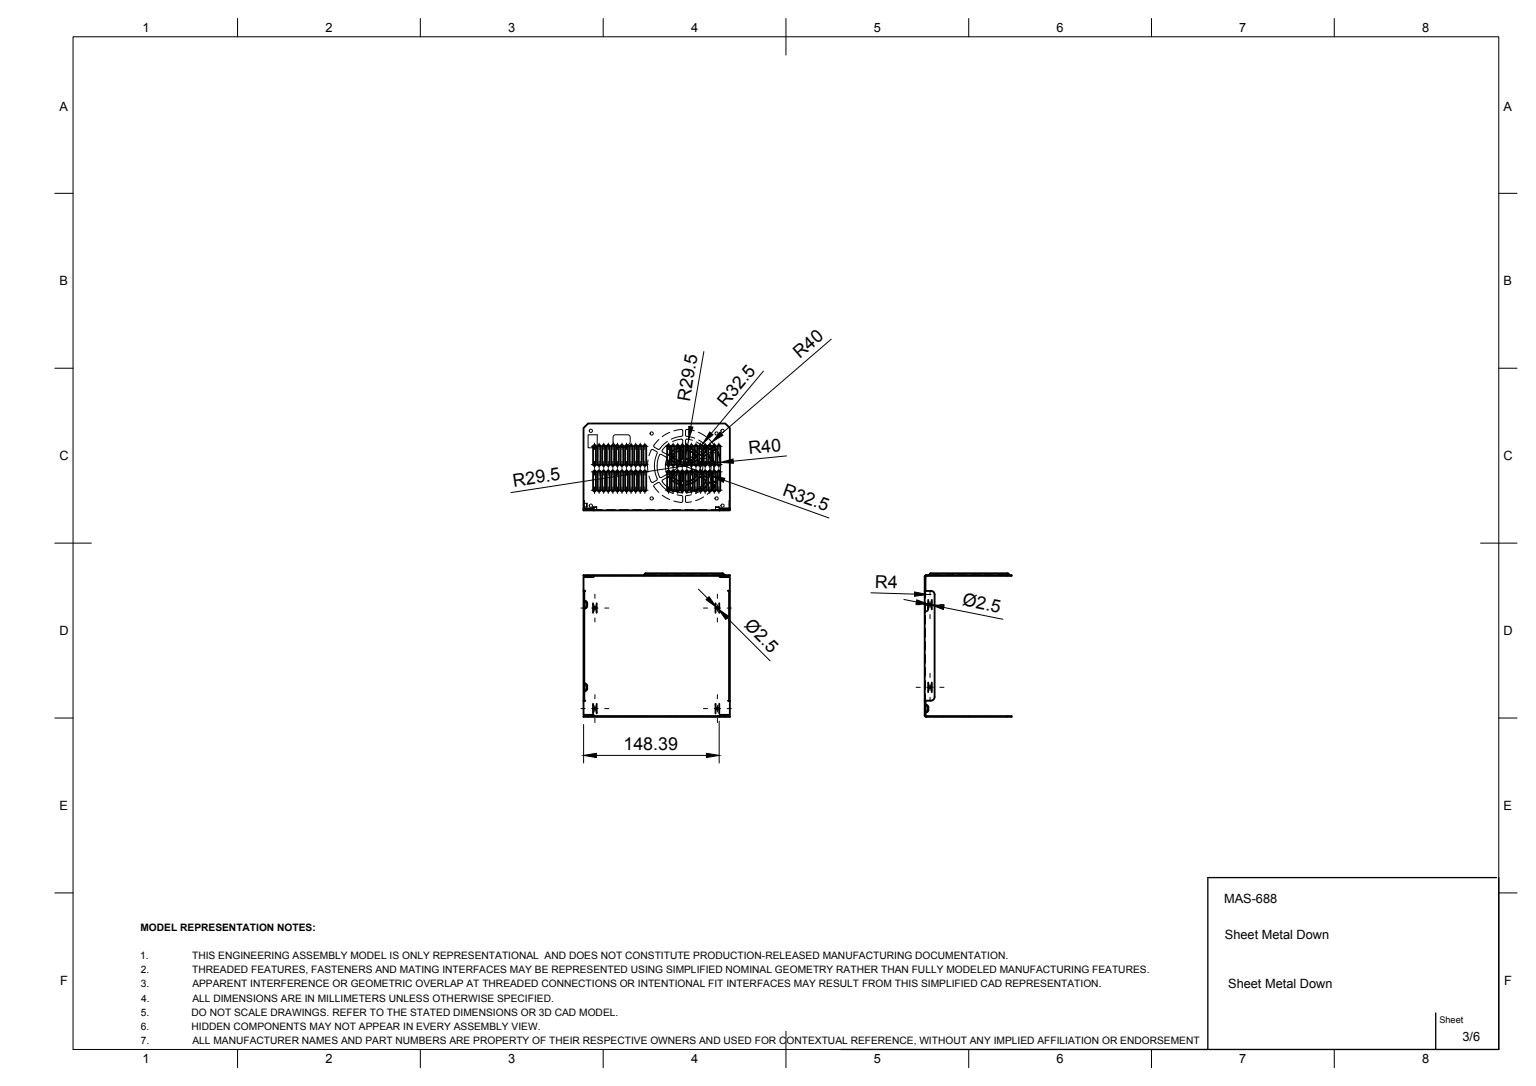
ISO-10303-21;
HEADER;
/* Generated by software containing ST-Developer
 * from STEP Tools, Inc. (www.steptools.com) 
 */

FILE_DESCRIPTION(
/* description */ ('STEP AP214'),
/* implementation_level */ '2;1');

FILE_NAME(
/* name */ 'Sheet Metal Down.step',
/* time_stamp */ '2026-11-14T03:58:36-08:00',
/* author */ (''),
/* organization */ (''),
/* preprocessor_version */ 'ST-DEVELOPER v20.2',
/* originating_system */ 'Autodesk Translation Framework v15.17.0.0',
/* authorisation */ '');

FILE_SCHEMA (('AUTOMOTIVE_DESIGN { 1 0 10303 214 3 1 1 }'));
ENDSEC;

DATA;
#10=MECHANICAL_DESIGN_GEOMETRIC_PRESENTATION_REPRESENTATION('',(#41),#65304);
#33=SHAPE_REPRESENTATION_RELATIONSHIP('SRR','None',#65324,#37);
#37=ADVANCED_BREP_SHAPE_REPRESENTATION('',(#45),#65300);
#41=STYLED_ITEM('',(#65353),#45);
#45=MANIFOLD_SOLID_BREP('Body1',#39933);
#48=FACE_BOUND('',#4336,.T.);
#49=FACE_BOUND('',#4337,.T.);
#50=FACE_BOUND('',#4338,.T.);
#51=FACE_BOUND('',#4339,.T.);
#52=FACE_BOUND('',#4341,.T.);
#53=FACE_BOUND('',#4342,.T.);
#54=FACE_BOUND('',#4343,.T.);
#55=FACE_BOUND('',#4344,.T.);
#56=FACE_BOUND('',#4348,.T.);
#57=FACE_BOUND('',#4349,.T.);
#58=FACE_BOUND('',#4351,.T.);
#59=FACE_BOUND('',#4352,.T.);
#60=FACE_BOUND('',#4356,.T.);
#61=FACE_BOUND('',#4357,.T.);
#62=FACE_BOUND('',#4358,.T.);
#63=FACE_BOUND('',#4359,.T.);
#64=FACE_BOUND('',#4360,.T.);
#65=FACE_BOUND('',#4361,.T.);
#66=FACE_BOUND('',#4362,.T.);
#67=FACE_BOUND('',#4363,.T.);
#68=FACE_BOUND('',#4364,.T.);
#69=FACE_BOUND('',#4365,.T.);
#70=FACE_BOUND('',#4366,.T.);
#71=FACE_BOUND('',#4367,.T.);
#72=FACE_BOUND('',#4368,.T.);
#73=FACE_BOUND('',#4369,.T.);
#74=FACE_BOUND('',#4370,.T.);
#75=FACE_BOUND('',#4371,.T.);
#76=FACE_BOUND('',#4372,.T.);
#77=FACE_BOUND('',#4373,.T.);
#78=FACE_BOUND('',#4374,.T.);
#79=FACE_BOUND('',#4375,.T.);
#80=FACE_BOUND('',#4376,.T.);
#81=FACE_BOUND('',#4377,.T.);
#82=FACE_BOUND('',#4378,.T.);
#83=FACE_BOUND('',#4379,.T.);
#84=FACE_BOUND('',#4380,.T.);
#85=FACE_BOUND('',#4381,.T.);
#86=FACE_BOUND('',#4382,.T.);
#87=FACE_BOUND('',#4383,.T.);
#88=FACE_BOUND('',#4384,.T.);
#89=FACE_BOUND('',#4385,.T.);
#90=FACE_BOUND('',#4386,.T.);
#91=FACE_BOUND('',#4387,.T.);
#92=FACE_BOUND('',#4388,.T.);
#93=FACE_BOUND('',#4389,.T.);
#94=FACE_BOUND('',#4390,.T.);
#95=FACE_BOUND('',#4391,.T.);
#96=FACE_BOUND('',#4392,.T.);
#97=FACE_BOUND('',#4393,.T.);
#98=FACE_BOUND('',#4394,.T.);
#99=FACE_BOUND('',#4395,.T.);
#100=FACE_BOUND('',#4396,.T.);
#101=FACE_BOUND('',#4397,.T.);
#102=FACE_BOUND('',#4398,.T.);
#103=FACE_BOUND('',#4399,.T.);
#104=FACE_BOUND('',#4400,.T.);
#105=FACE_BOUND('',#4401,.T.);
#106=FACE_BOUND('',#4402,.T.);
#107=FACE_BOUND('',#4403,.T.);
#108=FACE_BOUND('',#4405,.T.);
#109=FACE_BOUND('',#4406,.T.);
#110=FACE_BOUND('',#4407,.T.);
#111=FACE_BOUND('',#4408,.T.);
#112=FACE_BOUND('',#4409,.T.);
#113=FACE_BOUND('',#4410,.T.);
#114=FACE_BOUND('',#4411,.T.);
#115=FACE_BOUND('',#4412,.T.);
#116=FACE_BOUND('',#4413,.T.);
#117=FACE_BOUND('',#4414,.T.);
#118=FACE_BOUND('',#4415,.T.);
#119=FACE_BOUND('',#4416,.T.);
#120=FACE_BOUND('',#4417,.T.);
#121=FACE_BOUND('',#4418,.T.);
#122=FACE_BOUND('',#4419,.T.);
#123=FACE_BOUND('',#4420,.T.);
#124=FACE_BOUND('',#4421,.T.);
#125=FACE_BOUND('',#4422,.T.);
#126=FACE_BOUND('',#4423,.T.);
#127=FACE_BOUND('',#4424,.T.);
#128=FACE_BOUND('',#4425,.T.);
#129=FACE_BOUND('',#4426,.T.);
#130=FACE_BOUND('',#4427,.T.);
#131=FACE_BOUND('',#4428,.T.);
#132=FACE_BOUND('',#4429,.T.);
#133=FACE_BOUND('',#4430,.T.);
#134=FACE_BOUND('',#4431,.T.);
#135=FACE_BOUND('',#4432,.T.);
#136=FACE_BOUND('',#4433,.T.);
#137=FACE_BOUND('',#4434,.T.);
#138=FACE_BOUND('',#4435,.T.);
#139=FACE_BOUND('',#4436,.T.);
#140=FACE_BOUND('',#4437,.T.);
#141=FACE_BOUND('',#4438,.T.);
#142=FACE_BOUND('',#4439,.T.);
#143=FACE_BOUND('',#4440,.T.);
#144=FACE_BOUND('',#4441,.T.);
#145=FACE_BOUND('',#4442,.T.);
#146=FACE_BOUND('',#4443,.T.);
#147=FACE_BOUND('',#4444,.T.);
#148=FACE_BOUND('',#4445,.T.);
#149=FACE_BOUND('',#4446,.T.);
#150=FACE_BOUND('',#4447,.T.);
#151=FACE_BOUND('',#4448,.T.);
#152=FACE_BOUND('',#4449,.T.);
#153=FACE_BOUND('',#4450,.T.);
#154=FACE_BOUND('',#4451,.T.);
#155=FACE_BOUND('',#4452,.T.);
#156=FACE_BOUND('',#4479,.T.);
#157=FACE_BOUND('',#4480,.T.);
#158=FACE_BOUND('',#4481,.T.);
#159=FACE_BOUND('',#4482,.T.);
#160=FACE_BOUND('',#4483,.T.);
#161=FACE_BOUND('',#4484,.T.);
#162=FACE_BOUND('',#4485,.T.);
#163=FACE_BOUND('',#4486,.T.);
#164=FACE_BOUND('',#4487,.T.);
#165=FACE_BOUND('',#4488,.T.);
#166=FACE_BOUND('',#4489,.T.);
#167=FACE_BOUND('',#4490,.T.);
#168=FACE_BOUND('',#4491,.T.);
#169=FACE_BOUND('',#4492,.T.);
#170=FACE_BOUND('',#4493,.T.);
#171=FACE_BOUND('',#4494,.T.);
#172=FACE_BOUND('',#4495,.T.);
#173=FACE_BOUND('',#4496,.T.);
#174=FACE_BOUND('',#4503,.T.);
#175=FACE_BOUND('',#4504,.T.);
#176=FACE_BOUND('',#4505,.T.);
#177=FACE_BOUND('',#4506,.T.);
#178=FACE_BOUND('',#4507,.T.);
#179=FACE_BOUND('',#4508,.T.);
#180=FACE_BOUND('',#4509,.T.);
#181=FACE_BOUND('',#4510,.T.);
#182=FACE_BOUND('',#4511,.T.);
#183=FACE_BOUND('',#4512,.T.);
#184=FACE_BOUND('',#4513,.T.);
#185=FACE_BOUND('',#4515,.T.);
#186=FACE_BOUND('',#4516,.T.);
#187=FACE_BOUND('',#4517,.T.);
#188=FACE_BOUND('',#4518,.T.);
#189=FACE_BOUND('',#4519,.T.);
#190=FACE_BOUND('',#4520,.T.);
#191=FACE_BOUND('',#4521,.T.);
#192=FACE_BOUND('',#4522,.T.);
#193=FACE_BOUND('',#4523,.T.);
#194=FACE_BOUND('',#4524,.T.);
#195=FACE_BOUND('',#4525,.T.);
#196=FACE_BOUND('',#4567,.T.);
#197=FACE_BOUND('',#4575,.T.);
#198=FACE_BOUND('',#4587,.T.);
#199=FACE_BOUND('',#4595,.T.);
#200=FACE_BOUND('',#4607,.T.);
#201=FACE_BOUND('',#4615,.T.);
#202=FACE_BOUND('',#4627,.T.);
#203=FACE_BOUND('',#4635,.T.);
#204=FACE_BOUND('',#4637,.T.);
#205=FACE_BOUND('',#4638,.T.);
#206=FACE_BOUND('',#4639,.T.);
#207=FACE_BOUND('',#4640,.T.);
#208=FACE_BOUND('',#4641,.T.);
#209=FACE_BOUND('',#4642,.T.);
#210=FACE_BOUND('',#4643,.T.);
#211=FACE_BOUND('',#4644,.T.);
#212=FACE_BOUND('',#4645,.T.);
#213=FACE_BOUND('',#4646,.T.);
#214=FACE_BOUND('',#4647,.T.);
#215=FACE_BOUND('',#4648,.T.);
#216=FACE_BOUND('',#4649,.T.);
#217=FACE_BOUND('',#4650,.T.);
#218=FACE_BOUND('',#4651,.T.);
#219=FACE_BOUND('',#4652,.T.);
#220=FACE_BOUND('',#4653,.T.);
#221=FACE_BOUND('',#4654,.T.);
#222=FACE_BOUND('',#4941,.T.);
#223=FACE_BOUND('',#4949,.T.);
#224=FACE_BOUND('',#4961,.T.);
#225=FACE_BOUND('',#4969,.T.);
#629=PLANE('',#40239);
#630=PLANE('',#40244);
#631=PLANE('',#40249);
#632=PLANE('',#40250);
#633=PLANE('',#40251);
#634=PLANE('',#40254);
#635=PLANE('',#40257);
#636=PLANE('',#40258);
#637=PLANE('',#40259);
#638=PLANE('',#40310);
#639=PLANE('',#40361);
#640=PLANE('',#40362);
#641=PLANE('',#40363);
#642=PLANE('',#40364);
#643=PLANE('',#40365);
#644=PLANE('',#40366);
#645=PLANE('',#40367);
#646=PLANE('',#40368);
#647=PLANE('',#40369);
#648=PLANE('',#40370);
#649=PLANE('',#40371);
#650=PLANE('',#40372);
#651=PLANE('',#40373);
#652=PLANE('',#40374);
#653=PLANE('',#40375);
#654=PLANE('',#40376);
#655=PLANE('',#40377);
#656=PLANE('',#40378);
#657=PLANE('',#40379);
#658=PLANE('',#40380);
#659=PLANE('',#40381);
#660=PLANE('',#40382);
#661=PLANE('',#40383);
#662=PLANE('',#40384);
#663=PLANE('',#40385);
#664=PLANE('',#40440);
#665=PLANE('',#40441);
#666=PLANE('',#40450);
#667=PLANE('',#40460);
#668=PLANE('',#40462);
#669=PLANE('',#40464);
#670=PLANE('',#40466);
#671=PLANE('',#40469);
#672=PLANE('',#40470);
#673=PLANE('',#40471);
#674=PLANE('',#40472);
#675=PLANE('',#40473);
#676=PLANE('',#40478);
#677=PLANE('',#40479);
#678=PLANE('',#40480);
#679=PLANE('',#40481);
#680=PLANE('',#40482);
#681=PLANE('',#40485);
#682=PLANE('',#40488);
#683=PLANE('',#40497);
#684=PLANE('',#40504);
#685=PLANE('',#40513);
#686=PLANE('',#40514);
#687=PLANE('',#40515);
#688=PLANE('',#40520);
#689=PLANE('',#40521);
#690=PLANE('',#40522);
#691=PLANE('',#40523);
#692=PLANE('',#40526);
#693=PLANE('',#40535);
#694=PLANE('',#40542);
#695=PLANE('',#40551);
#696=PLANE('',#40552);
#697=PLANE('',#40553);
#698=PLANE('',#40558);
#699=PLANE('',#40559);
#700=PLANE('',#40560);
#701=PLANE('',#40561);
#702=PLANE('',#40564);
#703=PLANE('',#40573);
#704=PLANE('',#40580);
#705=PLANE('',#40589);
#706=PLANE('',#40590);
#707=PLANE('',#40591);
#708=PLANE('',#40596);
#709=PLANE('',#40597);
#710=PLANE('',#40598);
#711=PLANE('',#40599);
#712=PLANE('',#40602);
#713=PLANE('',#40611);
#714=PLANE('',#40618);
#715=PLANE('',#40627);
#716=PLANE('',#40628);
#717=PLANE('',#40629);
#718=PLANE('',#40634);
#719=PLANE('',#40635);
#720=PLANE('',#40636);
#721=PLANE('',#40637);
#722=PLANE('',#40692);
#723=PLANE('',#40693);
#724=PLANE('',#40694);
#725=PLANE('',#40695);
#726=PLANE('',#40696);
#727=PLANE('',#40697);
#728=PLANE('',#40698);
#729=PLANE('',#40699);
#730=PLANE('',#40700);
#731=PLANE('',#40701);
#732=PLANE('',#40702);
#733=PLANE('',#40758);
#734=PLANE('',#40760);
#735=PLANE('',#40762);
#736=PLANE('',#40764);
#737=PLANE('',#40766);
#738=PLANE('',#40768);
#739=PLANE('',#40769);
#740=PLANE('',#40770);
#741=PLANE('',#40771);
#742=PLANE('',#40772);
#743=PLANE('',#40773);
#744=PLANE('',#40774);
#745=PLANE('',#40775);
#746=PLANE('',#40776);
#747=PLANE('',#40777);
#748=PLANE('',#40779);
#749=PLANE('',#40780);
#750=PLANE('',#40781);
#751=PLANE('',#40783);
#752=PLANE('',#40784);
#753=PLANE('',#40786);
#754=PLANE('',#40788);
#755=PLANE('',#40789);
#756=PLANE('',#40790);
#757=PLANE('',#40792);
#758=PLANE('',#40794);
#759=PLANE('',#40795);
#760=PLANE('',#40797);
#761=PLANE('',#40798);
#762=PLANE('',#40799);
#763=PLANE('',#40801);
#764=PLANE('',#40802);
#765=PLANE('',#40804);
#766=PLANE('',#40805);
#767=PLANE('',#40807);
#768=PLANE('',#40808);
#769=PLANE('',#40810);
#770=PLANE('',#40812);
#771=PLANE('',#40813);
#772=PLANE('',#40815);
#773=PLANE('',#40816);
#774=PLANE('',#40818);
#775=PLANE('',#40819);
#776=PLANE('',#40821);
#777=PLANE('',#40822);
#778=PLANE('',#40824);
#779=PLANE('',#40825);
#780=PLANE('',#40827);
#781=PLANE('',#40828);
#782=PLANE('',#40830);
#783=PLANE('',#40831);
#784=PLANE('',#40832);
#785=PLANE('',#40834);
#786=PLANE('',#40835);
#787=PLANE('',#40837);
#788=PLANE('',#40838);
#789=PLANE('',#40840);
#790=PLANE('',#40841);
#791=PLANE('',#40843);
#792=PLANE('',#40844);
#793=PLANE('',#40846);
#794=PLANE('',#40848);
#795=PLANE('',#40849);
#796=PLANE('',#40851);
#797=PLANE('',#40852);
#798=PLANE('',#40854);
#799=PLANE('',#40855);
#800=PLANE('',#40857);
#801=PLANE('',#40858);
#802=PLANE('',#40860);
#803=PLANE('',#40861);
#804=PLANE('',#40863);
#805=PLANE('',#40864);
#806=PLANE('',#40866);
#807=PLANE('',#40867);
#808=PLANE('',#40869);
#809=PLANE('',#40870);
#810=PLANE('',#40872);
#811=PLANE('',#40873);
#812=PLANE('',#40875);
#813=PLANE('',#40876);
#814=PLANE('',#40878);
#815=PLANE('',#40879);
#816=PLANE('',#40881);
#817=PLANE('',#40882);
#818=PLANE('',#40884);
#819=PLANE('',#40885);
#820=PLANE('',#40887);
#821=PLANE('',#40888);
#822=PLANE('',#40890);
#823=PLANE('',#40891);
#824=PLANE('',#40893);
#825=PLANE('',#40894);
#826=PLANE('',#40896);
#827=PLANE('',#40897);
#828=PLANE('',#40899);
#829=PLANE('',#40900);
#830=PLANE('',#40902);
#831=PLANE('',#40903);
#832=PLANE('',#40905);
#833=PLANE('',#40906);
#834=PLANE('',#40908);
#835=PLANE('',#40909);
#836=PLANE('',#40911);
#837=PLANE('',#40912);
#838=PLANE('',#40914);
#839=PLANE('',#40915);
#840=PLANE('',#40917);
#841=PLANE('',#40918);
#842=PLANE('',#40920);
#843=PLANE('',#40921);
#844=PLANE('',#40922);
#845=PLANE('',#40923);
#846=PLANE('',#40924);
#847=PLANE('',#40925);
#848=PLANE('',#40926);
#849=PLANE('',#40927);
#850=PLANE('',#40930);
#851=PLANE('',#40935);
#852=PLANE('',#40936);
#853=PLANE('',#40938);
#854=PLANE('',#40940);
#855=PLANE('',#40943);
#856=PLANE('',#40952);
#857=PLANE('',#40959);
#858=PLANE('',#40968);
#859=PLANE('',#40969);
#860=PLANE('',#40970);
#861=PLANE('',#40975);
#862=PLANE('',#40976);
#863=PLANE('',#40977);
#864=PLANE('',#40978);
#865=PLANE('',#40981);
#866=PLANE('',#40990);
#867=PLANE('',#40997);
#868=PLANE('',#41006);
#869=PLANE('',#41007);
#870=PLANE('',#41008);
#871=PLANE('',#41013);
#872=PLANE('',#41014);
#873=PLANE('',#41015);
#874=PLANE('',#41016);
#875=PLANE('',#41017);
#876=PLANE('',#41018);
#877=PLANE('',#41019);
#878=PLANE('',#41020);
#879=PLANE('',#41021);
#880=PLANE('',#41022);
#881=PLANE('',#41025);
#882=PLANE('',#41030);
#883=PLANE('',#41031);
#884=PLANE('',#41032);
#885=PLANE('',#41035);
#886=PLANE('',#41039);
#2181=TOROIDAL_SURFACE('',#40213,42.,0.5);
#2182=TOROIDAL_SURFACE('',#40217,44.4494897427832,1.2);
#2183=TOROIDAL_SURFACE('',#40221,42.,1.3);
#2184=TOROIDAL_SURFACE('',#40224,44.4494897427832,2.);
#2193=B_SPLINE_CURVE_WITH_KNOTS('',3,(#53095,#53096,#53097,#53098,#53099,
#53100,#53101),.UNSPECIFIED.,.F.,.F.,(4,3,4),(0.,0.157051988846949,0.161817475839807),
 .UNSPECIFIED.);
#2194=B_SPLINE_CURVE_WITH_KNOTS('',3,(#53105,#53106,#53107,#53108,#53109,
#53110,#53111),.UNSPECIFIED.,.F.,.F.,(4,3,4),(-0.161817475844561,-0.157051988849942,
0.),.UNSPECIFIED.);
#2195=B_SPLINE_CURVE_WITH_KNOTS('',3,(#53125,#53126,#53127,#53128,#53129),
 .UNSPECIFIED.,.F.,.F.,(4,1,4),(0.,0.0312500000000001,0.0615627359467318),
 .UNSPECIFIED.);
#2196=B_SPLINE_CURVE_WITH_KNOTS('',3,(#53133,#53134,#53135,#53136,#53137),
 .UNSPECIFIED.,.F.,.F.,(4,1,4),(0.938437264048131,0.96875,1.),
 .UNSPECIFIED.);
#2197=B_SPLINE_CURVE_WITH_KNOTS('',3,(#53151,#53152,#53153,#53154,#53155),
 .UNSPECIFIED.,.F.,.F.,(4,1,4),(0.946686835703626,0.96875,1.),
 .UNSPECIFIED.);
#2198=B_SPLINE_CURVE_WITH_KNOTS('',3,(#53159,#53160,#53161,#53162,#53163),
 .UNSPECIFIED.,.F.,.F.,(4,1,4),(3.5013190022134E-10,0.0220631646607223,
0.0533131646607223),.UNSPECIFIED.);
#2199=B_SPLINE_CURVE_WITH_KNOTS('',3,(#53179,#53180,#53181,#53182,#53183,
#53184),.UNSPECIFIED.,.F.,.F.,(4,1,1,4),(0.,0.0312500000000001,0.0625000000000001,
0.0692715472300784),.UNSPECIFIED.);
#2200=B_SPLINE_CURVE_WITH_KNOTS('',3,(#53188,#53189,#53190,#53191,#53192,
#53193),.UNSPECIFIED.,.F.,.F.,(4,1,1,4),(0.930728452769685,0.9375,0.96875,
1.),.UNSPECIFIED.);
#2201=B_SPLINE_CURVE_WITH_KNOTS('',3,(#53209,#53210,#53211,#53212,#53213,
#53214),.UNSPECIFIED.,.F.,.F.,(4,1,1,4),(0.933751327236427,0.9375,0.96875,
1.),.UNSPECIFIED.);
#2202=B_SPLINE_CURVE_WITH_KNOTS('',3,(#53218,#53219,#53220,#53221,#53222,
#53223),.UNSPECIFIED.,.F.,.F.,(4,1,1,4),(0.,0.00374867276368319,0.0349986727636832,
0.0662486727636832),.UNSPECIFIED.);
#2203=B_SPLINE_CURVE_WITH_KNOTS('',3,(#53311,#53312,#53313,#53314,#53315,
#53316,#53317,#53318),.UNSPECIFIED.,.F.,.F.,(4,1,1,1,1,4),(-0.0709179217772133,
-0.0624999946725598,-0.0468738960837615,-0.0312499946726309,-0.0156244480037392,
3.22111226580546E-11),.UNSPECIFIED.);
#2204=B_SPLINE_CURVE_WITH_KNOTS('',3,(#53322,#53323,#53324,#53325,#53326,
#53327,#53328,#53329),.UNSPECIFIED.,.F.,.F.,(4,1,1,1,1,4),(-0.0709179217772133,
-0.0624999946725598,-0.0468738960837615,-0.0312499946726309,-0.0156244480037392,
3.22111226580546E-11),.UNSPECIFIED.);
#2205=B_SPLINE_CURVE_WITH_KNOTS('',3,(#54357,#54358,#54359,#54360,#54361,
#54362,#54363,#54364,#54365,#54366,#54367,#54368,#54369),.UNSPECIFIED.,
 .F.,.F.,(4,1,1,1,1,1,1,1,1,1,4),(0.762413302244216,0.765626103915763,0.781250005327804,
0.796876103916497,0.812500005327733,0.828126103916075,0.843750005327655,
0.859376103915845,0.875000005327586,0.890626103916147,0.904252904949607),
 .UNSPECIFIED.);
#2206=B_SPLINE_CURVE_WITH_KNOTS('',3,(#54373,#54374,#54375,#54376,#54377,
#54378,#54379,#54380,#54381,#54382,#54383,#54384,#54385),.UNSPECIFIED.,
 .F.,.F.,(4,1,1,1,1,1,1,1,1,1,4),(0.762413302244216,0.765626103915763,0.781250005327804,
0.796876103916497,0.812500005327733,0.828126103916075,0.843750005327655,
0.859376103915845,0.875000005327586,0.890626103916147,0.904252904949607),
 .UNSPECIFIED.);
#2207=B_SPLINE_CURVE_WITH_KNOTS('',3,(#54391,#54392,#54393,#54394,#54395),
 .UNSPECIFIED.,.F.,.F.,(4,1,4),(0.938437264053268,0.96875,1.),
 .UNSPECIFIED.);
#2208=B_SPLINE_CURVE_WITH_KNOTS('',3,(#54397,#54398,#54399,#54400,#54401,
#54402),.UNSPECIFIED.,.F.,.F.,(4,1,1,4),(0.,0.03125,0.0625,0.0662486727635731),
 .UNSPECIFIED.);
#2209=B_SPLINE_CURVE_WITH_KNOTS('',3,(#54409,#54410,#54411,#54412,#54413,
#54414,#54415),.UNSPECIFIED.,.F.,.F.,(4,3,4),(0.,0.00476894941081738,0.161935046139474),
 .UNSPECIFIED.);
#2210=B_SPLINE_CURVE_WITH_KNOTS('',3,(#54419,#54420,#54421,#54422,#54423),
 .UNSPECIFIED.,.F.,.F.,(4,1,4),(0.,0.0312500000000001,0.053313164296374),
 .UNSPECIFIED.);
#2211=B_SPLINE_CURVE_WITH_KNOTS('',3,(#54429,#54430,#54431,#54432,#54433,
#54434),.UNSPECIFIED.,.F.,.F.,(4,1,1,4),(0.801135800019621,0.8125,0.84375,
0.865533173173361),.UNSPECIFIED.);
#2212=B_SPLINE_CURVE_WITH_KNOTS('',3,(#54440,#54441,#54442,#54443,#54444,
#54445,#54446,#54447),.UNSPECIFIED.,.F.,.F.,(4,1,1,1,1,4),(0.780018892621858,
0.78125,0.8125,0.84375,0.875,0.886647915447513),.UNSPECIFIED.);
#2213=B_SPLINE_CURVE_WITH_KNOTS('',3,(#54452,#54453,#54454,#54455,#54456,
#54457),.UNSPECIFIED.,.F.,.F.,(4,1,1,4),(0.634466826826639,0.65625,0.6875,
0.698864199980379),.UNSPECIFIED.);
#2214=B_SPLINE_CURVE_WITH_KNOTS('',3,(#54465,#54466,#54467,#54468,#54469,
#54470,#54471,#54472),.UNSPECIFIED.,.F.,.F.,(4,1,1,1,1,4),(0.613352084552486,
0.625,0.65625,0.6875,0.71875,0.719981107378142),.UNSPECIFIED.);
#2215=B_SPLINE_CURVE_WITH_KNOTS('',3,(#54479,#54480,#54481,#54482,#54483,
#54484,#54485),.UNSPECIFIED.,.F.,.F.,(4,1,1,1,4),(0.467801769610686,0.46875,
0.5,0.53125,0.532198230389313),.UNSPECIFIED.);
#2216=B_SPLINE_CURVE_WITH_KNOTS('',3,(#54492,#54493,#54494,#54495,#54496,
#54497,#54498),.UNSPECIFIED.,.F.,.F.,(4,1,1,1,4),(0.446686835703626,0.46875,
0.5,0.53125,0.553313164296374),.UNSPECIFIED.);
#2217=B_SPLINE_CURVE_WITH_KNOTS('',3,(#54504,#54505,#54506,#54507,#54508,
#54509),.UNSPECIFIED.,.F.,.F.,(4,1,1,4),(0.301135800019622,0.3125,0.34375,
0.36553317317336),.UNSPECIFIED.);
#2218=B_SPLINE_CURVE_WITH_KNOTS('',3,(#54516,#54517,#54518,#54519,#54520,
#54521,#54522,#54523),.UNSPECIFIED.,.F.,.F.,(4,1,1,1,1,4),(0.280018892621858,
0.28125,0.3125,0.34375,0.375,0.386647915447513),.UNSPECIFIED.);
#2219=B_SPLINE_CURVE_WITH_KNOTS('',3,(#54530,#54531,#54532,#54533,#54534,
#54535),.UNSPECIFIED.,.F.,.F.,(4,1,1,4),(0.13446682682664,0.15625,0.1875,
0.198864199980378),.UNSPECIFIED.);
#2220=B_SPLINE_CURVE_WITH_KNOTS('',3,(#54540,#54541,#54542,#54543,#54544,
#54545,#54546,#54547),.UNSPECIFIED.,.F.,.F.,(4,1,1,1,1,4),(0.113352084552487,
0.125,0.15625,0.1875,0.21875,0.219981107378142),.UNSPECIFIED.);
#2221=B_SPLINE_CURVE_WITH_KNOTS('',3,(#54551,#54552,#54553,#54554,#54555,
#54556,#54557,#54558),.UNSPECIFIED.,.F.,.F.,(4,1,1,1,1,4),(0.771771373885868,
0.78125,0.8125,0.84375,0.875,0.894896231061431),.UNSPECIFIED.);
#2222=B_SPLINE_CURVE_WITH_KNOTS('',3,(#54562,#54563,#54564,#54565,#54566,
#54567,#54568,#54569),.UNSPECIFIED.,.F.,.F.,(4,1,1,1,1,4),(0.767085043602908,
0.78125,0.8125,0.84375,0.875,0.899580964190556),.UNSPECIFIED.);
#2223=B_SPLINE_CURVE_WITH_KNOTS('',3,(#54572,#54573,#54574,#54575,#54576,
#54577,#54578,#54579),.UNSPECIFIED.,.F.,.F.,(4,1,1,1,1,4),(0.605103768938569,
0.625,0.65625,0.6875,0.71875,0.728228626114132),.UNSPECIFIED.);
#2224=B_SPLINE_CURVE_WITH_KNOTS('',3,(#54584,#54585,#54586,#54587,#54588,
#54589,#54590,#54591),.UNSPECIFIED.,.F.,.F.,(4,1,1,1,1,4),(0.600419035809444,
0.625,0.65625,0.6875,0.71875,0.732914956397092),.UNSPECIFIED.);
#2225=B_SPLINE_CURVE_WITH_KNOTS('',3,(#54596,#54597,#54598,#54599,#54600,
#54601,#54602),.UNSPECIFIED.,.F.,.F.,(4,1,1,1,4),(0.438437264053268,0.46875,
0.5,0.53125,0.561562735946732),.UNSPECIFIED.);
#2226=B_SPLINE_CURVE_WITH_KNOTS('',3,(#54606,#54607,#54608,#54609,#54610,
#54611,#54612,#54613,#54614),.UNSPECIFIED.,.F.,.F.,(4,1,1,1,1,1,4),(0.433751327236426,
0.4375,0.46875,0.5,0.53125,0.5625,0.566248672763573),.UNSPECIFIED.);
#2227=B_SPLINE_CURVE_WITH_KNOTS('',3,(#54618,#54619,#54620,#54621,#54622,
#54623,#54624,#54625),.UNSPECIFIED.,.F.,.F.,(4,1,1,1,1,4),(0.271771373885868,
0.28125,0.3125,0.34375,0.375,0.394896231061431),.UNSPECIFIED.);
#2228=B_SPLINE_CURVE_WITH_KNOTS('',3,(#54629,#54630,#54631,#54632,#54633,
#54634,#54635,#54636),.UNSPECIFIED.,.F.,.F.,(4,1,1,1,1,4),(0.267085043602908,
0.28125,0.3125,0.34375,0.375,0.399580964190556),.UNSPECIFIED.);
#2229=B_SPLINE_CURVE_WITH_KNOTS('',3,(#54640,#54641,#54642,#54643,#54644,
#54645,#54646,#54647),.UNSPECIFIED.,.F.,.F.,(4,1,1,1,1,4),(0.105103768938569,
0.125,0.15625,0.1875,0.21875,0.228228626114132),.UNSPECIFIED.);
#2230=B_SPLINE_CURVE_WITH_KNOTS('',3,(#54650,#54651,#54652,#54653,#54654,
#54655,#54656,#54657),.UNSPECIFIED.,.F.,.F.,(4,1,1,1,1,4),(0.100419035809444,
0.125,0.15625,0.1875,0.21875,0.232914956397092),.UNSPECIFIED.);
#2231=B_SPLINE_CURVE_WITH_KNOTS('',3,(#54661,#54662,#54663,#54664,#54665,
#54666,#54667,#54668),.UNSPECIFIED.,.F.,.F.,(4,1,1,1,1,4),(0.764061321213706,
0.78125,0.8125,0.84375,0.875,0.902605614421776),.UNSPECIFIED.);
#2232=B_SPLINE_CURVE_WITH_KNOTS('',3,(#54672,#54673,#54674,#54675,#54676,
#54677,#54678,#54679),.UNSPECIFIED.,.F.,.F.,(4,1,1,1,1,4),(0.597394385578223,
0.625,0.65625,0.6875,0.71875,0.735938678786293),.UNSPECIFIED.);
#2233=B_SPLINE_CURVE_WITH_KNOTS('',3,(#54684,#54685,#54686,#54687,#54688,
#54689,#54690,#54691,#54692,#54693,#54694,#54695,#54696),.UNSPECIFIED.,
 .F.,.F.,(4,1,1,1,1,1,1,1,1,1,4),(0.595747106058032,0.609376103916341,0.625000005328168,
0.640626103916569,0.656250005328095,0.671876103916693,0.687500005328024,
0.703126103916646,0.718750005327949,0.734376103915816,0.737586706461852),
 .UNSPECIFIED.);
#2234=B_SPLINE_CURVE_WITH_KNOTS('',3,(#54701,#54702,#54703,#54704,#54705,
#54706,#54707,#54708,#54709),.UNSPECIFIED.,.F.,.F.,(4,1,1,1,1,1,4),(0.430728452769921,
0.4375,0.46875,0.5,0.53125,0.5625,0.569271547230078),.UNSPECIFIED.);
#2235=B_SPLINE_CURVE_WITH_KNOTS('',3,(#54713,#54714,#54715,#54716,#54717,
#54718,#54719,#54720,#54721,#54722,#54723,#54724,#54725),.UNSPECIFIED.,
 .F.,.F.,(4,1,1,1,1,1,1,1,1,1,4),(0.429082078647101,0.437500005328602,0.453126103916167,
0.468750005328528,0.484376103916409,0.500000005328459,0.515626103916853,
0.531250005328387,0.546876103916685,0.562500005328313,0.57091793098853),
 .UNSPECIFIED.);
#2236=B_SPLINE_CURVE_WITH_KNOTS('',3,(#54729,#54730,#54731,#54732,#54733,
#54734,#54735,#54736),.UNSPECIFIED.,.F.,.F.,(4,1,1,1,1,4),(0.264061321213707,
0.28125,0.3125,0.34375,0.375,0.402605614421775),.UNSPECIFIED.);
#2237=B_SPLINE_CURVE_WITH_KNOTS('',3,(#54740,#54741,#54742,#54743,#54744,
#54745,#54746,#54747,#54748,#54749,#54750,#54751,#54752),.UNSPECIFIED.,
 .F.,.F.,(4,1,1,1,1,1,1,1,1,1,4),(0.262413302245398,0.265626103917436,0.28125000532897,
0.296876103917406,0.312500005328897,0.328126103917406,0.343750005328825,
0.359376103917345,0.375000005328751,0.390626103917082,0.404252904915522),
 .UNSPECIFIED.);
#2238=B_SPLINE_CURVE_WITH_KNOTS('',3,(#54756,#54757,#54758,#54759,#54760,
#54761,#54762,#54763),.UNSPECIFIED.,.F.,.F.,(4,1,1,1,1,4),(0.097394385578224,
0.125,0.15625,0.1875,0.21875,0.235938678786293),.UNSPECIFIED.);
#2239=B_SPLINE_CURVE_WITH_KNOTS('',3,(#54766,#54767,#54768,#54769,#54770,
#54771,#54772,#54773,#54774,#54775,#54776,#54777,#54778),.UNSPECIFIED.,
 .F.,.F.,(4,1,1,1,1,1,1,1,1,1,4),(0.0957471060944922,0.109376103917698,
0.125000005329334,0.140626103917786,0.156250005329262,0.171876103917926,
0.18750000532919,0.203126103917764,0.218750005329116,0.234376103917514,
0.237586706463033),.UNSPECIFIED.);
#2240=B_SPLINE_CURVE_WITH_KNOTS('',3,(#54783,#54784,#54785,#54786,#54787,
#54788),.UNSPECIFIED.,.F.,.F.,(4,1,1,4),(0.930728452769921,0.9375,0.96875,
1.),.UNSPECIFIED.);
#2241=B_SPLINE_CURVE_WITH_KNOTS('',3,(#54790,#54791,#54792,#54793,#54794,
#54795,#54796,#54797),.UNSPECIFIED.,.F.,.F.,(4,1,1,1,1,4),(0.,0.0156255519209496,
0.0312500053295531,0.0468761039179887,0.0625000053294804,0.0709179305664047),
 .UNSPECIFIED.);
#2242=B_SPLINE_CURVE_WITH_KNOTS('',3,(#54814,#54815,#54816,#54817,#54818,
#54819,#54820,#54821),.UNSPECIFIED.,.F.,.F.,(4,1,1,1,1,4),(0.,0.0156255519209496,
0.0312500053295531,0.0468761039179887,0.0625000053294804,0.0709179305664047),
 .UNSPECIFIED.);
#2243=B_SPLINE_CURVE_WITH_KNOTS('',3,(#54853,#54854,#54855,#54856,#54857,
#54858,#54859,#54860,#54861,#54862,#54863,#54864,#54865),.UNSPECIFIED.,
 .F.,.F.,(4,1,1,1,1,1,1,1,1,1,4),(0.0957471060944922,0.109376103917698,
0.125000005329334,0.140626103917786,0.156250005329262,0.171876103917926,
0.18750000532919,0.203126103917764,0.218750005329116,0.234376103917514,
0.237586706463033),.UNSPECIFIED.);
#2244=B_SPLINE_CURVE_WITH_KNOTS('',3,(#54895,#54896,#54897,#54898,#54899,
#54900,#54901,#54902,#54903,#54904,#54905,#54906,#54907),.UNSPECIFIED.,
 .F.,.F.,(4,1,1,1,1,1,1,1,1,1,4),(0.262413302245398,0.265626103917436,0.28125000532897,
0.296876103917406,0.312500005328897,0.328126103917406,0.343750005328825,
0.359376103917345,0.375000005328751,0.390626103917082,0.404252904915522),
 .UNSPECIFIED.);
#2245=B_SPLINE_CURVE_WITH_KNOTS('',3,(#54936,#54937,#54938,#54939,#54940,
#54941,#54942,#54943,#54944,#54945,#54946,#54947,#54948),.UNSPECIFIED.,
 .F.,.F.,(4,1,1,1,1,1,1,1,1,1,4),(0.429082078647101,0.437500005328602,0.453126103916167,
0.468750005328528,0.484376103916409,0.500000005328459,0.515626103916853,
0.531250005328387,0.546876103916685,0.562500005328313,0.57091793098853),
 .UNSPECIFIED.);
#2246=B_SPLINE_CURVE_WITH_KNOTS('',3,(#55119,#55120,#55121,#55122,#55123,
#55124,#55125,#55126,#55127,#55128,#55129,#55130,#55131,#55132,#55133,#55134,
#55135,#55136,#55137,#55138),.UNSPECIFIED.,.F.,.F.,(4,2,2,2,2,2,2,2,2,4),
(0.,0.25,0.375,0.4375,0.46875,0.484375,0.4921875,0.5,0.75,1.),
 .UNSPECIFIED.);
#2247=B_SPLINE_CURVE_WITH_KNOTS('',3,(#55142,#55143,#55144,#55145,#55146,
#55147,#55148,#55149,#55150,#55151,#55152,#55153,#55154,#55155,#55156,#55157,
#55158,#55159,#55160,#55161,#55162,#55163,#55164,#55165,#55166,#55167,#55168,
#55169,#55170,#55171,#55172,#55173,#55174,#55175,#55176,#55177,#55178,#55179,
#55180,#55181,#55182,#55183,#55184),.UNSPECIFIED.,.F.,.F.,(4,3,3,3,3,3,
3,3,3,3,3,3,3,3,4),(0.,0.0927561114044612,0.190932288541826,0.249999999999901,
0.374999999999842,0.437499999999813,0.468749992147447,0.484374999999801,
0.492187499999797,0.499999999999798,0.749999999999899,0.83185850735952,
0.909993813469674,0.982561474349579,1.),.UNSPECIFIED.);
#2248=B_SPLINE_CURVE_WITH_KNOTS('',3,(#55228,#55229,#55230,#55231,#55232,
#55233,#55234,#55235,#55236,#55237,#55238,#55239,#55240,#55241,#55242,#55243,
#55244,#55245,#55246,#55247),.UNSPECIFIED.,.F.,.F.,(4,2,2,2,2,2,2,2,2,4),
(0.,0.25,0.375,0.4375,0.46875,0.484375,0.4921875,0.5,0.75,1.),
 .UNSPECIFIED.);
#2249=B_SPLINE_CURVE_WITH_KNOTS('',3,(#55248,#55249,#55250,#55251,#55252,
#55253,#55254,#55255,#55256,#55257,#55258,#55259,#55260,#55261,#55262,#55263,
#55264,#55265,#55266,#55267,#55268,#55269,#55270,#55271,#55272,#55273,#55274,
#55275,#55276,#55277,#55278,#55279,#55280,#55281,#55282,#55283,#55284,#55285,
#55286,#55287,#55288,#55289,#55290),.UNSPECIFIED.,.F.,.F.,(4,3,3,3,3,3,
3,3,3,3,3,3,3,3,4),(0.,0.0927561113839666,0.190932288501874,0.2499999999999,
0.374999999999847,0.437499999999822,0.468749992147457,0.48437499999981,
0.492187499999816,0.49999999999981,0.749999999999905,0.83185850736903,0.909993813488733,
0.982561474378202,1.),.UNSPECIFIED.);
#2250=B_SPLINE_CURVE_WITH_KNOTS('',3,(#55351,#55352,#55353,#55354,#55355,
#55356,#55357,#55358,#55359,#55360,#55361,#55362,#55363,#55364,#55365,#55366,
#55367,#55368,#55369,#55370),.UNSPECIFIED.,.F.,.F.,(4,2,2,2,2,2,2,2,2,4),
(0.,0.25,0.375,0.4375,0.46875,0.484375,0.4921875,0.5,0.75,1.),
 .UNSPECIFIED.);
#2251=B_SPLINE_CURVE_WITH_KNOTS('',3,(#55371,#55372,#55373,#55374,#55375,
#55376,#55377,#55378,#55379,#55380,#55381,#55382,#55383,#55384,#55385,#55386,
#55387,#55388,#55389,#55390,#55391,#55392,#55393,#55394,#55395,#55396,#55397,
#55398,#55399,#55400,#55401,#55402,#55403,#55404,#55405,#55406,#55407,#55408,
#55409,#55410,#55411,#55412,#55413),.UNSPECIFIED.,.F.,.F.,(4,3,3,3,3,3,
3,3,3,3,3,3,3,3,4),(0.,0.0927561113855575,0.190932288505144,0.250000000000093,
0.37500000000014,0.437500000000168,0.468749992147812,0.48437500000018,0.492187500000186,
0.500000000000184,0.750000000000092,0.831858507368402,0.909993813487336,
0.982561474376173,1.),.UNSPECIFIED.);
#2252=B_SPLINE_CURVE_WITH_KNOTS('',3,(#55454,#55455,#55456,#55457,#55458,
#55459,#55460,#55461,#55462,#55463,#55464,#55465,#55466,#55467,#55468,#55469,
#55470,#55471,#55472,#55473),.UNSPECIFIED.,.F.,.F.,(4,2,2,2,2,2,2,2,2,4),
(0.,0.25,0.375,0.4375,0.46875,0.484375,0.4921875,0.5,0.75,1.),
 .UNSPECIFIED.);
#2253=B_SPLINE_CURVE_WITH_KNOTS('',3,(#55477,#55478,#55479,#55480,#55481,
#55482,#55483,#55484,#55485,#55486,#55487,#55488,#55489,#55490,#55491,#55492,
#55493,#55494,#55495,#55496,#55497,#55498,#55499,#55500,#55501,#55502,#55503,
#55504,#55505,#55506,#55507,#55508,#55509,#55510,#55511,#55512,#55513,#55514,
#55515,#55516,#55517,#55518,#55519),.UNSPECIFIED.,.F.,.F.,(4,3,3,3,3,3,
3,3,3,3,3,3,3,3,4),(0.,0.092756111383829,0.190932288501491,0.249999999999982,
0.374999999999972,0.437499999999958,0.468749992147606,0.484374999999957,
0.492187499999956,0.499999999999956,0.749999999999978,0.831858507368429,
0.909993813487417,0.982561474376421,1.),.UNSPECIFIED.);
#2254=B_SPLINE_CURVE_WITH_KNOTS('',3,(#55882,#55883,#55884,#55885,#55886),
 .UNSPECIFIED.,.F.,.F.,(4,1,4),(0.,0.0312500000000001,0.0533131643109959),
 .UNSPECIFIED.);
#2255=B_SPLINE_CURVE_WITH_KNOTS('',3,(#55889,#55890,#55891,#55892,#55893,
#55894,#55895),.UNSPECIFIED.,.F.,.F.,(4,3,4),(-0.161935046144155,-0.00476894941103452,
0.),.UNSPECIFIED.);
#2256=B_SPLINE_CURVE_WITH_KNOTS('',3,(#55903,#55904,#55905,#55906,#55907,
#55908,#55909,#55910),.UNSPECIFIED.,.F.,.F.,(4,1,1,1,1,4),(0.,0.00123110737814575,
0.0324811073781457,0.0637311073781457,0.0949811073781457,0.106629022825536),
 .UNSPECIFIED.);
#2257=B_SPLINE_CURVE_WITH_KNOTS('',3,(#55915,#55916,#55917,#55918,#55919,
#55920),.UNSPECIFIED.,.F.,.F.,(4,1,1,4),(0.134466826826819,0.15625,0.1875,
0.198864199679252),.UNSPECIFIED.);
#2258=B_SPLINE_CURVE_WITH_KNOTS('',3,(#55928,#55929,#55930,#55931,#55932,
#55933,#55934,#55935),.UNSPECIFIED.,.F.,.F.,(4,1,1,1,1,4),(0.,0.0116479154473907,
0.0428979154473907,0.0741479154473907,0.105397915447391,0.106629022825536),
 .UNSPECIFIED.);
#2259=B_SPLINE_CURVE_WITH_KNOTS('',3,(#55942,#55943,#55944,#55945,#55946,
#55947),.UNSPECIFIED.,.F.,.F.,(4,1,1,4),(0.301135800390954,0.3125,0.34375,
0.365533173173181),.UNSPECIFIED.);
#2260=B_SPLINE_CURVE_WITH_KNOTS('',3,(#55952,#55953,#55954,#55955,#55956,
#55957,#55958),.UNSPECIFIED.,.F.,.F.,(4,1,1,1,4),(0.,0.0220631642961554,
0.0533131642961553,0.0845631642961553,0.10662632859231),.UNSPECIFIED.);
#2261=B_SPLINE_CURVE_WITH_KNOTS('',3,(#55966,#55967,#55968,#55969,#55970,
#55971,#55972),.UNSPECIFIED.,.F.,.F.,(4,1,1,1,4),(0.467801769610687,0.46875,
0.5,0.53125,0.532198230389314),.UNSPECIFIED.);
#2262=B_SPLINE_CURVE_WITH_KNOTS('',3,(#55977,#55978,#55979,#55980,#55981,
#55982,#55983,#55984),.UNSPECIFIED.,.F.,.F.,(4,1,1,1,1,4),(0.,0.00123110737814613,
0.0324811073781462,0.063731107378146,0.0949811073781461,0.106629022825536),
 .UNSPECIFIED.);
#2263=B_SPLINE_CURVE_WITH_KNOTS('',3,(#55992,#55993,#55994,#55995,#55996,
#55997),.UNSPECIFIED.,.F.,.F.,(4,1,1,4),(0.63446682682682,0.65625,0.6875,
0.698864199679252),.UNSPECIFIED.);
#2264=B_SPLINE_CURVE_WITH_KNOTS('',3,(#56002,#56003,#56004,#56005,#56006,
#56007,#56008,#56009),.UNSPECIFIED.,.F.,.F.,(4,1,1,1,1,4),(0.,0.0116479154473909,
0.0428979154473909,0.0741479154473906,0.105397915447391,0.106629022825536),
 .UNSPECIFIED.);
#2265=B_SPLINE_CURVE_WITH_KNOTS('',3,(#56015,#56016,#56017,#56018,#56019,
#56020),.UNSPECIFIED.,.F.,.F.,(4,1,1,4),(0.801135800390954,0.8125,0.84375,
0.86553317317318),.UNSPECIFIED.);
#2266=B_SPLINE_CURVE_WITH_KNOTS('',3,(#56026,#56027,#56028,#56029,#56030,
#56031),.UNSPECIFIED.,.F.,.F.,(4,1,1,4),(0.,0.03125,0.0625,0.0662486727636835),
 .UNSPECIFIED.);
#2267=B_SPLINE_CURVE_WITH_KNOTS('',3,(#56034,#56035,#56036,#56037,#56038),
 .UNSPECIFIED.,.F.,.F.,(4,1,4),(0.,0.03125,0.0615627359472197),
 .UNSPECIFIED.);
#2268=B_SPLINE_CURVE_WITH_KNOTS('',3,(#56043,#56044,#56045,#56046,#56047,
#56048,#56049,#56050),.UNSPECIFIED.,.F.,.F.,(4,1,1,1,1,4),(0.,0.0141649563968439,
0.0454149563968439,0.0766649563968438,0.107914956396844,0.132495920587091),
 .UNSPECIFIED.);
#2269=B_SPLINE_CURVE_WITH_KNOTS('',3,(#56053,#56054,#56055,#56056,#56057,
#56058,#56059,#56060),.UNSPECIFIED.,.F.,.F.,(4,1,1,1,1,4),(0.105103768938473,
0.125,0.15625,0.1875,0.21875,0.228228626114295),.UNSPECIFIED.);
#2270=B_SPLINE_CURVE_WITH_KNOTS('',3,(#56065,#56066,#56067,#56068,#56069,
#56070,#56071,#56072),.UNSPECIFIED.,.F.,.F.,(4,1,1,1,1,4),(0.,0.0245809641902474,
0.0558309641902474,0.0870809641902473,0.118330964190247,0.132495920587091),
 .UNSPECIFIED.);
#2271=B_SPLINE_CURVE_WITH_KNOTS('',3,(#56076,#56077,#56078,#56079,#56080,
#56081,#56082,#56083),.UNSPECIFIED.,.F.,.F.,(4,1,1,1,1,4),(0.271771373885705,
0.28125,0.3125,0.34375,0.375,0.394896231061528),.UNSPECIFIED.);
#2272=B_SPLINE_CURVE_WITH_KNOTS('',3,(#56086,#56087,#56088,#56089,#56090,
#56091,#56092,#56093,#56094),.UNSPECIFIED.,.F.,.F.,(4,1,1,1,1,1,4),(0.,
0.00374867276368307,0.034998672763683,0.0662486727636831,0.0974986727636831,
0.128748672763683,0.132497345527366),.UNSPECIFIED.);
#2273=B_SPLINE_CURVE_WITH_KNOTS('',3,(#56099,#56100,#56101,#56102,#56103,
#56104,#56105),.UNSPECIFIED.,.F.,.F.,(4,1,1,1,4),(0.43843726405327,0.46875,
0.5,0.53125,0.561562735946731),.UNSPECIFIED.);
#2274=B_SPLINE_CURVE_WITH_KNOTS('',3,(#56108,#56109,#56110,#56111,#56112,
#56113,#56114,#56115),.UNSPECIFIED.,.F.,.F.,(4,1,1,1,1,4),(0.,0.0141649563968442,
0.0454149563968442,0.0766649563968441,0.107914956396844,0.132495920587091),
 .UNSPECIFIED.);
#2275=B_SPLINE_CURVE_WITH_KNOTS('',3,(#56120,#56121,#56122,#56123,#56124,
#56125,#56126,#56127),.UNSPECIFIED.,.F.,.F.,(4,1,1,1,1,4),(0.605103768938473,
0.625,0.65625,0.6875,0.71875,0.728228626114296),.UNSPECIFIED.);
#2276=B_SPLINE_CURVE_WITH_KNOTS('',3,(#56130,#56131,#56132,#56133,#56134,
#56135,#56136,#56137),.UNSPECIFIED.,.F.,.F.,(4,1,1,1,1,4),(0.,0.0245809641902476,
0.0558309641902476,0.0870809641902475,0.118330964190247,0.132495920587092),
 .UNSPECIFIED.);
#2277=B_SPLINE_CURVE_WITH_KNOTS('',3,(#56141,#56142,#56143,#56144,#56145,
#56146,#56147,#56148),.UNSPECIFIED.,.F.,.F.,(4,1,1,1,1,4),(0.771771373885705,
0.78125,0.8125,0.84375,0.875,0.894896231061527),.UNSPECIFIED.);
#2278=B_SPLINE_CURVE_WITH_KNOTS('',3,(#56153,#56154,#56155,#56156,#56157,
#56158),.UNSPECIFIED.,.F.,.F.,(4,1,1,4),(0.,0.03125,0.0625,0.0692715472303151),
 .UNSPECIFIED.);
#2279=B_SPLINE_CURVE_WITH_KNOTS('',3,(#56163,#56164,#56165,#56166,#56167,
#56168,#56169,#56170),.UNSPECIFIED.,.F.,.F.,(4,1,1,1,1,4),(0.0973943855783285,
0.125,0.15625,0.1875,0.21875,0.235938678786541),.UNSPECIFIED.);
#2280=B_SPLINE_CURVE_WITH_KNOTS('',3,(#56175,#56176,#56177,#56178,#56179,
#56180,#56181,#56182,#56183,#56184,#56185,#56186,#56187),.UNSPECIFIED.,
 .F.,.F.,(4,1,1,1,1,1,1,1,1,1,4),(0.595747106058032,0.609376103916341,0.625000005328168,
0.640626103916569,0.656250005328095,0.671876103916693,0.687500005328024,
0.703126103916646,0.718750005327949,0.734376103915816,0.737586706461852),
 .UNSPECIFIED.);
#2281=B_SPLINE_CURVE_WITH_KNOTS('',3,(#56191,#56192,#56193,#56194,#56195,
#56196,#56197,#56198),.UNSPECIFIED.,.F.,.F.,(4,1,1,1,1,4),(0.26406132121346,
0.28125,0.3125,0.34375,0.375,0.402605614421673),.UNSPECIFIED.);
#2282=B_SPLINE_CURVE_WITH_KNOTS('',3,(#56204,#56205,#56206,#56207,#56208,
#56209,#56210,#56211,#56212),.UNSPECIFIED.,.F.,.F.,(4,1,1,1,1,1,4),(0.430728452769685,
0.4375,0.46875,0.5,0.53125,0.5625,0.569271547230316),.UNSPECIFIED.);
#2283=B_SPLINE_CURVE_WITH_KNOTS('',3,(#56218,#56219,#56220,#56221,#56222,
#56223,#56224,#56225),.UNSPECIFIED.,.F.,.F.,(4,1,1,1,1,4),(0.597394385578329,
0.625,0.65625,0.6875,0.71875,0.735938678786541),.UNSPECIFIED.);
#2284=B_SPLINE_CURVE_WITH_KNOTS('',3,(#56230,#56231,#56232,#56233,#56234,
#56235,#56236,#56237),.UNSPECIFIED.,.F.,.F.,(4,1,1,1,1,4),(0.76406132121346,
0.78125,0.8125,0.84375,0.875,0.902605614421672),.UNSPECIFIED.);
#2285=B_SPLINE_SURFACE_WITH_KNOTS('',3,1,((#53083,#53084),(#53085,#53086),
(#53087,#53088),(#53089,#53090),(#53091,#53092)),.UNSPECIFIED.,.F.,.F.,
 .F.,(4,1,4),(2,2),(0.967801769610354,0.96875,1.),(0.,0.0959999999999937),
 .UNSPECIFIED.);
#2286=B_SPLINE_SURFACE_WITH_KNOTS('',3,1,((#53113,#53114),(#53115,#53116),
(#53117,#53118),(#53119,#53120),(#53121,#53122)),.UNSPECIFIED.,.F.,.F.,
 .F.,(4,1,4),(2,2),(0.938437264048131,0.96875,1.),(0.,0.0959999999999979),
 .UNSPECIFIED.);
#2287=B_SPLINE_SURFACE_WITH_KNOTS('',3,1,((#53139,#53140),(#53141,#53142),
(#53143,#53144),(#53145,#53146),(#53147,#53148)),.UNSPECIFIED.,.F.,.F.,
 .F.,(4,1,4),(2,2),(0.,0.0220631646607223,0.0533131646607223),(0.,0.0960000000000576),
 .UNSPECIFIED.);
#2288=B_SPLINE_SURFACE_WITH_KNOTS('',3,1,((#53165,#53166),(#53167,#53168),
(#53169,#53170),(#53171,#53172),(#53173,#53174),(#53175,#53176)),
 .UNSPECIFIED.,.F.,.F.,.F.,(4,1,1,4),(2,2),(0.930728452769685,0.9375,0.96875,
1.),(0.,0.0960000000000171),.UNSPECIFIED.);
#2289=B_SPLINE_SURFACE_WITH_KNOTS('',3,1,((#53195,#53196),(#53197,#53198),
(#53199,#53200),(#53201,#53202),(#53203,#53204),(#53205,#53206)),
 .UNSPECIFIED.,.F.,.F.,.F.,(4,1,1,4),(2,2),(0.,0.00374867276368319,0.0349986727636832,
0.0662486727636832),(0.,0.0960000000000512),.UNSPECIFIED.);
#2290=B_SPLINE_SURFACE_WITH_KNOTS('',3,1,((#53293,#53294),(#53295,#53296),
(#53297,#53298),(#53299,#53300),(#53301,#53302),(#53303,#53304),(#53305,
#53306),(#53307,#53308)),.UNSPECIFIED.,.F.,.F.,.F.,(4,1,1,1,1,4),(2,2),
(-3.22111226580546E-11,0.0156244480037392,0.0312499946726309,0.0468738960837615,
0.0624999946725598,0.0709179217772133),(0.,0.0960000000000491),
 .UNSPECIFIED.);
#2291=B_SPLINE_SURFACE_WITH_KNOTS('',3,1,((#54329,#54330),(#54331,#54332),
(#54333,#54334),(#54335,#54336),(#54337,#54338),(#54339,#54340),(#54341,
#54342),(#54343,#54344),(#54345,#54346),(#54347,#54348),(#54349,#54350),
(#54351,#54352),(#54353,#54354)),.UNSPECIFIED.,.F.,.F.,.F.,(4,1,1,1,1,1,
1,1,1,1,4),(2,2),(0.0957470950504153,0.109373896083853,0.124999994672414,
0.140623896084155,0.156249994672345,0.171873896083925,0.187499994672267,
0.203123896083503,0.218749994672196,0.234373896084237,0.237586697755757),
(0.,0.0960000000000299),.UNSPECIFIED.);
#2292=B_SPLINE_SURFACE_WITH_KNOTS('',3,1,((#54798,#54799),(#54800,#54801),
(#54802,#54803),(#54804,#54805),(#54806,#54807),(#54808,#54809),(#54810,
#54811),(#54812,#54813)),.UNSPECIFIED.,.F.,.F.,.F.,(4,1,1,1,1,4),(2,2),
(0.929082069433556,0.93749999467052,0.953123896082011,0.968749994670447,
0.98437444807905,1.),(0.,0.0960000000000576),.UNSPECIFIED.);
#2293=B_SPLINE_SURFACE_WITH_KNOTS('',3,1,((#54826,#54827),(#54828,#54829),
(#54830,#54831),(#54832,#54833),(#54834,#54835),(#54836,#54837),(#54838,
#54839),(#54840,#54841),(#54842,#54843),(#54844,#54845),(#54846,#54847),
(#54848,#54849),(#54850,#54851)),.UNSPECIFIED.,.F.,.F.,.F.,(4,1,1,1,1,1,
1,1,1,1,4),(2,2),(0.762413293536994,0.765623896082486,0.781249994670884,
0.796873896082236,0.81249999467081,0.828123896082074,0.843749994670738,
0.859373896082214,0.874999994670666,0.890623896082302,0.904252893905486),
(0.,0.0960000000000257),.UNSPECIFIED.);
#2294=B_SPLINE_SURFACE_WITH_KNOTS('',3,1,((#54867,#54868),(#54869,#54870),
(#54871,#54872),(#54873,#54874),(#54875,#54876),(#54877,#54878),(#54879,
#54880),(#54881,#54882),(#54883,#54884),(#54885,#54886),(#54887,#54888),
(#54889,#54890),(#54891,#54892)),.UNSPECIFIED.,.F.,.F.,.F.,(4,1,1,1,1,1,
1,1,1,1,4),(2,2),(0.595747095084501,0.609373896082918,0.624999994671249,
0.640623896082655,0.656249994671175,0.671873896082594,0.687499994671103,
0.703123896082594,0.71874999467103,0.734373896082564,0.737586697754574),
(0.,0.0960000000000214),.UNSPECIFIED.);
#2295=B_SPLINE_SURFACE_WITH_KNOTS('',3,1,((#54908,#54909),(#54910,#54911),
(#54912,#54913),(#54914,#54915),(#54916,#54917),(#54918,#54919),(#54920,
#54921),(#54922,#54923),(#54924,#54925),(#54926,#54927),(#54928,#54929),
(#54930,#54931),(#54932,#54933)),.UNSPECIFIED.,.F.,.F.,.F.,(4,1,1,1,1,1,
1,1,1,1,4),(2,2),(0.429082069011431,0.437499994671687,0.453123896083315,
0.468749994671613,0.484373896083147,0.499999994671541,0.515623896083591,
0.531249994671472,0.546873896083833,0.562499994671398,0.570917921352938),
(0.,0.0960000000000299),.UNSPECIFIED.);
#2296=B_SPLINE_SURFACE_WITH_KNOTS('',1,3,((#55079,#55080,#55081,#55082,
#55083,#55084,#55085,#55086,#55087,#55088,#55089,#55090,#55091,#55092,#55093,
#55094,#55095,#55096,#55097,#55098),(#55099,#55100,#55101,#55102,#55103,
#55104,#55105,#55106,#55107,#55108,#55109,#55110,#55111,#55112,#55113,#55114,
#55115,#55116,#55117,#55118)),.UNSPECIFIED.,.F.,.F.,.F.,(2,2),(4,2,2,2,
2,2,2,2,2,4),(0.,1.),(0.,0.25,0.375,0.4375,0.46875,0.484375,0.4921875,0.5,
0.75,1.),.UNSPECIFIED.);
#2297=B_SPLINE_SURFACE_WITH_KNOTS('',1,3,((#55185,#55186,#55187,#55188,
#55189,#55190,#55191,#55192,#55193,#55194,#55195,#55196,#55197,#55198,#55199,
#55200,#55201,#55202,#55203,#55204),(#55205,#55206,#55207,#55208,#55209,
#55210,#55211,#55212,#55213,#55214,#55215,#55216,#55217,#55218,#55219,#55220,
#55221,#55222,#55223,#55224)),.UNSPECIFIED.,.F.,.F.,.F.,(2,2),(4,2,2,2,
2,2,2,2,2,4),(0.,1.),(0.,0.25,0.375,0.4375,0.46875,0.484375,0.4921875,0.5,
0.75,1.),.UNSPECIFIED.);
#2298=B_SPLINE_SURFACE_WITH_KNOTS('',1,3,((#55308,#55309,#55310,#55311,
#55312,#55313,#55314,#55315,#55316,#55317,#55318,#55319,#55320,#55321,#55322,
#55323,#55324,#55325,#55326,#55327),(#55328,#55329,#55330,#55331,#55332,
#55333,#55334,#55335,#55336,#55337,#55338,#55339,#55340,#55341,#55342,#55343,
#55344,#55345,#55346,#55347)),.UNSPECIFIED.,.F.,.F.,.F.,(2,2),(4,2,2,2,
2,2,2,2,2,4),(0.,1.),(0.,0.25,0.375,0.4375,0.46875,0.484375,0.4921875,0.5,
0.75,1.),.UNSPECIFIED.);
#2299=B_SPLINE_SURFACE_WITH_KNOTS('',1,3,((#55414,#55415,#55416,#55417,
#55418,#55419,#55420,#55421,#55422,#55423,#55424,#55425,#55426,#55427,#55428,
#55429,#55430,#55431,#55432,#55433),(#55434,#55435,#55436,#55437,#55438,
#55439,#55440,#55441,#55442,#55443,#55444,#55445,#55446,#55447,#55448,#55449,
#55450,#55451,#55452,#55453)),.UNSPECIFIED.,.F.,.F.,.F.,(2,2),(4,2,2,2,
2,2,2,2,2,4),(0.,1.),(0.,0.25,0.375,0.4375,0.46875,0.484375,0.4921875,0.5,
0.75,1.),.UNSPECIFIED.);
#2300=B_SPLINE_SURFACE_WITH_KNOTS('',3,1,((#56240,#56241),(#56242,#56243),
(#56244,#56245),(#56246,#56247),(#56248,#56249),(#56250,#56251),(#56252,
#56253),(#56254,#56255),(#56256,#56257),(#56258,#56259),(#56260,#56261),
(#56262,#56263),(#56264,#56265)),.UNSPECIFIED.,.F.,.F.,.F.,(4,1,1,1,1,1,
1,1,1,1,4),(2,2),(0.262413293538176,0.265623896084184,0.281249994672051,
0.296873896083354,0.312499994671976,0.328123896083308,0.343749994671905,
0.359373896083431,0.374999994671832,0.390623896083659,0.404252893941946),
(0.,0.0960000000000214),.UNSPECIFIED.);
#2301=B_SPLINE_SURFACE_WITH_KNOTS('',3,1,((#56296,#56297),(#56298,#56299),
(#56300,#56301),(#56302,#56303),(#56304,#56305),(#56306,#56307),(#56308,
#56309),(#56310,#56311)),.UNSPECIFIED.,.F.,.F.,.F.,(4,1,1,1,1,4),(2,2),
(0.,0.0245809641902474,0.0558309641902474,0.0870809641902473,0.118330964190247,
0.132495920587091),(0.,0.096000000000015),.UNSPECIFIED.);
#2302=B_SPLINE_SURFACE_WITH_KNOTS('',3,1,((#56314,#56315),(#56316,#56317),
(#56318,#56319),(#56320,#56321),(#56322,#56323),(#56324,#56325),(#56326,
#56327),(#56328,#56329)),.UNSPECIFIED.,.F.,.F.,.F.,(4,1,1,1,1,4),(2,2),
(0.26406132121346,0.28125,0.3125,0.34375,0.375,0.402605614421673),(0.,0.0960000000000342),
 .UNSPECIFIED.);
#2303=B_SPLINE_SURFACE_WITH_KNOTS('',3,1,((#56331,#56332),(#56333,#56334),
(#56335,#56336),(#56337,#56338),(#56339,#56340),(#56341,#56342),(#56343,
#56344),(#56345,#56346)),.UNSPECIFIED.,.F.,.F.,.F.,(4,1,1,1,1,4),(2,2),
(0.,0.0141649563968439,0.0454149563968439,0.0766649563968438,0.107914956396844,
0.132495920587091),(0.,0.0959999999999916),.UNSPECIFIED.);
#2304=B_SPLINE_SURFACE_WITH_KNOTS('',3,1,((#56349,#56350),(#56351,#56352),
(#56353,#56354),(#56355,#56356),(#56357,#56358),(#56359,#56360),(#56361,
#56362),(#56363,#56364)),.UNSPECIFIED.,.F.,.F.,.F.,(4,1,1,1,1,4),(2,2),
(0.0973943855783285,0.125,0.15625,0.1875,0.21875,0.235938678786541),(0.,
0.0960000000000321),.UNSPECIFIED.);
#2305=B_SPLINE_SURFACE_WITH_KNOTS('',3,1,((#56366,#56367),(#56368,#56369),
(#56370,#56371),(#56372,#56373),(#56374,#56375),(#56376,#56377)),
 .UNSPECIFIED.,.F.,.F.,.F.,(4,1,1,4),(2,2),(0.,0.03125,0.0625,0.0662486727636835),
(0.,0.0960000000000193),.UNSPECIFIED.);
#2306=B_SPLINE_SURFACE_WITH_KNOTS('',3,1,((#56378,#56379),(#56380,#56381),
(#56382,#56383),(#56384,#56385),(#56386,#56387),(#56388,#56389)),
 .UNSPECIFIED.,.F.,.F.,.F.,(4,1,1,4),(2,2),(0.,0.03125,0.0625,0.0692715472303151),
(0.,0.0960000000000278),.UNSPECIFIED.);
#2307=B_SPLINE_SURFACE_WITH_KNOTS('',3,1,((#56391,#56392),(#56393,#56394),
(#56395,#56396),(#56397,#56398),(#56399,#56400),(#56401,#56402),(#56403,
#56404),(#56405,#56406)),.UNSPECIFIED.,.F.,.F.,.F.,(4,1,1,1,1,4),(2,2),
(0.,0.0245809641902476,0.0558309641902476,0.0870809641902475,0.118330964190247,
0.132495920587092),(0.,0.0959999999999617),.UNSPECIFIED.);
#2308=B_SPLINE_SURFACE_WITH_KNOTS('',3,1,((#56408,#56409),(#56410,#56411),
(#56412,#56413),(#56414,#56415),(#56416,#56417),(#56418,#56419),(#56420,
#56421),(#56422,#56423)),.UNSPECIFIED.,.F.,.F.,.F.,(4,1,1,1,1,4),(2,2),
(0.76406132121346,0.78125,0.8125,0.84375,0.875,0.902605614421672),(0.,0.0960000000000022),
 .UNSPECIFIED.);
#2309=B_SPLINE_SURFACE_WITH_KNOTS('',3,1,((#56426,#56427),(#56428,#56429),
(#56430,#56431),(#56432,#56433),(#56434,#56435),(#56436,#56437),(#56438,
#56439),(#56440,#56441)),.UNSPECIFIED.,.F.,.F.,.F.,(4,1,1,1,1,4),(2,2),
(0.,0.0141649563968442,0.0454149563968442,0.0766649563968441,0.107914956396844,
0.132495920587091),(0.,0.0959999999999745),.UNSPECIFIED.);
#2310=B_SPLINE_SURFACE_WITH_KNOTS('',3,1,((#56443,#56444),(#56445,#56446),
(#56447,#56448),(#56449,#56450),(#56451,#56452),(#56453,#56454),(#56455,
#56456),(#56457,#56458)),.UNSPECIFIED.,.F.,.F.,.F.,(4,1,1,1,1,4),(2,2),
(0.597394385578329,0.625,0.65625,0.6875,0.71875,0.735938678786541),(0.,
0.0960000000000129),.UNSPECIFIED.);
#2311=B_SPLINE_SURFACE_WITH_KNOTS('',3,1,((#56461,#56462),(#56463,#56464),
(#56465,#56466),(#56467,#56468),(#56469,#56470),(#56471,#56472),(#56473,
#56474),(#56475,#56476),(#56477,#56478)),.UNSPECIFIED.,.F.,.F.,.F.,(4,1,
1,1,1,1,4),(2,2),(0.430728452769685,0.4375,0.46875,0.5,0.53125,0.5625,0.569271547230316),
(0.,0.0959999999999958),.UNSPECIFIED.);
#2312=B_SPLINE_SURFACE_WITH_KNOTS('',3,1,((#56481,#56482),(#56483,#56484),
(#56485,#56486),(#56487,#56488),(#56489,#56490),(#56491,#56492),(#56493,
#56494),(#56495,#56496),(#56497,#56498)),.UNSPECIFIED.,.F.,.F.,.F.,(4,1,
1,1,1,1,4),(2,2),(0.,0.00374867276368307,0.034998672763683,0.0662486727636831,
0.0974986727636831,0.128748672763683,0.132497345527366),(0.,0.0959999999999873),
 .UNSPECIFIED.);
#2313=B_SPLINE_SURFACE_WITH_KNOTS('',3,1,((#56500,#56501),(#56502,#56503),
(#56504,#56505),(#56506,#56507),(#56508,#56509),(#56510,#56511),(#56512,
#56513),(#56514,#56515)),.UNSPECIFIED.,.F.,.F.,.F.,(4,1,1,1,1,4),(2,2),
(0.,0.0116479154473907,0.0428979154473907,0.0741479154473907,0.105397915447391,
0.106629022825536),(0.,0.0960000000000235),.UNSPECIFIED.);
#2314=B_SPLINE_SURFACE_WITH_KNOTS('',3,1,((#56518,#56519),(#56520,#56521),
(#56522,#56523),(#56524,#56525),(#56526,#56527),(#56528,#56529),(#56530,
#56531),(#56532,#56533)),.UNSPECIFIED.,.F.,.F.,.F.,(4,1,1,1,1,4),(2,2),
(0.271771373885705,0.28125,0.3125,0.34375,0.375,0.394896231061528),(0.,
0.0959999999999894),.UNSPECIFIED.);
#2315=B_SPLINE_SURFACE_WITH_KNOTS('',3,1,((#56535,#56536),(#56537,#56538),
(#56539,#56540),(#56541,#56542),(#56543,#56544),(#56545,#56546),(#56547,
#56548),(#56549,#56550)),.UNSPECIFIED.,.F.,.F.,.F.,(4,1,1,1,1,4),(2,2),
(0.,0.00123110737814575,0.0324811073781457,0.0637311073781457,0.0949811073781457,
0.106629022825536),(0.,0.0960000000000043),.UNSPECIFIED.);
#2316=B_SPLINE_SURFACE_WITH_KNOTS('',3,1,((#56553,#56554),(#56555,#56556),
(#56557,#56558),(#56559,#56560),(#56561,#56562),(#56563,#56564),(#56565,
#56566),(#56567,#56568)),.UNSPECIFIED.,.F.,.F.,.F.,(4,1,1,1,1,4),(2,2),
(0.105103768938473,0.125,0.15625,0.1875,0.21875,0.228228626114295),(0.,
0.0959999999999894),.UNSPECIFIED.);
#2317=B_SPLINE_SURFACE_WITH_KNOTS('',3,1,((#56570,#56571),(#56572,#56573),
(#56574,#56575),(#56576,#56577),(#56578,#56579)),.UNSPECIFIED.,.F.,.F.,
 .F.,(4,1,4),(2,2),(0.,0.0312500000000001,0.0533131646711191),(0.,0.0960000000000768),
 .UNSPECIFIED.);
#2318=B_SPLINE_SURFACE_WITH_KNOTS('',3,1,((#56580,#56581),(#56582,#56583),
(#56584,#56585),(#56586,#56587),(#56588,#56589)),.UNSPECIFIED.,.F.,.F.,
 .F.,(4,1,4),(2,2),(0.,0.03125,0.0615627359472197),(0.,0.0960000000000001),
 .UNSPECIFIED.);
#2319=B_SPLINE_SURFACE_WITH_KNOTS('',3,1,((#56591,#56592),(#56593,#56594),
(#56595,#56596),(#56597,#56598),(#56599,#56600),(#56601,#56602),(#56603,
#56604),(#56605,#56606)),.UNSPECIFIED.,.F.,.F.,.F.,(4,1,1,1,1,4),(2,2),
(0.,0.0116479154473909,0.0428979154473909,0.0741479154473906,0.105397915447391,
0.106629022825536),(0.,0.0960000000000491),.UNSPECIFIED.);
#2320=B_SPLINE_SURFACE_WITH_KNOTS('',3,1,((#56608,#56609),(#56610,#56611),
(#56612,#56613),(#56614,#56615),(#56616,#56617),(#56618,#56619),(#56620,
#56621),(#56622,#56623)),.UNSPECIFIED.,.F.,.F.,.F.,(4,1,1,1,1,4),(2,2),
(0.771771373885705,0.78125,0.8125,0.84375,0.875,0.894896231061527),(0.,
0.0960000000000001),.UNSPECIFIED.);
#2321=B_SPLINE_SURFACE_WITH_KNOTS('',3,1,((#56626,#56627),(#56628,#56629),
(#56630,#56631),(#56632,#56633),(#56634,#56635),(#56636,#56637),(#56638,
#56639),(#56640,#56641)),.UNSPECIFIED.,.F.,.F.,.F.,(4,1,1,1,1,4),(2,2),
(0.,0.00123110737814613,0.0324811073781462,0.063731107378146,0.0949811073781461,
0.106629022825536),(0.,0.0960000000000043),.UNSPECIFIED.);
#2322=B_SPLINE_SURFACE_WITH_KNOTS('',3,1,((#56643,#56644),(#56645,#56646),
(#56647,#56648),(#56649,#56650),(#56651,#56652),(#56653,#56654),(#56655,
#56656),(#56657,#56658)),.UNSPECIFIED.,.F.,.F.,.F.,(4,1,1,1,1,4),(2,2),
(0.605103768938473,0.625,0.65625,0.6875,0.71875,0.728228626114296),(0.,
0.0959999999999873),.UNSPECIFIED.);
#2323=B_SPLINE_SURFACE_WITH_KNOTS('',3,1,((#56661,#56662),(#56663,#56664),
(#56665,#56666),(#56667,#56668),(#56669,#56670),(#56671,#56672),(#56673,
#56674)),.UNSPECIFIED.,.F.,.F.,.F.,(4,1,1,1,4),(2,2),(0.43843726405327,
0.46875,0.5,0.53125,0.561562735946731),(0.,0.0960000000000065),
 .UNSPECIFIED.);
#2324=B_SPLINE_SURFACE_WITH_KNOTS('',3,1,((#56677,#56678),(#56679,#56680),
(#56681,#56682),(#56683,#56684),(#56685,#56686),(#56687,#56688),(#56689,
#56690)),.UNSPECIFIED.,.F.,.F.,.F.,(4,1,1,1,4),(2,2),(0.,0.0220631642961554,
0.0533131642961553,0.0845631642961553,0.10662632859231),(0.,0.0960000000000299),
 .UNSPECIFIED.);
#2325=B_SPLINE_SURFACE_WITH_KNOTS('',3,1,((#56692,#56693),(#56694,#56695),
(#56696,#56697),(#56698,#56699),(#56700,#56701),(#56702,#56703)),
 .UNSPECIFIED.,.F.,.F.,.F.,(4,1,1,4),(2,2),(0.301135800019707,0.3125,0.34375,
0.365533173173181),(0.,0.0959999999999553),.UNSPECIFIED.);
#2326=B_SPLINE_SURFACE_WITH_KNOTS('',3,1,((#56705,#56706),(#56707,#56708),
(#56709,#56710),(#56711,#56712),(#56713,#56714),(#56715,#56716)),
 .UNSPECIFIED.,.F.,.F.,.F.,(4,1,1,4),(2,2),(0.134466826826819,0.15625,0.1875,
0.198864199980294),(0.,0.0959999999999489),.UNSPECIFIED.);
#2327=B_SPLINE_SURFACE_WITH_KNOTS('',3,1,((#56718,#56719),(#56720,#56721),
(#56722,#56723),(#56724,#56725),(#56726,#56727)),.UNSPECIFIED.,.F.,.F.,
 .F.,(4,1,4),(2,2),(0.,0.03125,0.0321982303893307),(0.,0.0959999999999532),
 .UNSPECIFIED.);
#2328=B_SPLINE_SURFACE_WITH_KNOTS('',3,1,((#56729,#56730),(#56731,#56732),
(#56733,#56734),(#56735,#56736),(#56737,#56738),(#56739,#56740)),
 .UNSPECIFIED.,.F.,.F.,.F.,(4,1,1,4),(2,2),(0.801135800019707,0.8125,0.84375,
0.86553317317318),(0.,0.0959999999999511),.UNSPECIFIED.);
#2329=B_SPLINE_SURFACE_WITH_KNOTS('',3,1,((#56743,#56744),(#56745,#56746),
(#56747,#56748),(#56749,#56750),(#56751,#56752),(#56753,#56754)),
 .UNSPECIFIED.,.F.,.F.,.F.,(4,1,1,4),(2,2),(0.63446682682682,0.65625,0.6875,
0.698864199980293),(0.,0.0959999999999106),.UNSPECIFIED.);
#2330=B_SPLINE_SURFACE_WITH_KNOTS('',3,1,((#56757,#56758),(#56759,#56760),
(#56761,#56762),(#56763,#56764),(#56765,#56766),(#56767,#56768),(#56769,
#56770)),.UNSPECIFIED.,.F.,.F.,.F.,(4,1,1,1,4),(2,2),(0.467801769610687,
0.46875,0.5,0.53125,0.532198230389314),(0.,0.0959999999999468),
 .UNSPECIFIED.);
#2331=FACE_OUTER_BOUND('',#4245,.T.);
#2332=FACE_OUTER_BOUND('',#4246,.T.);
#2333=FACE_OUTER_BOUND('',#4247,.T.);
#2334=FACE_OUTER_BOUND('',#4248,.T.);
#2335=FACE_OUTER_BOUND('',#4249,.T.);
#2336=FACE_OUTER_BOUND('',#4250,.T.);
#2337=FACE_OUTER_BOUND('',#4251,.T.);
#2338=FACE_OUTER_BOUND('',#4252,.T.);
#2339=FACE_OUTER_BOUND('',#4253,.T.);
#2340=FACE_OUTER_BOUND('',#4254,.T.);
#2341=FACE_OUTER_BOUND('',#4255,.T.);
#2342=FACE_OUTER_BOUND('',#4256,.T.);
#2343=FACE_OUTER_BOUND('',#4257,.T.);
#2344=FACE_OUTER_BOUND('',#4258,.T.);
#2345=FACE_OUTER_BOUND('',#4259,.T.);
#2346=FACE_OUTER_BOUND('',#4260,.T.);
#2347=FACE_OUTER_BOUND('',#4261,.T.);
#2348=FACE_OUTER_BOUND('',#4262,.T.);
#2349=FACE_OUTER_BOUND('',#4263,.T.);
#2350=FACE_OUTER_BOUND('',#4264,.T.);
#2351=FACE_OUTER_BOUND('',#4265,.T.);
#2352=FACE_OUTER_BOUND('',#4266,.T.);
#2353=FACE_OUTER_BOUND('',#4267,.T.);
#2354=FACE_OUTER_BOUND('',#4268,.T.);
#2355=FACE_OUTER_BOUND('',#4269,.T.);
#2356=FACE_OUTER_BOUND('',#4270,.T.);
#2357=FACE_OUTER_BOUND('',#4271,.T.);
#2358=FACE_OUTER_BOUND('',#4272,.T.);
#2359=FACE_OUTER_BOUND('',#4273,.T.);
#2360=FACE_OUTER_BOUND('',#4274,.T.);
#2361=FACE_OUTER_BOUND('',#4275,.T.);
#2362=FACE_OUTER_BOUND('',#4276,.T.);
#2363=FACE_OUTER_BOUND('',#4277,.T.);
#2364=FACE_OUTER_BOUND('',#4278,.T.);
#2365=FACE_OUTER_BOUND('',#4279,.T.);
#2366=FACE_OUTER_BOUND('',#4280,.T.);
#2367=FACE_OUTER_BOUND('',#4281,.T.);
#2368=FACE_OUTER_BOUND('',#4282,.T.);
#2369=FACE_OUTER_BOUND('',#4283,.T.);
#2370=FACE_OUTER_BOUND('',#4284,.T.);
#2371=FACE_OUTER_BOUND('',#4285,.T.);
#2372=FACE_OUTER_BOUND('',#4286,.T.);
#2373=FACE_OUTER_BOUND('',#4287,.T.);
#2374=FACE_OUTER_BOUND('',#4288,.T.);
#2375=FACE_OUTER_BOUND('',#4289,.T.);
#2376=FACE_OUTER_BOUND('',#4290,.T.);
#2377=FACE_OUTER_BOUND('',#4291,.T.);
#2378=FACE_OUTER_BOUND('',#4292,.T.);
#2379=FACE_OUTER_BOUND('',#4293,.T.);
#2380=FACE_OUTER_BOUND('',#4294,.T.);
#2381=FACE_OUTER_BOUND('',#4295,.T.);
#2382=FACE_OUTER_BOUND('',#4296,.T.);
#2383=FACE_OUTER_BOUND('',#4297,.T.);
#2384=FACE_OUTER_BOUND('',#4298,.T.);
#2385=FACE_OUTER_BOUND('',#4299,.T.);
#2386=FACE_OUTER_BOUND('',#4300,.T.);
#2387=FACE_OUTER_BOUND('',#4301,.T.);
#2388=FACE_OUTER_BOUND('',#4302,.T.);
#2389=FACE_OUTER_BOUND('',#4303,.T.);
#2390=FACE_OUTER_BOUND('',#4304,.T.);
#2391=FACE_OUTER_BOUND('',#4305,.T.);
#2392=FACE_OUTER_BOUND('',#4306,.T.);
#2393=FACE_OUTER_BOUND('',#4307,.T.);
#2394=FACE_OUTER_BOUND('',#4308,.T.);
#2395=FACE_OUTER_BOUND('',#4309,.T.);
#2396=FACE_OUTER_BOUND('',#4310,.T.);
#2397=FACE_OUTER_BOUND('',#4311,.T.);
#2398=FACE_OUTER_BOUND('',#4312,.T.);
#2399=FACE_OUTER_BOUND('',#4313,.T.);
#2400=FACE_OUTER_BOUND('',#4314,.T.);
#2401=FACE_OUTER_BOUND('',#4315,.T.);
#2402=FACE_OUTER_BOUND('',#4316,.T.);
#2403=FACE_OUTER_BOUND('',#4317,.T.);
#2404=FACE_OUTER_BOUND('',#4318,.T.);
#2405=FACE_OUTER_BOUND('',#4319,.T.);
#2406=FACE_OUTER_BOUND('',#4320,.T.);
#2407=FACE_OUTER_BOUND('',#4321,.T.);
#2408=FACE_OUTER_BOUND('',#4322,.T.);
#2409=FACE_OUTER_BOUND('',#4323,.T.);
#2410=FACE_OUTER_BOUND('',#4324,.T.);
#2411=FACE_OUTER_BOUND('',#4325,.T.);
#2412=FACE_OUTER_BOUND('',#4326,.T.);
#2413=FACE_OUTER_BOUND('',#4327,.T.);
#2414=FACE_OUTER_BOUND('',#4328,.T.);
#2415=FACE_OUTER_BOUND('',#4329,.T.);
#2416=FACE_OUTER_BOUND('',#4330,.T.);
#2417=FACE_OUTER_BOUND('',#4331,.T.);
#2418=FACE_OUTER_BOUND('',#4332,.T.);
#2419=FACE_OUTER_BOUND('',#4333,.T.);
#2420=FACE_OUTER_BOUND('',#4334,.T.);
#2421=FACE_OUTER_BOUND('',#4335,.T.);
#2422=FACE_OUTER_BOUND('',#4340,.T.);
#2423=FACE_OUTER_BOUND('',#4345,.T.);
#2424=FACE_OUTER_BOUND('',#4346,.T.);
#2425=FACE_OUTER_BOUND('',#4347,.T.);
#2426=FACE_OUTER_BOUND('',#4350,.T.);
#2427=FACE_OUTER_BOUND('',#4353,.T.);
#2428=FACE_OUTER_BOUND('',#4354,.T.);
#2429=FACE_OUTER_BOUND('',#4355,.T.);
#2430=FACE_OUTER_BOUND('',#4404,.T.);
#2431=FACE_OUTER_BOUND('',#4453,.T.);
#2432=FACE_OUTER_BOUND('',#4454,.T.);
#2433=FACE_OUTER_BOUND('',#4455,.T.);
#2434=FACE_OUTER_BOUND('',#4456,.T.);
#2435=FACE_OUTER_BOUND('',#4457,.T.);
#2436=FACE_OUTER_BOUND('',#4458,.T.);
#2437=FACE_OUTER_BOUND('',#4459,.T.);
#2438=FACE_OUTER_BOUND('',#4460,.T.);
#2439=FACE_OUTER_BOUND('',#4461,.T.);
#2440=FACE_OUTER_BOUND('',#4462,.T.);
#2441=FACE_OUTER_BOUND('',#4463,.T.);
#2442=FACE_OUTER_BOUND('',#4464,.T.);
#2443=FACE_OUTER_BOUND('',#4465,.T.);
#2444=FACE_OUTER_BOUND('',#4466,.T.);
#2445=FACE_OUTER_BOUND('',#4467,.T.);
#2446=FACE_OUTER_BOUND('',#4468,.T.);
#2447=FACE_OUTER_BOUND('',#4469,.T.);
#2448=FACE_OUTER_BOUND('',#4470,.T.);
#2449=FACE_OUTER_BOUND('',#4471,.T.);
#2450=FACE_OUTER_BOUND('',#4472,.T.);
#2451=FACE_OUTER_BOUND('',#4473,.T.);
#2452=FACE_OUTER_BOUND('',#4474,.T.);
#2453=FACE_OUTER_BOUND('',#4475,.T.);
#2454=FACE_OUTER_BOUND('',#4476,.T.);
#2455=FACE_OUTER_BOUND('',#4477,.T.);
#2456=FACE_OUTER_BOUND('',#4478,.T.);
#2457=FACE_OUTER_BOUND('',#4497,.T.);
#2458=FACE_OUTER_BOUND('',#4498,.T.);
#2459=FACE_OUTER_BOUND('',#4499,.T.);
#2460=FACE_OUTER_BOUND('',#4500,.T.);
#2461=FACE_OUTER_BOUND('',#4501,.T.);
#2462=FACE_OUTER_BOUND('',#4502,.T.);
#2463=FACE_OUTER_BOUND('',#4514,.T.);
#2464=FACE_OUTER_BOUND('',#4526,.T.);
#2465=FACE_OUTER_BOUND('',#4527,.T.);
#2466=FACE_OUTER_BOUND('',#4528,.T.);
#2467=FACE_OUTER_BOUND('',#4529,.T.);
#2468=FACE_OUTER_BOUND('',#4530,.T.);
#2469=FACE_OUTER_BOUND('',#4531,.T.);
#2470=FACE_OUTER_BOUND('',#4532,.T.);
#2471=FACE_OUTER_BOUND('',#4533,.T.);
#2472=FACE_OUTER_BOUND('',#4534,.T.);
#2473=FACE_OUTER_BOUND('',#4535,.T.);
#2474=FACE_OUTER_BOUND('',#4536,.T.);
#2475=FACE_OUTER_BOUND('',#4537,.T.);
#2476=FACE_OUTER_BOUND('',#4538,.T.);
#2477=FACE_OUTER_BOUND('',#4539,.T.);
#2478=FACE_OUTER_BOUND('',#4540,.T.);
#2479=FACE_OUTER_BOUND('',#4541,.T.);
#2480=FACE_OUTER_BOUND('',#4542,.T.);
#2481=FACE_OUTER_BOUND('',#4543,.T.);
#2482=FACE_OUTER_BOUND('',#4544,.T.);
#2483=FACE_OUTER_BOUND('',#4545,.T.);
#2484=FACE_OUTER_BOUND('',#4546,.T.);
#2485=FACE_OUTER_BOUND('',#4547,.T.);
#2486=FACE_OUTER_BOUND('',#4548,.T.);
#2487=FACE_OUTER_BOUND('',#4549,.T.);
#2488=FACE_OUTER_BOUND('',#4550,.T.);
#2489=FACE_OUTER_BOUND('',#4551,.T.);
#2490=FACE_OUTER_BOUND('',#4552,.T.);
#2491=FACE_OUTER_BOUND('',#4553,.T.);
#2492=FACE_OUTER_BOUND('',#4554,.T.);
#2493=FACE_OUTER_BOUND('',#4555,.T.);
#2494=FACE_OUTER_BOUND('',#4556,.T.);
#2495=FACE_OUTER_BOUND('',#4557,.T.);
#2496=FACE_OUTER_BOUND('',#4558,.T.);
#2497=FACE_OUTER_BOUND('',#4559,.T.);
#2498=FACE_OUTER_BOUND('',#4560,.T.);
#2499=FACE_OUTER_BOUND('',#4561,.T.);
#2500=FACE_OUTER_BOUND('',#4562,.T.);
#2501=FACE_OUTER_BOUND('',#4563,.T.);
#2502=FACE_OUTER_BOUND('',#4564,.T.);
#2503=FACE_OUTER_BOUND('',#4565,.T.);
#2504=FACE_OUTER_BOUND('',#4566,.T.);
#2505=FACE_OUTER_BOUND('',#4568,.T.);
#2506=FACE_OUTER_BOUND('',#4569,.T.);
#2507=FACE_OUTER_BOUND('',#4570,.T.);
#2508=FACE_OUTER_BOUND('',#4571,.T.);
#2509=FACE_OUTER_BOUND('',#4572,.T.);
#2510=FACE_OUTER_BOUND('',#4573,.T.);
#2511=FACE_OUTER_BOUND('',#4574,.T.);
#2512=FACE_OUTER_BOUND('',#4576,.T.);
#2513=FACE_OUTER_BOUND('',#4577,.T.);
#2514=FACE_OUTER_BOUND('',#4578,.T.);
#2515=FACE_OUTER_BOUND('',#4579,.T.);
#2516=FACE_OUTER_BOUND('',#4580,.T.);
#2517=FACE_OUTER_BOUND('',#4581,.T.);
#2518=FACE_OUTER_BOUND('',#4582,.T.);
#2519=FACE_OUTER_BOUND('',#4583,.T.);
#2520=FACE_OUTER_BOUND('',#4584,.T.);
#2521=FACE_OUTER_BOUND('',#4585,.T.);
#2522=FACE_OUTER_BOUND('',#4586,.T.);
#2523=FACE_OUTER_BOUND('',#4588,.T.);
#2524=FACE_OUTER_BOUND('',#4589,.T.);
#2525=FACE_OUTER_BOUND('',#4590,.T.);
#2526=FACE_OUTER_BOUND('',#4591,.T.);
#2527=FACE_OUTER_BOUND('',#4592,.T.);
#2528=FACE_OUTER_BOUND('',#4593,.T.);
#2529=FACE_OUTER_BOUND('',#4594,.T.);
#2530=FACE_OUTER_BOUND('',#4596,.T.);
#2531=FACE_OUTER_BOUND('',#4597,.T.);
#2532=FACE_OUTER_BOUND('',#4598,.T.);
#2533=FACE_OUTER_BOUND('',#4599,.T.);
#2534=FACE_OUTER_BOUND('',#4600,.T.);
#2535=FACE_OUTER_BOUND('',#4601,.T.);
#2536=FACE_OUTER_BOUND('',#4602,.T.);
#2537=FACE_OUTER_BOUND('',#4603,.T.);
#2538=FACE_OUTER_BOUND('',#4604,.T.);
#2539=FACE_OUTER_BOUND('',#4605,.T.);
#2540=FACE_OUTER_BOUND('',#4606,.T.);
#2541=FACE_OUTER_BOUND('',#4608,.T.);
#2542=FACE_OUTER_BOUND('',#4609,.T.);
#2543=FACE_OUTER_BOUND('',#4610,.T.);
#2544=FACE_OUTER_BOUND('',#4611,.T.);
#2545=FACE_OUTER_BOUND('',#4612,.T.);
#2546=FACE_OUTER_BOUND('',#4613,.T.);
#2547=FACE_OUTER_BOUND('',#4614,.T.);
#2548=FACE_OUTER_BOUND('',#4616,.T.);
#2549=FACE_OUTER_BOUND('',#4617,.T.);
#2550=FACE_OUTER_BOUND('',#4618,.T.);
#2551=FACE_OUTER_BOUND('',#4619,.T.);
#2552=FACE_OUTER_BOUND('',#4620,.T.);
#2553=FACE_OUTER_BOUND('',#4621,.T.);
#2554=FACE_OUTER_BOUND('',#4622,.T.);
#2555=FACE_OUTER_BOUND('',#4623,.T.);
#2556=FACE_OUTER_BOUND('',#4624,.T.);
#2557=FACE_OUTER_BOUND('',#4625,.T.);
#2558=FACE_OUTER_BOUND('',#4626,.T.);
#2559=FACE_OUTER_BOUND('',#4628,.T.);
#2560=FACE_OUTER_BOUND('',#4629,.T.);
#2561=FACE_OUTER_BOUND('',#4630,.T.);
#2562=FACE_OUTER_BOUND('',#4631,.T.);
#2563=FACE_OUTER_BOUND('',#4632,.T.);
#2564=FACE_OUTER_BOUND('',#4633,.T.);
#2565=FACE_OUTER_BOUND('',#4634,.T.);
#2566=FACE_OUTER_BOUND('',#4636,.T.);
#2567=FACE_OUTER_BOUND('',#4655,.T.);
#2568=FACE_OUTER_BOUND('',#4656,.T.);
#2569=FACE_OUTER_BOUND('',#4657,.T.);
#2570=FACE_OUTER_BOUND('',#4658,.T.);
#2571=FACE_OUTER_BOUND('',#4659,.T.);
#2572=FACE_OUTER_BOUND('',#4660,.T.);
#2573=FACE_OUTER_BOUND('',#4661,.T.);
#2574=FACE_OUTER_BOUND('',#4662,.T.);
#2575=FACE_OUTER_BOUND('',#4663,.T.);
#2576=FACE_OUTER_BOUND('',#4664,.T.);
#2577=FACE_OUTER_BOUND('',#4665,.T.);
#2578=FACE_OUTER_BOUND('',#4666,.T.);
#2579=FACE_OUTER_BOUND('',#4667,.T.);
#2580=FACE_OUTER_BOUND('',#4668,.T.);
#2581=FACE_OUTER_BOUND('',#4669,.T.);
#2582=FACE_OUTER_BOUND('',#4670,.T.);
#2583=FACE_OUTER_BOUND('',#4671,.T.);
#2584=FACE_OUTER_BOUND('',#4672,.T.);
#2585=FACE_OUTER_BOUND('',#4673,.T.);
#2586=FACE_OUTER_BOUND('',#4674,.T.);
#2587=FACE_OUTER_BOUND('',#4675,.T.);
#2588=FACE_OUTER_BOUND('',#4676,.T.);
#2589=FACE_OUTER_BOUND('',#4677,.T.);
#2590=FACE_OUTER_BOUND('',#4678,.T.);
#2591=FACE_OUTER_BOUND('',#4679,.T.);
#2592=FACE_OUTER_BOUND('',#4680,.T.);
#2593=FACE_OUTER_BOUND('',#4681,.T.);
#2594=FACE_OUTER_BOUND('',#4682,.T.);
#2595=FACE_OUTER_BOUND('',#4683,.T.);
#2596=FACE_OUTER_BOUND('',#4684,.T.);
#2597=FACE_OUTER_BOUND('',#4685,.T.);
#2598=FACE_OUTER_BOUND('',#4686,.T.);
#2599=FACE_OUTER_BOUND('',#4687,.T.);
#2600=FACE_OUTER_BOUND('',#4688,.T.);
#2601=FACE_OUTER_BOUND('',#4689,.T.);
#2602=FACE_OUTER_BOUND('',#4690,.T.);
#2603=FACE_OUTER_BOUND('',#4691,.T.);
#2604=FACE_OUTER_BOUND('',#4692,.T.);
#2605=FACE_OUTER_BOUND('',#4693,.T.);
#2606=FACE_OUTER_BOUND('',#4694,.T.);
#2607=FACE_OUTER_BOUND('',#4695,.T.);
#2608=FACE_OUTER_BOUND('',#4696,.T.);
#2609=FACE_OUTER_BOUND('',#4697,.T.);
#2610=FACE_OUTER_BOUND('',#4698,.T.);
#2611=FACE_OUTER_BOUND('',#4699,.T.);
#2612=FACE_OUTER_BOUND('',#4700,.T.);
#2613=FACE_OUTER_BOUND('',#4701,.T.);
#2614=FACE_OUTER_BOUND('',#4702,.T.);
#2615=FACE_OUTER_BOUND('',#4703,.T.);
#2616=FACE_OUTER_BOUND('',#4704,.T.);
#2617=FACE_OUTER_BOUND('',#4705,.T.);
#2618=FACE_OUTER_BOUND('',#4706,.T.);
#2619=FACE_OUTER_BOUND('',#4707,.T.);
#2620=FACE_OUTER_BOUND('',#4708,.T.);
#2621=FACE_OUTER_BOUND('',#4709,.T.);
#2622=FACE_OUTER_BOUND('',#4710,.T.);
#2623=FACE_OUTER_BOUND('',#4711,.T.);
#2624=FACE_OUTER_BOUND('',#4712,.T.);
#2625=FACE_OUTER_BOUND('',#4713,.T.);
#2626=FACE_OUTER_BOUND('',#4714,.T.);
#2627=FACE_OUTER_BOUND('',#4715,.T.);
#2628=FACE_OUTER_BOUND('',#4716,.T.);
#2629=FACE_OUTER_BOUND('',#4717,.T.);
#2630=FACE_OUTER_BOUND('',#4718,.T.);
#2631=FACE_OUTER_BOUND('',#4719,.T.);
#2632=FACE_OUTER_BOUND('',#4720,.T.);
#2633=FACE_OUTER_BOUND('',#4721,.T.);
#2634=FACE_OUTER_BOUND('',#4722,.T.);
#2635=FACE_OUTER_BOUND('',#4723,.T.);
#2636=FACE_OUTER_BOUND('',#4724,.T.);
#2637=FACE_OUTER_BOUND('',#4725,.T.);
#2638=FACE_OUTER_BOUND('',#4726,.T.);
#2639=FACE_OUTER_BOUND('',#4727,.T.);
#2640=FACE_OUTER_BOUND('',#4728,.T.);
#2641=FACE_OUTER_BOUND('',#4729,.T.);
#2642=FACE_OUTER_BOUND('',#4730,.T.);
#2643=FACE_OUTER_BOUND('',#4731,.T.);
#2644=FACE_OUTER_BOUND('',#4732,.T.);
#2645=FACE_OUTER_BOUND('',#4733,.T.);
#2646=FACE_OUTER_BOUND('',#4734,.T.);
#2647=FACE_OUTER_BOUND('',#4735,.T.);
#2648=FACE_OUTER_BOUND('',#4736,.T.);
#2649=FACE_OUTER_BOUND('',#4737,.T.);
#2650=FACE_OUTER_BOUND('',#4738,.T.);
#2651=FACE_OUTER_BOUND('',#4739,.T.);
#2652=FACE_OUTER_BOUND('',#4740,.T.);
#2653=FACE_OUTER_BOUND('',#4741,.T.);
#2654=FACE_OUTER_BOUND('',#4742,.T.);
#2655=FACE_OUTER_BOUND('',#4743,.T.);
#2656=FACE_OUTER_BOUND('',#4744,.T.);
#2657=FACE_OUTER_BOUND('',#4745,.T.);
#2658=FACE_OUTER_BOUND('',#4746,.T.);
#2659=FACE_OUTER_BOUND('',#4747,.T.);
#2660=FACE_OUTER_BOUND('',#4748,.T.);
#2661=FACE_OUTER_BOUND('',#4749,.T.);
#2662=FACE_OUTER_BOUND('',#4750,.T.);
#2663=FACE_OUTER_BOUND('',#4751,.T.);
#2664=FACE_OUTER_BOUND('',#4752,.T.);
#2665=FACE_OUTER_BOUND('',#4753,.T.);
#2666=FACE_OUTER_BOUND('',#4754,.T.);
#2667=FACE_OUTER_BOUND('',#4755,.T.);
#2668=FACE_OUTER_BOUND('',#4756,.T.);
#2669=FACE_OUTER_BOUND('',#4757,.T.);
#2670=FACE_OUTER_BOUND('',#4758,.T.);
#2671=FACE_OUTER_BOUND('',#4759,.T.);
#2672=FACE_OUTER_BOUND('',#4760,.T.);
#2673=FACE_OUTER_BOUND('',#4761,.T.);
#2674=FACE_OUTER_BOUND('',#4762,.T.);
#2675=FACE_OUTER_BOUND('',#4763,.T.);
#2676=FACE_OUTER_BOUND('',#4764,.T.);
#2677=FACE_OUTER_BOUND('',#4765,.T.);
#2678=FACE_OUTER_BOUND('',#4766,.T.);
#2679=FACE_OUTER_BOUND('',#4767,.T.);
#2680=FACE_OUTER_BOUND('',#4768,.T.);
#2681=FACE_OUTER_BOUND('',#4769,.T.);
#2682=FACE_OUTER_BOUND('',#4770,.T.);
#2683=FACE_OUTER_BOUND('',#4771,.T.);
#2684=FACE_OUTER_BOUND('',#4772,.T.);
#2685=FACE_OUTER_BOUND('',#4773,.T.);
#2686=FACE_OUTER_BOUND('',#4774,.T.);
#2687=FACE_OUTER_BOUND('',#4775,.T.);
#2688=FACE_OUTER_BOUND('',#4776,.T.);
#2689=FACE_OUTER_BOUND('',#4777,.T.);
#2690=FACE_OUTER_BOUND('',#4778,.T.);
#2691=FACE_OUTER_BOUND('',#4779,.T.);
#2692=FACE_OUTER_BOUND('',#4780,.T.);
#2693=FACE_OUTER_BOUND('',#4781,.T.);
#2694=FACE_OUTER_BOUND('',#4782,.T.);
#2695=FACE_OUTER_BOUND('',#4783,.T.);
#2696=FACE_OUTER_BOUND('',#4784,.T.);
#2697=FACE_OUTER_BOUND('',#4785,.T.);
#2698=FACE_OUTER_BOUND('',#4786,.T.);
#2699=FACE_OUTER_BOUND('',#4787,.T.);
#2700=FACE_OUTER_BOUND('',#4788,.T.);
#2701=FACE_OUTER_BOUND('',#4789,.T.);
#2702=FACE_OUTER_BOUND('',#4790,.T.);
#2703=FACE_OUTER_BOUND('',#4791,.T.);
#2704=FACE_OUTER_BOUND('',#4792,.T.);
#2705=FACE_OUTER_BOUND('',#4793,.T.);
#2706=FACE_OUTER_BOUND('',#4794,.T.);
#2707=FACE_OUTER_BOUND('',#4795,.T.);
#2708=FACE_OUTER_BOUND('',#4796,.T.);
#2709=FACE_OUTER_BOUND('',#4797,.T.);
#2710=FACE_OUTER_BOUND('',#4798,.T.);
#2711=FACE_OUTER_BOUND('',#4799,.T.);
#2712=FACE_OUTER_BOUND('',#4800,.T.);
#2713=FACE_OUTER_BOUND('',#4801,.T.);
#2714=FACE_OUTER_BOUND('',#4802,.T.);
#2715=FACE_OUTER_BOUND('',#4803,.T.);
#2716=FACE_OUTER_BOUND('',#4804,.T.);
#2717=FACE_OUTER_BOUND('',#4805,.T.);
#2718=FACE_OUTER_BOUND('',#4806,.T.);
#2719=FACE_OUTER_BOUND('',#4807,.T.);
#2720=FACE_OUTER_BOUND('',#4808,.T.);
#2721=FACE_OUTER_BOUND('',#4809,.T.);
#2722=FACE_OUTER_BOUND('',#4810,.T.);
#2723=FACE_OUTER_BOUND('',#4811,.T.);
#2724=FACE_OUTER_BOUND('',#4812,.T.);
#2725=FACE_OUTER_BOUND('',#4813,.T.);
#2726=FACE_OUTER_BOUND('',#4814,.T.);
#2727=FACE_OUTER_BOUND('',#4815,.T.);
#2728=FACE_OUTER_BOUND('',#4816,.T.);
#2729=FACE_OUTER_BOUND('',#4817,.T.);
#2730=FACE_OUTER_BOUND('',#4818,.T.);
#2731=FACE_OUTER_BOUND('',#4819,.T.);
#2732=FACE_OUTER_BOUND('',#4820,.T.);
#2733=FACE_OUTER_BOUND('',#4821,.T.);
#2734=FACE_OUTER_BOUND('',#4822,.T.);
#2735=FACE_OUTER_BOUND('',#4823,.T.);
#2736=FACE_OUTER_BOUND('',#4824,.T.);
#2737=FACE_OUTER_BOUND('',#4825,.T.);
#2738=FACE_OUTER_BOUND('',#4826,.T.);
#2739=FACE_OUTER_BOUND('',#4827,.T.);
#2740=FACE_OUTER_BOUND('',#4828,.T.);
#2741=FACE_OUTER_BOUND('',#4829,.T.);
#2742=FACE_OUTER_BOUND('',#4830,.T.);
#2743=FACE_OUTER_BOUND('',#4831,.T.);
#2744=FACE_OUTER_BOUND('',#4832,.T.);
#2745=FACE_OUTER_BOUND('',#4833,.T.);
#2746=FACE_OUTER_BOUND('',#4834,.T.);
#2747=FACE_OUTER_BOUND('',#4835,.T.);
#2748=FACE_OUTER_BOUND('',#4836,.T.);
#2749=FACE_OUTER_BOUND('',#4837,.T.);
#2750=FACE_OUTER_BOUND('',#4838,.T.);
#2751=FACE_OUTER_BOUND('',#4839,.T.);
#2752=FACE_OUTER_BOUND('',#4840,.T.);
#2753=FACE_OUTER_BOUND('',#4841,.T.);
#2754=FACE_OUTER_BOUND('',#4842,.T.);
#2755=FACE_OUTER_BOUND('',#4843,.T.);
#2756=FACE_OUTER_BOUND('',#4844,.T.);
#2757=FACE_OUTER_BOUND('',#4845,.T.);
#2758=FACE_OUTER_BOUND('',#4846,.T.);
#2759=FACE_OUTER_BOUND('',#4847,.T.);
#2760=FACE_OUTER_BOUND('',#4848,.T.);
#2761=FACE_OUTER_BOUND('',#4849,.T.);
#2762=FACE_OUTER_BOUND('',#4850,.T.);
#2763=FACE_OUTER_BOUND('',#4851,.T.);
#2764=FACE_OUTER_BOUND('',#4852,.T.);
#2765=FACE_OUTER_BOUND('',#4853,.T.);
#2766=FACE_OUTER_BOUND('',#4854,.T.);
#2767=FACE_OUTER_BOUND('',#4855,.T.);
#2768=FACE_OUTER_BOUND('',#4856,.T.);
#2769=FACE_OUTER_BOUND('',#4857,.T.);
#2770=FACE_OUTER_BOUND('',#4858,.T.);
#2771=FACE_OUTER_BOUND('',#4859,.T.);
#2772=FACE_OUTER_BOUND('',#4860,.T.);
#2773=FACE_OUTER_BOUND('',#4861,.T.);
#2774=FACE_OUTER_BOUND('',#4862,.T.);
#2775=FACE_OUTER_BOUND('',#4863,.T.);
#2776=FACE_OUTER_BOUND('',#4864,.T.);
#2777=FACE_OUTER_BOUND('',#4865,.T.);
#2778=FACE_OUTER_BOUND('',#4866,.T.);
#2779=FACE_OUTER_BOUND('',#4867,.T.);
#2780=FACE_OUTER_BOUND('',#4868,.T.);
#2781=FACE_OUTER_BOUND('',#4869,.T.);
#2782=FACE_OUTER_BOUND('',#4870,.T.);
#2783=FACE_OUTER_BOUND('',#4871,.T.);
#2784=FACE_OUTER_BOUND('',#4872,.T.);
#2785=FACE_OUTER_BOUND('',#4873,.T.);
#2786=FACE_OUTER_BOUND('',#4874,.T.);
#2787=FACE_OUTER_BOUND('',#4875,.T.);
#2788=FACE_OUTER_BOUND('',#4876,.T.);
#2789=FACE_OUTER_BOUND('',#4877,.T.);
#2790=FACE_OUTER_BOUND('',#4878,.T.);
#2791=FACE_OUTER_BOUND('',#4879,.T.);
#2792=FACE_OUTER_BOUND('',#4880,.T.);
#2793=FACE_OUTER_BOUND('',#4881,.T.);
#2794=FACE_OUTER_BOUND('',#4882,.T.);
#2795=FACE_OUTER_BOUND('',#4883,.T.);
#2796=FACE_OUTER_BOUND('',#4884,.T.);
#2797=FACE_OUTER_BOUND('',#4885,.T.);
#2798=FACE_OUTER_BOUND('',#4886,.T.);
#2799=FACE_OUTER_BOUND('',#4887,.T.);
#2800=FACE_OUTER_BOUND('',#4888,.T.);
#2801=FACE_OUTER_BOUND('',#4889,.T.);
#2802=FACE_OUTER_BOUND('',#4890,.T.);
#2803=FACE_OUTER_BOUND('',#4891,.T.);
#2804=FACE_OUTER_BOUND('',#4892,.T.);
#2805=FACE_OUTER_BOUND('',#4893,.T.);
#2806=FACE_OUTER_BOUND('',#4894,.T.);
#2807=FACE_OUTER_BOUND('',#4895,.T.);
#2808=FACE_OUTER_BOUND('',#4896,.T.);
#2809=FACE_OUTER_BOUND('',#4897,.T.);
#2810=FACE_OUTER_BOUND('',#4898,.T.);
#2811=FACE_OUTER_BOUND('',#4899,.T.);
#2812=FACE_OUTER_BOUND('',#4900,.T.);
#2813=FACE_OUTER_BOUND('',#4901,.T.);
#2814=FACE_OUTER_BOUND('',#4902,.T.);
#2815=FACE_OUTER_BOUND('',#4903,.T.);
#2816=FACE_OUTER_BOUND('',#4904,.T.);
#2817=FACE_OUTER_BOUND('',#4905,.T.);
#2818=FACE_OUTER_BOUND('',#4906,.T.);
#2819=FACE_OUTER_BOUND('',#4907,.T.);
#2820=FACE_OUTER_BOUND('',#4908,.T.);
#2821=FACE_OUTER_BOUND('',#4909,.T.);
#2822=FACE_OUTER_BOUND('',#4910,.T.);
#2823=FACE_OUTER_BOUND('',#4911,.T.);
#2824=FACE_OUTER_BOUND('',#4912,.T.);
#2825=FACE_OUTER_BOUND('',#4913,.T.);
#2826=FACE_OUTER_BOUND('',#4914,.T.);
#2827=FACE_OUTER_BOUND('',#4915,.T.);
#2828=FACE_OUTER_BOUND('',#4916,.T.);
#2829=FACE_OUTER_BOUND('',#4917,.T.);
#2830=FACE_OUTER_BOUND('',#4918,.T.);
#2831=FACE_OUTER_BOUND('',#4919,.T.);
#2832=FACE_OUTER_BOUND('',#4920,.T.);
#2833=FACE_OUTER_BOUND('',#4921,.T.);
#2834=FACE_OUTER_BOUND('',#4922,.T.);
#2835=FACE_OUTER_BOUND('',#4923,.T.);
#2836=FACE_OUTER_BOUND('',#4924,.T.);
#2837=FACE_OUTER_BOUND('',#4925,.T.);
#2838=FACE_OUTER_BOUND('',#4926,.T.);
#2839=FACE_OUTER_BOUND('',#4927,.T.);
#2840=FACE_OUTER_BOUND('',#4928,.T.);
#2841=FACE_OUTER_BOUND('',#4929,.T.);
#2842=FACE_OUTER_BOUND('',#4930,.T.);
#2843=FACE_OUTER_BOUND('',#4931,.T.);
#2844=FACE_OUTER_BOUND('',#4932,.T.);
#2845=FACE_OUTER_BOUND('',#4933,.T.);
#2846=FACE_OUTER_BOUND('',#4934,.T.);
#2847=FACE_OUTER_BOUND('',#4935,.T.);
#2848=FACE_OUTER_BOUND('',#4936,.T.);
#2849=FACE_OUTER_BOUND('',#4937,.T.);
#2850=FACE_OUTER_BOUND('',#4938,.T.);
#2851=FACE_OUTER_BOUND('',#4939,.T.);
#2852=FACE_OUTER_BOUND('',#4940,.T.);
#2853=FACE_OUTER_BOUND('',#4942,.T.);
#2854=FACE_OUTER_BOUND('',#4943,.T.);
#2855=FACE_OUTER_BOUND('',#4944,.T.);
#2856=FACE_OUTER_BOUND('',#4945,.T.);
#2857=FACE_OUTER_BOUND('',#4946,.T.);
#2858=FACE_OUTER_BOUND('',#4947,.T.);
#2859=FACE_OUTER_BOUND('',#4948,.T.);
#2860=FACE_OUTER_BOUND('',#4950,.T.);
#2861=FACE_OUTER_BOUND('',#4951,.T.);
#2862=FACE_OUTER_BOUND('',#4952,.T.);
#2863=FACE_OUTER_BOUND('',#4953,.T.);
#2864=FACE_OUTER_BOUND('',#4954,.T.);
#2865=FACE_OUTER_BOUND('',#4955,.T.);
#2866=FACE_OUTER_BOUND('',#4956,.T.);
#2867=FACE_OUTER_BOUND('',#4957,.T.);
#2868=FACE_OUTER_BOUND('',#4958,.T.);
#2869=FACE_OUTER_BOUND('',#4959,.T.);
#2870=FACE_OUTER_BOUND('',#4960,.T.);
#2871=FACE_OUTER_BOUND('',#4962,.T.);
#2872=FACE_OUTER_BOUND('',#4963,.T.);
#2873=FACE_OUTER_BOUND('',#4964,.T.);
#2874=FACE_OUTER_BOUND('',#4965,.T.);
#2875=FACE_OUTER_BOUND('',#4966,.T.);
#2876=FACE_OUTER_BOUND('',#4967,.T.);
#2877=FACE_OUTER_BOUND('',#4968,.T.);
#2878=FACE_OUTER_BOUND('',#4970,.T.);
#2879=FACE_OUTER_BOUND('',#4971,.T.);
#2880=FACE_OUTER_BOUND('',#4972,.T.);
#2881=FACE_OUTER_BOUND('',#4973,.T.);
#2882=FACE_OUTER_BOUND('',#4974,.T.);
#2883=FACE_OUTER_BOUND('',#4975,.T.);
#2884=FACE_OUTER_BOUND('',#4976,.T.);
#2885=FACE_OUTER_BOUND('',#4977,.T.);
#2886=FACE_OUTER_BOUND('',#4978,.T.);
#2887=FACE_OUTER_BOUND('',#4979,.T.);
#2888=FACE_OUTER_BOUND('',#4980,.T.);
#2889=FACE_OUTER_BOUND('',#4981,.T.);
#2890=FACE_OUTER_BOUND('',#4982,.T.);
#2891=FACE_OUTER_BOUND('',#4983,.T.);
#2892=FACE_OUTER_BOUND('',#4984,.T.);
#2893=FACE_OUTER_BOUND('',#4985,.T.);
#2894=FACE_OUTER_BOUND('',#4986,.T.);
#4245=EDGE_LOOP('',(#26477,#26478,#26479,#26480));
#4246=EDGE_LOOP('',(#26481,#26482,#26483,#26484));
#4247=EDGE_LOOP('',(#26485,#26486,#26487,#26488));
#4248=EDGE_LOOP('',(#26489,#26490,#26491,#26492));
#4249=EDGE_LOOP('',(#26493,#26494,#26495,#26496));
#4250=EDGE_LOOP('',(#26497,#26498,#26499,#26500));
#4251=EDGE_LOOP('',(#26501,#26502,#26503,#26504));
#4252=EDGE_LOOP('',(#26505,#26506,#26507,#26508));
#4253=EDGE_LOOP('',(#26509,#26510,#26511,#26512));
#4254=EDGE_LOOP('',(#26513,#26514,#26515,#26516));
#4255=EDGE_LOOP('',(#26517,#26518,#26519,#26520));
#4256=EDGE_LOOP('',(#26521,#26522,#26523,#26524));
#4257=EDGE_LOOP('',(#26525,#26526,#26527,#26528));
#4258=EDGE_LOOP('',(#26529,#26530,#26531,#26532));
#4259=EDGE_LOOP('',(#26533,#26534,#26535,#26536));
#4260=EDGE_LOOP('',(#26537,#26538,#26539,#26540));
#4261=EDGE_LOOP('',(#26541,#26542,#26543,#26544));
#4262=EDGE_LOOP('',(#26545,#26546,#26547,#26548));
#4263=EDGE_LOOP('',(#26549,#26550,#26551,#26552));
#4264=EDGE_LOOP('',(#26553,#26554,#26555,#26556));
#4265=EDGE_LOOP('',(#26557,#26558,#26559,#26560));
#4266=EDGE_LOOP('',(#26561,#26562,#26563,#26564));
#4267=EDGE_LOOP('',(#26565,#26566,#26567,#26568));
#4268=EDGE_LOOP('',(#26569,#26570,#26571,#26572));
#4269=EDGE_LOOP('',(#26573,#26574,#26575,#26576));
#4270=EDGE_LOOP('',(#26577,#26578,#26579,#26580));
#4271=EDGE_LOOP('',(#26581,#26582,#26583,#26584));
#4272=EDGE_LOOP('',(#26585,#26586,#26587,#26588));
#4273=EDGE_LOOP('',(#26589,#26590,#26591,#26592));
#4274=EDGE_LOOP('',(#26593,#26594,#26595,#26596));
#4275=EDGE_LOOP('',(#26597,#26598,#26599,#26600));
#4276=EDGE_LOOP('',(#26601,#26602,#26603,#26604));
#4277=EDGE_LOOP('',(#26605,#26606,#26607,#26608));
#4278=EDGE_LOOP('',(#26609,#26610,#26611,#26612));
#4279=EDGE_LOOP('',(#26613,#26614,#26615,#26616));
#4280=EDGE_LOOP('',(#26617,#26618,#26619,#26620));
#4281=EDGE_LOOP('',(#26621,#26622,#26623,#26624));
#4282=EDGE_LOOP('',(#26625,#26626,#26627,#26628));
#4283=EDGE_LOOP('',(#26629,#26630,#26631,#26632));
#4284=EDGE_LOOP('',(#26633,#26634,#26635,#26636));
#4285=EDGE_LOOP('',(#26637,#26638,#26639,#26640));
#4286=EDGE_LOOP('',(#26641,#26642,#26643,#26644));
#4287=EDGE_LOOP('',(#26645,#26646,#26647,#26648));
#4288=EDGE_LOOP('',(#26649,#26650,#26651,#26652));
#4289=EDGE_LOOP('',(#26653,#26654,#26655,#26656));
#4290=EDGE_LOOP('',(#26657,#26658,#26659,#26660));
#4291=EDGE_LOOP('',(#26661,#26662,#26663,#26664));
#4292=EDGE_LOOP('',(#26665,#26666,#26667,#26668));
#4293=EDGE_LOOP('',(#26669,#26670,#26671,#26672));
#4294=EDGE_LOOP('',(#26673,#26674,#26675,#26676));
#4295=EDGE_LOOP('',(#26677,#26678,#26679,#26680));
#4296=EDGE_LOOP('',(#26681,#26682,#26683,#26684));
#4297=EDGE_LOOP('',(#26685,#26686,#26687,#26688));
#4298=EDGE_LOOP('',(#26689,#26690,#26691,#26692));
#4299=EDGE_LOOP('',(#26693,#26694,#26695,#26696));
#4300=EDGE_LOOP('',(#26697,#26698,#26699,#26700));
#4301=EDGE_LOOP('',(#26701,#26702,#26703,#26704));
#4302=EDGE_LOOP('',(#26705,#26706,#26707,#26708));
#4303=EDGE_LOOP('',(#26709,#26710,#26711,#26712));
#4304=EDGE_LOOP('',(#26713,#26714,#26715,#26716));
#4305=EDGE_LOOP('',(#26717,#26718,#26719,#26720));
#4306=EDGE_LOOP('',(#26721,#26722,#26723,#26724));
#4307=EDGE_LOOP('',(#26725,#26726,#26727,#26728));
#4308=EDGE_LOOP('',(#26729,#26730,#26731,#26732));
#4309=EDGE_LOOP('',(#26733,#26734,#26735,#26736));
#4310=EDGE_LOOP('',(#26737,#26738,#26739,#26740));
#4311=EDGE_LOOP('',(#26741,#26742,#26743,#26744));
#4312=EDGE_LOOP('',(#26745,#26746,#26747,#26748));
#4313=EDGE_LOOP('',(#26749,#26750,#26751,#26752));
#4314=EDGE_LOOP('',(#26753,#26754,#26755,#26756));
#4315=EDGE_LOOP('',(#26757,#26758,#26759,#26760));
#4316=EDGE_LOOP('',(#26761,#26762,#26763,#26764));
#4317=EDGE_LOOP('',(#26765,#26766,#26767,#26768));
#4318=EDGE_LOOP('',(#26769,#26770,#26771,#26772));
#4319=EDGE_LOOP('',(#26773,#26774,#26775,#26776));
#4320=EDGE_LOOP('',(#26777,#26778,#26779,#26780));
#4321=EDGE_LOOP('',(#26781,#26782,#26783,#26784));
#4322=EDGE_LOOP('',(#26785,#26786,#26787,#26788));
#4323=EDGE_LOOP('',(#26789,#26790,#26791,#26792));
#4324=EDGE_LOOP('',(#26793,#26794,#26795,#26796));
#4325=EDGE_LOOP('',(#26797,#26798,#26799,#26800));
#4326=EDGE_LOOP('',(#26801,#26802,#26803,#26804));
#4327=EDGE_LOOP('',(#26805,#26806,#26807,#26808));
#4328=EDGE_LOOP('',(#26809,#26810,#26811,#26812));
#4329=EDGE_LOOP('',(#26813,#26814,#26815,#26816));
#4330=EDGE_LOOP('',(#26817,#26818,#26819,#26820));
#4331=EDGE_LOOP('',(#26821,#26822,#26823,#26824));
#4332=EDGE_LOOP('',(#26825,#26826,#26827,#26828));
#4333=EDGE_LOOP('',(#26829,#26830,#26831,#26832));
#4334=EDGE_LOOP('',(#26833,#26834,#26835,#26836));
#4335=EDGE_LOOP('',(#26837,#26838,#26839,#26840,#26841,#26842,#26843,#26844,
#26845,#26846,#26847,#26848,#26849,#26850,#26851,#26852,#26853,#26854,#26855,
#26856,#26857,#26858,#26859,#26860,#26861,#26862,#26863,#26864));
#4336=EDGE_LOOP('',(#26865,#26866,#26867,#26868,#26869,#26870,#26871,#26872));
#4337=EDGE_LOOP('',(#26873,#26874,#26875,#26876,#26877,#26878,#26879,#26880));
#4338=EDGE_LOOP('',(#26881,#26882,#26883,#26884,#26885,#26886,#26887,#26888));
#4339=EDGE_LOOP('',(#26889,#26890,#26891,#26892,#26893,#26894,#26895,#26896));
#4340=EDGE_LOOP('',(#26897,#26898,#26899,#26900,#26901,#26902,#26903,#26904,
#26905,#26906,#26907,#26908,#26909,#26910,#26911,#26912,#26913,#26914,#26915,
#26916,#26917,#26918,#26919,#26920,#26921,#26922,#26923,#26924));
#4341=EDGE_LOOP('',(#26925,#26926,#26927,#26928));
#4342=EDGE_LOOP('',(#26929,#26930,#26931,#26932));
#4343=EDGE_LOOP('',(#26933,#26934,#26935,#26936));
#4344=EDGE_LOOP('',(#26937,#26938,#26939,#26940));
#4345=EDGE_LOOP('',(#26941,#26942,#26943,#26944));
#4346=EDGE_LOOP('',(#26945,#26946,#26947,#26948));
#4347=EDGE_LOOP('',(#26949,#26950,#26951,#26952,#26953,#26954));
#4348=EDGE_LOOP('',(#26955,#26956,#26957,#26958,#26959,#26960,#26961,#26962));
#4349=EDGE_LOOP('',(#26963,#26964,#26965,#26966,#26967,#26968,#26969,#26970));
#4350=EDGE_LOOP('',(#26971,#26972,#26973,#26974,#26975,#26976));
#4351=EDGE_LOOP('',(#26977,#26978,#26979,#26980));
#4352=EDGE_LOOP('',(#26981,#26982,#26983,#26984));
#4353=EDGE_LOOP('',(#26985,#26986,#26987,#26988));
#4354=EDGE_LOOP('',(#26989,#26990,#26991,#26992));
#4355=EDGE_LOOP('',(#26993,#26994,#26995,#26996,#26997,#26998,#26999,#27000,
#27001,#27002));
#4356=EDGE_LOOP('',(#27003,#27004,#27005,#27006));
#4357=EDGE_LOOP('',(#27007,#27008,#27009,#27010));
#4358=EDGE_LOOP('',(#27011,#27012,#27013,#27014));
#4359=EDGE_LOOP('',(#27015,#27016,#27017,#27018));
#4360=EDGE_LOOP('',(#27019,#27020,#27021,#27022));
#4361=EDGE_LOOP('',(#27023,#27024,#27025,#27026));
#4362=EDGE_LOOP('',(#27027,#27028,#27029,#27030));
#4363=EDGE_LOOP('',(#27031,#27032,#27033,#27034));
#4364=EDGE_LOOP('',(#27035,#27036,#27037,#27038));
#4365=EDGE_LOOP('',(#27039,#27040,#27041,#27042));
#4366=EDGE_LOOP('',(#27043,#27044,#27045,#27046));
#4367=EDGE_LOOP('',(#27047,#27048,#27049,#27050));
#4368=EDGE_LOOP('',(#27051,#27052,#27053,#27054));
#4369=EDGE_LOOP('',(#27055,#27056,#27057,#27058));
#4370=EDGE_LOOP('',(#27059,#27060,#27061,#27062));
#4371=EDGE_LOOP('',(#27063,#27064,#27065,#27066));
#4372=EDGE_LOOP('',(#27067,#27068,#27069,#27070));
#4373=EDGE_LOOP('',(#27071,#27072,#27073,#27074));
#4374=EDGE_LOOP('',(#27075,#27076,#27077,#27078));
#4375=EDGE_LOOP('',(#27079,#27080,#27081,#27082));
#4376=EDGE_LOOP('',(#27083,#27084,#27085,#27086));
#4377=EDGE_LOOP('',(#27087,#27088,#27089,#27090));
#4378=EDGE_LOOP('',(#27091,#27092,#27093,#27094));
#4379=EDGE_LOOP('',(#27095,#27096,#27097,#27098));
#4380=EDGE_LOOP('',(#27099,#27100,#27101,#27102));
#4381=EDGE_LOOP('',(#27103,#27104,#27105,#27106));
#4382=EDGE_LOOP('',(#27107,#27108,#27109,#27110));
#4383=EDGE_LOOP('',(#27111,#27112,#27113,#27114));
#4384=EDGE_LOOP('',(#27115,#27116,#27117,#27118));
#4385=EDGE_LOOP('',(#27119,#27120,#27121,#27122));
#4386=EDGE_LOOP('',(#27123,#27124,#27125,#27126));
#4387=EDGE_LOOP('',(#27127,#27128,#27129,#27130));
#4388=EDGE_LOOP('',(#27131,#27132,#27133,#27134));
#4389=EDGE_LOOP('',(#27135,#27136,#27137,#27138));
#4390=EDGE_LOOP('',(#27139,#27140,#27141,#27142));
#4391=EDGE_LOOP('',(#27143,#27144,#27145,#27146));
#4392=EDGE_LOOP('',(#27147,#27148,#27149,#27150));
#4393=EDGE_LOOP('',(#27151,#27152,#27153,#27154));
#4394=EDGE_LOOP('',(#27155,#27156,#27157,#27158));
#4395=EDGE_LOOP('',(#27159,#27160,#27161,#27162));
#4396=EDGE_LOOP('',(#27163,#27164,#27165,#27166));
#4397=EDGE_LOOP('',(#27167,#27168,#27169,#27170));
#4398=EDGE_LOOP('',(#27171,#27172,#27173,#27174));
#4399=EDGE_LOOP('',(#27175,#27176,#27177,#27178));
#4400=EDGE_LOOP('',(#27179,#27180,#27181,#27182));
#4401=EDGE_LOOP('',(#27183,#27184,#27185,#27186));
#4402=EDGE_LOOP('',(#27187,#27188,#27189,#27190));
#4403=EDGE_LOOP('',(#27191,#27192,#27193,#27194));
#4404=EDGE_LOOP('',(#27195,#27196,#27197,#27198,#27199,#27200,#27201,#27202,
#27203,#27204));
#4405=EDGE_LOOP('',(#27205,#27206,#27207,#27208));
#4406=EDGE_LOOP('',(#27209,#27210,#27211,#27212));
#4407=EDGE_LOOP('',(#27213,#27214,#27215,#27216));
#4408=EDGE_LOOP('',(#27217,#27218,#27219,#27220));
#4409=EDGE_LOOP('',(#27221,#27222,#27223,#27224));
#4410=EDGE_LOOP('',(#27225,#27226,#27227,#27228));
#4411=EDGE_LOOP('',(#27229,#27230,#27231,#27232));
#4412=EDGE_LOOP('',(#27233,#27234,#27235,#27236));
#4413=EDGE_LOOP('',(#27237,#27238,#27239,#27240));
#4414=EDGE_LOOP('',(#27241,#27242,#27243,#27244));
#4415=EDGE_LOOP('',(#27245,#27246,#27247,#27248));
#4416=EDGE_LOOP('',(#27249,#27250,#27251,#27252));
#4417=EDGE_LOOP('',(#27253,#27254,#27255,#27256));
#4418=EDGE_LOOP('',(#27257,#27258,#27259,#27260));
#4419=EDGE_LOOP('',(#27261,#27262,#27263,#27264));
#4420=EDGE_LOOP('',(#27265,#27266,#27267,#27268));
#4421=EDGE_LOOP('',(#27269,#27270,#27271,#27272));
#4422=EDGE_LOOP('',(#27273,#27274,#27275,#27276));
#4423=EDGE_LOOP('',(#27277,#27278,#27279,#27280));
#4424=EDGE_LOOP('',(#27281,#27282,#27283,#27284));
#4425=EDGE_LOOP('',(#27285,#27286,#27287,#27288));
#4426=EDGE_LOOP('',(#27289,#27290,#27291,#27292));
#4427=EDGE_LOOP('',(#27293,#27294,#27295,#27296));
#4428=EDGE_LOOP('',(#27297,#27298,#27299,#27300));
#4429=EDGE_LOOP('',(#27301,#27302,#27303,#27304));
#4430=EDGE_LOOP('',(#27305,#27306,#27307,#27308));
#4431=EDGE_LOOP('',(#27309,#27310,#27311,#27312));
#4432=EDGE_LOOP('',(#27313,#27314,#27315,#27316));
#4433=EDGE_LOOP('',(#27317,#27318,#27319,#27320));
#4434=EDGE_LOOP('',(#27321,#27322,#27323,#27324));
#4435=EDGE_LOOP('',(#27325,#27326,#27327,#27328));
#4436=EDGE_LOOP('',(#27329,#27330,#27331,#27332));
#4437=EDGE_LOOP('',(#27333,#27334,#27335,#27336));
#4438=EDGE_LOOP('',(#27337,#27338,#27339,#27340));
#4439=EDGE_LOOP('',(#27341,#27342,#27343,#27344));
#4440=EDGE_LOOP('',(#27345,#27346,#27347,#27348));
#4441=EDGE_LOOP('',(#27349,#27350,#27351,#27352));
#4442=EDGE_LOOP('',(#27353,#27354,#27355,#27356));
#4443=EDGE_LOOP('',(#27357,#27358,#27359,#27360));
#4444=EDGE_LOOP('',(#27361,#27362,#27363,#27364));
#4445=EDGE_LOOP('',(#27365,#27366,#27367,#27368));
#4446=EDGE_LOOP('',(#27369,#27370,#27371,#27372));
#4447=EDGE_LOOP('',(#27373,#27374,#27375,#27376));
#4448=EDGE_LOOP('',(#27377,#27378,#27379,#27380));
#4449=EDGE_LOOP('',(#27381,#27382,#27383,#27384));
#4450=EDGE_LOOP('',(#27385,#27386,#27387,#27388));
#4451=EDGE_LOOP('',(#27389,#27390,#27391,#27392));
#4452=EDGE_LOOP('',(#27393,#27394,#27395,#27396));
#4453=EDGE_LOOP('',(#27397,#27398,#27399,#27400));
#4454=EDGE_LOOP('',(#27401,#27402,#27403,#27404));
#4455=EDGE_LOOP('',(#27405,#27406,#27407,#27408));
#4456=EDGE_LOOP('',(#27409,#27410,#27411,#27412));
#4457=EDGE_LOOP('',(#27413,#27414,#27415,#27416));
#4458=EDGE_LOOP('',(#27417,#27418,#27419,#27420));
#4459=EDGE_LOOP('',(#27421,#27422,#27423,#27424));
#4460=EDGE_LOOP('',(#27425,#27426,#27427,#27428));
#4461=EDGE_LOOP('',(#27429,#27430,#27431,#27432));
#4462=EDGE_LOOP('',(#27433,#27434,#27435,#27436));
#4463=EDGE_LOOP('',(#27437,#27438,#27439,#27440));
#4464=EDGE_LOOP('',(#27441,#27442,#27443,#27444));
#4465=EDGE_LOOP('',(#27445,#27446,#27447,#27448));
#4466=EDGE_LOOP('',(#27449,#27450,#27451,#27452));
#4467=EDGE_LOOP('',(#27453,#27454,#27455,#27456));
#4468=EDGE_LOOP('',(#27457,#27458,#27459,#27460));
#4469=EDGE_LOOP('',(#27461,#27462,#27463,#27464));
#4470=EDGE_LOOP('',(#27465,#27466,#27467,#27468));
#4471=EDGE_LOOP('',(#27469,#27470,#27471,#27472));
#4472=EDGE_LOOP('',(#27473,#27474,#27475,#27476));
#4473=EDGE_LOOP('',(#27477,#27478,#27479,#27480));
#4474=EDGE_LOOP('',(#27481,#27482,#27483,#27484));
#4475=EDGE_LOOP('',(#27485,#27486,#27487,#27488));
#4476=EDGE_LOOP('',(#27489,#27490,#27491,#27492));
#4477=EDGE_LOOP('',(#27493,#27494,#27495,#27496));
#4478=EDGE_LOOP('',(#27497));
#4479=EDGE_LOOP('',(#27498,#27499,#27500,#27501,#27502,#27503,#27504,#27505,
#27506,#27507));
#4480=EDGE_LOOP('',(#27508,#27509,#27510,#27511,#27512,#27513,#27514,#27515,
#27516,#27517));
#4481=EDGE_LOOP('',(#27518,#27519,#27520,#27521,#27522,#27523,#27524,#27525));
#4482=EDGE_LOOP('',(#27526,#27527,#27528,#27529,#27530,#27531,#27532,#27533));
#4483=EDGE_LOOP('',(#27534,#27535,#27536,#27537,#27538,#27539,#27540,#27541));
#4484=EDGE_LOOP('',(#27542,#27543,#27544,#27545,#27546,#27547,#27548,#27549));
#4485=EDGE_LOOP('',(#27550,#27551,#27552,#27553,#27554,#27555,#27556,#27557));
#4486=EDGE_LOOP('',(#27558,#27559,#27560,#27561,#27562,#27563,#27564,#27565));
#4487=EDGE_LOOP('',(#27566,#27567,#27568,#27569,#27570,#27571,#27572,#27573));
#4488=EDGE_LOOP('',(#27574,#27575,#27576,#27577,#27578,#27579,#27580,#27581));
#4489=EDGE_LOOP('',(#27582,#27583,#27584,#27585,#27586,#27587,#27588,#27589));
#4490=EDGE_LOOP('',(#27590,#27591,#27592,#27593,#27594,#27595,#27596,#27597));
#4491=EDGE_LOOP('',(#27598,#27599,#27600,#27601,#27602,#27603,#27604,#27605));
#4492=EDGE_LOOP('',(#27606,#27607,#27608,#27609,#27610,#27611,#27612,#27613));
#4493=EDGE_LOOP('',(#27614,#27615,#27616,#27617,#27618,#27619,#27620,#27621));
#4494=EDGE_LOOP('',(#27622,#27623,#27624,#27625,#27626,#27627,#27628,#27629));
#4495=EDGE_LOOP('',(#27630,#27631,#27632,#27633,#27634,#27635,#27636,#27637));
#4496=EDGE_LOOP('',(#27638,#27639,#27640,#27641,#27642,#27643,#27644,#27645,
#27646,#27647));
#4497=EDGE_LOOP('',(#27648,#27649,#27650,#27651));
#4498=EDGE_LOOP('',(#27652,#27653,#27654,#27655));
#4499=EDGE_LOOP('',(#27656,#27657,#27658,#27659));
#4500=EDGE_LOOP('',(#27660,#27661,#27662,#27663));
#4501=EDGE_LOOP('',(#27664,#27665,#27666,#27667));
#4502=EDGE_LOOP('',(#27668,#27669,#27670,#27671,#27672,#27673,#27674,#27675,
#27676,#27677));
#4503=EDGE_LOOP('',(#27678));
#4504=EDGE_LOOP('',(#27679));
#4505=EDGE_LOOP('',(#27680));
#4506=EDGE_LOOP('',(#27681));
#4507=EDGE_LOOP('',(#27682));
#4508=EDGE_LOOP('',(#27683));
#4509=EDGE_LOOP('',(#27684,#27685,#27686,#27687));
#4510=EDGE_LOOP('',(#27688,#27689,#27690,#27691,#27692,#27693,#27694,#27695,
#27696,#27697,#27698,#27699));
#4511=EDGE_LOOP('',(#27700));
#4512=EDGE_LOOP('',(#27701));
#4513=EDGE_LOOP('',(#27702));
#4514=EDGE_LOOP('',(#27703,#27704,#27705,#27706,#27707,#27708,#27709,#27710,
#27711,#27712));
#4515=EDGE_LOOP('',(#27713));
#4516=EDGE_LOOP('',(#27714));
#4517=EDGE_LOOP('',(#27715));
#4518=EDGE_LOOP('',(#27716));
#4519=EDGE_LOOP('',(#27717));
#4520=EDGE_LOOP('',(#27718));
#4521=EDGE_LOOP('',(#27719,#27720,#27721,#27722));
#4522=EDGE_LOOP('',(#27723,#27724,#27725,#27726,#27727,#27728,#27729,#27730,
#27731,#27732,#27733,#27734));
#4523=EDGE_LOOP('',(#27735));
#4524=EDGE_LOOP('',(#27736));
#4525=EDGE_LOOP('',(#27737));
#4526=EDGE_LOOP('',(#27738,#27739,#27740,#27741,#27742));
#4527=EDGE_LOOP('',(#27743,#27744,#27745,#27746));
#4528=EDGE_LOOP('',(#27747,#27748,#27749,#27750,#27751));
#4529=EDGE_LOOP('',(#27752,#27753,#27754,#27755));
#4530=EDGE_LOOP('',(#27756,#27757,#27758,#27759,#27760));
#4531=EDGE_LOOP('',(#27761,#27762,#27763,#27764));
#4532=EDGE_LOOP('',(#27765,#27766,#27767,#27768,#27769));
#4533=EDGE_LOOP('',(#27770,#27771,#27772,#27773));
#4534=EDGE_LOOP('',(#27774,#27775,#27776,#27777,#27778,#27779));
#4535=EDGE_LOOP('',(#27780,#27781,#27782,#27783,#27784,#27785));
#4536=EDGE_LOOP('',(#27786,#27787,#27788,#27789));
#4537=EDGE_LOOP('',(#27790,#27791,#27792,#27793));
#4538=EDGE_LOOP('',(#27794,#27795,#27796,#27797));
#4539=EDGE_LOOP('',(#27798,#27799,#27800,#27801));
#4540=EDGE_LOOP('',(#27802,#27803,#27804,#27805));
#4541=EDGE_LOOP('',(#27806,#27807,#27808,#27809));
#4542=EDGE_LOOP('',(#27810,#27811,#27812,#27813));
#4543=EDGE_LOOP('',(#27814,#27815,#27816,#27817,#27818));
#4544=EDGE_LOOP('',(#27819,#27820,#27821,#27822,#27823));
#4545=EDGE_LOOP('',(#27824,#27825,#27826,#27827,#27828,#27829));
#4546=EDGE_LOOP('',(#27830,#27831,#27832,#27833,#27834,#27835));
#4547=EDGE_LOOP('',(#27836,#27837,#27838,#27839));
#4548=EDGE_LOOP('',(#27840,#27841,#27842,#27843));
#4549=EDGE_LOOP('',(#27844,#27845,#27846,#27847));
#4550=EDGE_LOOP('',(#27848,#27849,#27850,#27851));
#4551=EDGE_LOOP('',(#27852,#27853,#27854,#27855));
#4552=EDGE_LOOP('',(#27856,#27857,#27858,#27859));
#4553=EDGE_LOOP('',(#27860,#27861,#27862,#27863));
#4554=EDGE_LOOP('',(#27864,#27865,#27866,#27867,#27868));
#4555=EDGE_LOOP('',(#27869,#27870,#27871,#27872,#27873));
#4556=EDGE_LOOP('',(#27874,#27875,#27876,#27877));
#4557=EDGE_LOOP('',(#27878,#27879,#27880,#27881));
#4558=EDGE_LOOP('',(#27882,#27883,#27884,#27885,#27886,#27887));
#4559=EDGE_LOOP('',(#27888,#27889,#27890,#27891,#27892,#27893));
#4560=EDGE_LOOP('',(#27894,#27895,#27896,#27897,#27898,#27899,#27900,#27901,
#27902,#27903,#27904,#27905,#27906,#27907,#27908,#27909));
#4561=EDGE_LOOP('',(#27910,#27911,#27912,#27913,#27914,#27915,#27916,#27917,
#27918,#27919,#27920,#27921,#27922,#27923,#27924,#27925));
#4562=EDGE_LOOP('',(#27926,#27927,#27928,#27929));
#4563=EDGE_LOOP('',(#27930,#27931,#27932,#27933));
#4564=EDGE_LOOP('',(#27934,#27935,#27936,#27937));
#4565=EDGE_LOOP('',(#27938,#27939,#27940,#27941));
#4566=EDGE_LOOP('',(#27942,#27943,#27944,#27945));
#4567=EDGE_LOOP('',(#27946));
#4568=EDGE_LOOP('',(#27947,#27948,#27949,#27950));
#4569=EDGE_LOOP('',(#27951,#27952,#27953,#27954));
#4570=EDGE_LOOP('',(#27955,#27956,#27957,#27958));
#4571=EDGE_LOOP('',(#27959,#27960,#27961,#27962));
#4572=EDGE_LOOP('',(#27963,#27964,#27965,#27966));
#4573=EDGE_LOOP('',(#27967,#27968,#27969,#27970));
#4574=EDGE_LOOP('',(#27971,#27972,#27973,#27974));
#4575=EDGE_LOOP('',(#27975));
#4576=EDGE_LOOP('',(#27976,#27977,#27978,#27979));
#4577=EDGE_LOOP('',(#27980,#27981,#27982,#27983));
#4578=EDGE_LOOP('',(#27984,#27985,#27986,#27987,#27988,#27989));
#4579=EDGE_LOOP('',(#27990,#27991,#27992,#27993,#27994,#27995));
#4580=EDGE_LOOP('',(#27996,#27997,#27998,#27999,#28000,#28001,#28002,#28003,
#28004,#28005,#28006,#28007,#28008,#28009,#28010,#28011));
#4581=EDGE_LOOP('',(#28012,#28013,#28014,#28015,#28016,#28017,#28018,#28019,
#28020,#28021,#28022,#28023,#28024,#28025,#28026,#28027));
#4582=EDGE_LOOP('',(#28028,#28029,#28030,#28031));
#4583=EDGE_LOOP('',(#28032,#28033,#28034,#28035));
#4584=EDGE_LOOP('',(#28036,#28037,#28038,#28039));
#4585=EDGE_LOOP('',(#28040,#28041,#28042,#28043));
#4586=EDGE_LOOP('',(#28044,#28045,#28046,#28047));
#4587=EDGE_LOOP('',(#28048));
#4588=EDGE_LOOP('',(#28049,#28050,#28051,#28052));
#4589=EDGE_LOOP('',(#28053,#28054,#28055,#28056));
#4590=EDGE_LOOP('',(#28057,#28058,#28059,#28060));
#4591=EDGE_LOOP('',(#28061,#28062,#28063,#28064));
#4592=EDGE_LOOP('',(#28065,#28066,#28067,#28068));
#4593=EDGE_LOOP('',(#28069,#28070,#28071,#28072));
#4594=EDGE_LOOP('',(#28073,#28074,#28075,#28076));
#4595=EDGE_LOOP('',(#28077));
#4596=EDGE_LOOP('',(#28078,#28079,#28080,#28081));
#4597=EDGE_LOOP('',(#28082,#28083,#28084,#28085));
#4598=EDGE_LOOP('',(#28086,#28087,#28088,#28089,#28090,#28091));
#4599=EDGE_LOOP('',(#28092,#28093,#28094,#28095,#28096,#28097));
#4600=EDGE_LOOP('',(#28098,#28099,#28100,#28101,#28102,#28103,#28104,#28105,
#28106,#28107,#28108,#28109,#28110,#28111,#28112,#28113));
#4601=EDGE_LOOP('',(#28114,#28115,#28116,#28117,#28118,#28119,#28120,#28121,
#28122,#28123,#28124,#28125,#28126,#28127,#28128,#28129));
#4602=EDGE_LOOP('',(#28130,#28131,#28132,#28133));
#4603=EDGE_LOOP('',(#28134,#28135,#28136,#28137));
#4604=EDGE_LOOP('',(#28138,#28139,#28140,#28141));
#4605=EDGE_LOOP('',(#28142,#28143,#28144,#28145));
#4606=EDGE_LOOP('',(#28146,#28147,#28148,#28149));
#4607=EDGE_LOOP('',(#28150));
#4608=EDGE_LOOP('',(#28151,#28152,#28153,#28154));
#4609=EDGE_LOOP('',(#28155,#28156,#28157,#28158));
#4610=EDGE_LOOP('',(#28159,#28160,#28161,#28162));
#4611=EDGE_LOOP('',(#28163,#28164,#28165,#28166));
#4612=EDGE_LOOP('',(#28167,#28168,#28169,#28170));
#4613=EDGE_LOOP('',(#28171,#28172,#28173,#28174));
#4614=EDGE_LOOP('',(#28175,#28176,#28177,#28178));
#4615=EDGE_LOOP('',(#28179));
#4616=EDGE_LOOP('',(#28180,#28181,#28182,#28183));
#4617=EDGE_LOOP('',(#28184,#28185,#28186,#28187));
#4618=EDGE_LOOP('',(#28188,#28189,#28190,#28191,#28192,#28193));
#4619=EDGE_LOOP('',(#28194,#28195,#28196,#28197,#28198,#28199));
#4620=EDGE_LOOP('',(#28200,#28201,#28202,#28203,#28204,#28205,#28206,#28207,
#28208,#28209,#28210,#28211,#28212,#28213,#28214,#28215));
#4621=EDGE_LOOP('',(#28216,#28217,#28218,#28219,#28220,#28221,#28222,#28223,
#28224,#28225,#28226,#28227,#28228,#28229,#28230,#28231));
#4622=EDGE_LOOP('',(#28232,#28233,#28234,#28235));
#4623=EDGE_LOOP('',(#28236,#28237,#28238,#28239));
#4624=EDGE_LOOP('',(#28240,#28241,#28242,#28243));
#4625=EDGE_LOOP('',(#28244,#28245,#28246,#28247));
#4626=EDGE_LOOP('',(#28248,#28249,#28250,#28251));
#4627=EDGE_LOOP('',(#28252));
#4628=EDGE_LOOP('',(#28253,#28254,#28255,#28256));
#4629=EDGE_LOOP('',(#28257,#28258,#28259,#28260));
#4630=EDGE_LOOP('',(#28261,#28262,#28263,#28264));
#4631=EDGE_LOOP('',(#28265,#28266,#28267,#28268));
#4632=EDGE_LOOP('',(#28269,#28270,#28271,#28272));
#4633=EDGE_LOOP('',(#28273,#28274,#28275,#28276));
#4634=EDGE_LOOP('',(#28277,#28278,#28279,#28280));
#4635=EDGE_LOOP('',(#28281));
#4636=EDGE_LOOP('',(#28282));
#4637=EDGE_LOOP('',(#28283,#28284,#28285,#28286,#28287,#28288,#28289,#28290,
#28291,#28292));
#4638=EDGE_LOOP('',(#28293,#28294,#28295,#28296,#28297,#28298,#28299,#28300));
#4639=EDGE_LOOP('',(#28301,#28302,#28303,#28304,#28305,#28306,#28307,#28308));
#4640=EDGE_LOOP('',(#28309,#28310,#28311,#28312,#28313,#28314,#28315,#28316));
#4641=EDGE_LOOP('',(#28317,#28318,#28319,#28320,#28321,#28322,#28323,#28324));
#4642=EDGE_LOOP('',(#28325,#28326,#28327,#28328,#28329,#28330,#28331,#28332));
#4643=EDGE_LOOP('',(#28333,#28334,#28335,#28336,#28337,#28338,#28339,#28340,
#28341,#28342));
#4644=EDGE_LOOP('',(#28343,#28344,#28345,#28346,#28347,#28348,#28349,#28350));
#4645=EDGE_LOOP('',(#28351,#28352,#28353,#28354,#28355,#28356,#28357,#28358));
#4646=EDGE_LOOP('',(#28359,#28360,#28361,#28362,#28363,#28364,#28365,#28366));
#4647=EDGE_LOOP('',(#28367,#28368,#28369,#28370,#28371,#28372,#28373,#28374));
#4648=EDGE_LOOP('',(#28375,#28376,#28377,#28378,#28379,#28380,#28381,#28382));
#4649=EDGE_LOOP('',(#28383,#28384,#28385,#28386,#28387,#28388,#28389,#28390,
#28391,#28392));
#4650=EDGE_LOOP('',(#28393,#28394,#28395,#28396,#28397,#28398,#28399,#28400));
#4651=EDGE_LOOP('',(#28401,#28402,#28403,#28404,#28405,#28406,#28407,#28408));
#4652=EDGE_LOOP('',(#28409,#28410,#28411,#28412,#28413,#28414,#28415,#28416));
#4653=EDGE_LOOP('',(#28417,#28418,#28419,#28420,#28421,#28422,#28423,#28424));
#4654=EDGE_LOOP('',(#28425,#28426,#28427,#28428,#28429,#28430,#28431,#28432));
#4655=EDGE_LOOP('',(#28433,#28434,#28435,#28436));
#4656=EDGE_LOOP('',(#28437,#28438,#28439,#28440));
#4657=EDGE_LOOP('',(#28441,#28442,#28443,#28444));
#4658=EDGE_LOOP('',(#28445,#28446,#28447,#28448));
#4659=EDGE_LOOP('',(#28449,#28450,#28451,#28452));
#4660=EDGE_LOOP('',(#28453,#28454,#28455,#28456));
#4661=EDGE_LOOP('',(#28457,#28458,#28459,#28460));
#4662=EDGE_LOOP('',(#28461,#28462,#28463,#28464));
#4663=EDGE_LOOP('',(#28465,#28466,#28467,#28468));
#4664=EDGE_LOOP('',(#28469,#28470,#28471,#28472));
#4665=EDGE_LOOP('',(#28473,#28474,#28475,#28476));
#4666=EDGE_LOOP('',(#28477,#28478,#28479,#28480));
#4667=EDGE_LOOP('',(#28481,#28482,#28483,#28484));
#4668=EDGE_LOOP('',(#28485,#28486,#28487,#28488));
#4669=EDGE_LOOP('',(#28489,#28490,#28491,#28492));
#4670=EDGE_LOOP('',(#28493,#28494,#28495,#28496));
#4671=EDGE_LOOP('',(#28497,#28498,#28499,#28500));
#4672=EDGE_LOOP('',(#28501,#28502,#28503,#28504));
#4673=EDGE_LOOP('',(#28505,#28506,#28507,#28508));
#4674=EDGE_LOOP('',(#28509,#28510,#28511,#28512));
#4675=EDGE_LOOP('',(#28513,#28514,#28515,#28516));
#4676=EDGE_LOOP('',(#28517,#28518,#28519,#28520));
#4677=EDGE_LOOP('',(#28521,#28522,#28523,#28524));
#4678=EDGE_LOOP('',(#28525,#28526,#28527,#28528));
#4679=EDGE_LOOP('',(#28529,#28530,#28531,#28532));
#4680=EDGE_LOOP('',(#28533,#28534,#28535,#28536));
#4681=EDGE_LOOP('',(#28537,#28538,#28539,#28540));
#4682=EDGE_LOOP('',(#28541,#28542,#28543,#28544));
#4683=EDGE_LOOP('',(#28545,#28546,#28547,#28548));
#4684=EDGE_LOOP('',(#28549,#28550,#28551,#28552));
#4685=EDGE_LOOP('',(#28553,#28554,#28555,#28556));
#4686=EDGE_LOOP('',(#28557,#28558,#28559,#28560));
#4687=EDGE_LOOP('',(#28561,#28562,#28563,#28564));
#4688=EDGE_LOOP('',(#28565,#28566,#28567,#28568));
#4689=EDGE_LOOP('',(#28569,#28570,#28571,#28572));
#4690=EDGE_LOOP('',(#28573,#28574,#28575,#28576));
#4691=EDGE_LOOP('',(#28577,#28578,#28579,#28580));
#4692=EDGE_LOOP('',(#28581,#28582,#28583,#28584));
#4693=EDGE_LOOP('',(#28585,#28586,#28587,#28588));
#4694=EDGE_LOOP('',(#28589,#28590,#28591,#28592));
#4695=EDGE_LOOP('',(#28593,#28594,#28595,#28596));
#4696=EDGE_LOOP('',(#28597,#28598,#28599,#28600));
#4697=EDGE_LOOP('',(#28601,#28602,#28603,#28604));
#4698=EDGE_LOOP('',(#28605,#28606,#28607,#28608));
#4699=EDGE_LOOP('',(#28609,#28610,#28611,#28612));
#4700=EDGE_LOOP('',(#28613,#28614,#28615,#28616));
#4701=EDGE_LOOP('',(#28617,#28618,#28619,#28620));
#4702=EDGE_LOOP('',(#28621,#28622,#28623,#28624));
#4703=EDGE_LOOP('',(#28625,#28626,#28627,#28628));
#4704=EDGE_LOOP('',(#28629,#28630,#28631,#28632));
#4705=EDGE_LOOP('',(#28633,#28634,#28635,#28636));
#4706=EDGE_LOOP('',(#28637,#28638,#28639,#28640));
#4707=EDGE_LOOP('',(#28641,#28642,#28643,#28644));
#4708=EDGE_LOOP('',(#28645,#28646,#28647,#28648));
#4709=EDGE_LOOP('',(#28649,#28650,#28651,#28652));
#4710=EDGE_LOOP('',(#28653,#28654,#28655,#28656));
#4711=EDGE_LOOP('',(#28657,#28658,#28659,#28660));
#4712=EDGE_LOOP('',(#28661,#28662,#28663,#28664));
#4713=EDGE_LOOP('',(#28665,#28666,#28667,#28668));
#4714=EDGE_LOOP('',(#28669,#28670,#28671,#28672));
#4715=EDGE_LOOP('',(#28673,#28674,#28675,#28676));
#4716=EDGE_LOOP('',(#28677,#28678,#28679,#28680));
#4717=EDGE_LOOP('',(#28681,#28682,#28683,#28684));
#4718=EDGE_LOOP('',(#28685,#28686,#28687,#28688));
#4719=EDGE_LOOP('',(#28689,#28690,#28691,#28692));
#4720=EDGE_LOOP('',(#28693,#28694,#28695,#28696));
#4721=EDGE_LOOP('',(#28697,#28698,#28699,#28700));
#4722=EDGE_LOOP('',(#28701,#28702,#28703,#28704));
#4723=EDGE_LOOP('',(#28705,#28706,#28707,#28708));
#4724=EDGE_LOOP('',(#28709,#28710,#28711,#28712));
#4725=EDGE_LOOP('',(#28713,#28714,#28715,#28716));
#4726=EDGE_LOOP('',(#28717,#28718,#28719,#28720));
#4727=EDGE_LOOP('',(#28721,#28722,#28723,#28724));
#4728=EDGE_LOOP('',(#28725,#28726,#28727,#28728));
#4729=EDGE_LOOP('',(#28729,#28730,#28731,#28732));
#4730=EDGE_LOOP('',(#28733,#28734,#28735,#28736));
#4731=EDGE_LOOP('',(#28737,#28738,#28739,#28740));
#4732=EDGE_LOOP('',(#28741,#28742,#28743,#28744));
#4733=EDGE_LOOP('',(#28745,#28746,#28747,#28748));
#4734=EDGE_LOOP('',(#28749,#28750,#28751,#28752));
#4735=EDGE_LOOP('',(#28753,#28754,#28755,#28756));
#4736=EDGE_LOOP('',(#28757,#28758,#28759,#28760));
#4737=EDGE_LOOP('',(#28761,#28762,#28763,#28764));
#4738=EDGE_LOOP('',(#28765,#28766,#28767,#28768));
#4739=EDGE_LOOP('',(#28769,#28770,#28771,#28772));
#4740=EDGE_LOOP('',(#28773,#28774,#28775,#28776));
#4741=EDGE_LOOP('',(#28777,#28778,#28779,#28780));
#4742=EDGE_LOOP('',(#28781,#28782,#28783,#28784));
#4743=EDGE_LOOP('',(#28785,#28786,#28787,#28788));
#4744=EDGE_LOOP('',(#28789,#28790,#28791,#28792));
#4745=EDGE_LOOP('',(#28793,#28794,#28795,#28796));
#4746=EDGE_LOOP('',(#28797,#28798,#28799,#28800));
#4747=EDGE_LOOP('',(#28801,#28802,#28803,#28804));
#4748=EDGE_LOOP('',(#28805,#28806,#28807,#28808));
#4749=EDGE_LOOP('',(#28809,#28810,#28811,#28812));
#4750=EDGE_LOOP('',(#28813,#28814,#28815,#28816));
#4751=EDGE_LOOP('',(#28817,#28818,#28819,#28820));
#4752=EDGE_LOOP('',(#28821,#28822,#28823,#28824));
#4753=EDGE_LOOP('',(#28825,#28826,#28827,#28828));
#4754=EDGE_LOOP('',(#28829,#28830,#28831,#28832));
#4755=EDGE_LOOP('',(#28833,#28834,#28835,#28836));
#4756=EDGE_LOOP('',(#28837,#28838,#28839,#28840));
#4757=EDGE_LOOP('',(#28841,#28842,#28843,#28844));
#4758=EDGE_LOOP('',(#28845,#28846,#28847,#28848));
#4759=EDGE_LOOP('',(#28849,#28850,#28851,#28852));
#4760=EDGE_LOOP('',(#28853,#28854,#28855,#28856));
#4761=EDGE_LOOP('',(#28857,#28858,#28859,#28860));
#4762=EDGE_LOOP('',(#28861,#28862,#28863,#28864));
#4763=EDGE_LOOP('',(#28865,#28866,#28867,#28868));
#4764=EDGE_LOOP('',(#28869,#28870,#28871,#28872));
#4765=EDGE_LOOP('',(#28873,#28874,#28875,#28876));
#4766=EDGE_LOOP('',(#28877,#28878,#28879,#28880));
#4767=EDGE_LOOP('',(#28881,#28882,#28883,#28884));
#4768=EDGE_LOOP('',(#28885,#28886,#28887,#28888));
#4769=EDGE_LOOP('',(#28889,#28890,#28891,#28892));
#4770=EDGE_LOOP('',(#28893,#28894,#28895,#28896));
#4771=EDGE_LOOP('',(#28897,#28898,#28899,#28900));
#4772=EDGE_LOOP('',(#28901,#28902,#28903,#28904));
#4773=EDGE_LOOP('',(#28905,#28906,#28907,#28908));
#4774=EDGE_LOOP('',(#28909,#28910,#28911,#28912));
#4775=EDGE_LOOP('',(#28913,#28914,#28915,#28916));
#4776=EDGE_LOOP('',(#28917,#28918,#28919,#28920));
#4777=EDGE_LOOP('',(#28921,#28922,#28923,#28924));
#4778=EDGE_LOOP('',(#28925,#28926,#28927,#28928));
#4779=EDGE_LOOP('',(#28929,#28930,#28931,#28932));
#4780=EDGE_LOOP('',(#28933,#28934,#28935,#28936));
#4781=EDGE_LOOP('',(#28937,#28938,#28939,#28940));
#4782=EDGE_LOOP('',(#28941,#28942,#28943,#28944));
#4783=EDGE_LOOP('',(#28945,#28946,#28947,#28948));
#4784=EDGE_LOOP('',(#28949,#28950,#28951,#28952));
#4785=EDGE_LOOP('',(#28953,#28954,#28955,#28956));
#4786=EDGE_LOOP('',(#28957,#28958,#28959,#28960));
#4787=EDGE_LOOP('',(#28961,#28962,#28963,#28964));
#4788=EDGE_LOOP('',(#28965,#28966,#28967,#28968));
#4789=EDGE_LOOP('',(#28969,#28970,#28971,#28972));
#4790=EDGE_LOOP('',(#28973,#28974,#28975,#28976));
#4791=EDGE_LOOP('',(#28977,#28978,#28979,#28980));
#4792=EDGE_LOOP('',(#28981,#28982,#28983,#28984));
#4793=EDGE_LOOP('',(#28985,#28986,#28987,#28988));
#4794=EDGE_LOOP('',(#28989,#28990,#28991,#28992));
#4795=EDGE_LOOP('',(#28993,#28994,#28995,#28996));
#4796=EDGE_LOOP('',(#28997,#28998,#28999,#29000));
#4797=EDGE_LOOP('',(#29001,#29002,#29003,#29004));
#4798=EDGE_LOOP('',(#29005,#29006,#29007,#29008));
#4799=EDGE_LOOP('',(#29009,#29010,#29011,#29012));
#4800=EDGE_LOOP('',(#29013,#29014,#29015,#29016));
#4801=EDGE_LOOP('',(#29017,#29018,#29019,#29020));
#4802=EDGE_LOOP('',(#29021,#29022,#29023,#29024));
#4803=EDGE_LOOP('',(#29025,#29026,#29027,#29028));
#4804=EDGE_LOOP('',(#29029,#29030,#29031,#29032));
#4805=EDGE_LOOP('',(#29033,#29034,#29035,#29036));
#4806=EDGE_LOOP('',(#29037,#29038,#29039,#29040));
#4807=EDGE_LOOP('',(#29041,#29042,#29043,#29044));
#4808=EDGE_LOOP('',(#29045,#29046,#29047,#29048));
#4809=EDGE_LOOP('',(#29049,#29050,#29051,#29052));
#4810=EDGE_LOOP('',(#29053,#29054,#29055,#29056));
#4811=EDGE_LOOP('',(#29057,#29058,#29059,#29060));
#4812=EDGE_LOOP('',(#29061,#29062,#29063,#29064));
#4813=EDGE_LOOP('',(#29065,#29066,#29067,#29068));
#4814=EDGE_LOOP('',(#29069,#29070,#29071,#29072));
#4815=EDGE_LOOP('',(#29073,#29074,#29075,#29076));
#4816=EDGE_LOOP('',(#29077,#29078,#29079,#29080));
#4817=EDGE_LOOP('',(#29081,#29082,#29083,#29084));
#4818=EDGE_LOOP('',(#29085,#29086,#29087,#29088));
#4819=EDGE_LOOP('',(#29089,#29090,#29091,#29092));
#4820=EDGE_LOOP('',(#29093,#29094,#29095,#29096));
#4821=EDGE_LOOP('',(#29097,#29098,#29099,#29100));
#4822=EDGE_LOOP('',(#29101,#29102,#29103,#29104));
#4823=EDGE_LOOP('',(#29105,#29106,#29107,#29108));
#4824=EDGE_LOOP('',(#29109,#29110,#29111,#29112));
#4825=EDGE_LOOP('',(#29113,#29114,#29115,#29116));
#4826=EDGE_LOOP('',(#29117,#29118,#29119,#29120));
#4827=EDGE_LOOP('',(#29121,#29122,#29123,#29124));
#4828=EDGE_LOOP('',(#29125,#29126,#29127,#29128));
#4829=EDGE_LOOP('',(#29129,#29130,#29131,#29132));
#4830=EDGE_LOOP('',(#29133,#29134,#29135,#29136));
#4831=EDGE_LOOP('',(#29137,#29138,#29139,#29140));
#4832=EDGE_LOOP('',(#29141,#29142,#29143,#29144));
#4833=EDGE_LOOP('',(#29145,#29146,#29147,#29148));
#4834=EDGE_LOOP('',(#29149,#29150,#29151,#29152));
#4835=EDGE_LOOP('',(#29153,#29154,#29155,#29156));
#4836=EDGE_LOOP('',(#29157,#29158,#29159,#29160));
#4837=EDGE_LOOP('',(#29161,#29162,#29163,#29164));
#4838=EDGE_LOOP('',(#29165,#29166,#29167,#29168));
#4839=EDGE_LOOP('',(#29169,#29170,#29171,#29172));
#4840=EDGE_LOOP('',(#29173,#29174,#29175,#29176));
#4841=EDGE_LOOP('',(#29177,#29178,#29179,#29180));
#4842=EDGE_LOOP('',(#29181,#29182,#29183,#29184));
#4843=EDGE_LOOP('',(#29185,#29186,#29187,#29188));
#4844=EDGE_LOOP('',(#29189,#29190,#29191,#29192));
#4845=EDGE_LOOP('',(#29193,#29194,#29195,#29196));
#4846=EDGE_LOOP('',(#29197,#29198,#29199,#29200));
#4847=EDGE_LOOP('',(#29201,#29202,#29203,#29204));
#4848=EDGE_LOOP('',(#29205,#29206,#29207,#29208));
#4849=EDGE_LOOP('',(#29209,#29210,#29211,#29212));
#4850=EDGE_LOOP('',(#29213,#29214,#29215,#29216));
#4851=EDGE_LOOP('',(#29217,#29218,#29219,#29220));
#4852=EDGE_LOOP('',(#29221,#29222,#29223,#29224));
#4853=EDGE_LOOP('',(#29225,#29226,#29227,#29228));
#4854=EDGE_LOOP('',(#29229,#29230,#29231,#29232));
#4855=EDGE_LOOP('',(#29233,#29234,#29235,#29236));
#4856=EDGE_LOOP('',(#29237,#29238,#29239,#29240));
#4857=EDGE_LOOP('',(#29241,#29242,#29243,#29244));
#4858=EDGE_LOOP('',(#29245,#29246,#29247,#29248));
#4859=EDGE_LOOP('',(#29249,#29250,#29251,#29252));
#4860=EDGE_LOOP('',(#29253,#29254,#29255,#29256));
#4861=EDGE_LOOP('',(#29257,#29258,#29259,#29260));
#4862=EDGE_LOOP('',(#29261,#29262,#29263,#29264));
#4863=EDGE_LOOP('',(#29265,#29266,#29267,#29268));
#4864=EDGE_LOOP('',(#29269,#29270,#29271,#29272));
#4865=EDGE_LOOP('',(#29273,#29274,#29275,#29276));
#4866=EDGE_LOOP('',(#29277,#29278,#29279,#29280));
#4867=EDGE_LOOP('',(#29281,#29282,#29283,#29284));
#4868=EDGE_LOOP('',(#29285,#29286,#29287,#29288));
#4869=EDGE_LOOP('',(#29289,#29290,#29291,#29292));
#4870=EDGE_LOOP('',(#29293,#29294,#29295,#29296));
#4871=EDGE_LOOP('',(#29297,#29298,#29299,#29300));
#4872=EDGE_LOOP('',(#29301,#29302,#29303,#29304));
#4873=EDGE_LOOP('',(#29305,#29306,#29307,#29308));
#4874=EDGE_LOOP('',(#29309,#29310,#29311,#29312));
#4875=EDGE_LOOP('',(#29313,#29314,#29315,#29316));
#4876=EDGE_LOOP('',(#29317,#29318,#29319,#29320));
#4877=EDGE_LOOP('',(#29321,#29322,#29323,#29324));
#4878=EDGE_LOOP('',(#29325,#29326,#29327,#29328));
#4879=EDGE_LOOP('',(#29329,#29330,#29331,#29332));
#4880=EDGE_LOOP('',(#29333,#29334,#29335,#29336));
#4881=EDGE_LOOP('',(#29337,#29338,#29339,#29340));
#4882=EDGE_LOOP('',(#29341,#29342,#29343,#29344));
#4883=EDGE_LOOP('',(#29345,#29346,#29347,#29348));
#4884=EDGE_LOOP('',(#29349,#29350,#29351,#29352));
#4885=EDGE_LOOP('',(#29353,#29354,#29355,#29356));
#4886=EDGE_LOOP('',(#29357,#29358,#29359,#29360));
#4887=EDGE_LOOP('',(#29361,#29362,#29363,#29364));
#4888=EDGE_LOOP('',(#29365,#29366,#29367,#29368));
#4889=EDGE_LOOP('',(#29369,#29370,#29371,#29372));
#4890=EDGE_LOOP('',(#29373,#29374,#29375,#29376));
#4891=EDGE_LOOP('',(#29377,#29378,#29379,#29380));
#4892=EDGE_LOOP('',(#29381,#29382,#29383,#29384));
#4893=EDGE_LOOP('',(#29385,#29386,#29387,#29388));
#4894=EDGE_LOOP('',(#29389,#29390,#29391,#29392));
#4895=EDGE_LOOP('',(#29393,#29394,#29395,#29396));
#4896=EDGE_LOOP('',(#29397,#29398,#29399,#29400));
#4897=EDGE_LOOP('',(#29401,#29402,#29403,#29404));
#4898=EDGE_LOOP('',(#29405,#29406,#29407,#29408));
#4899=EDGE_LOOP('',(#29409,#29410,#29411,#29412));
#4900=EDGE_LOOP('',(#29413,#29414,#29415,#29416));
#4901=EDGE_LOOP('',(#29417,#29418,#29419,#29420));
#4902=EDGE_LOOP('',(#29421,#29422,#29423,#29424));
#4903=EDGE_LOOP('',(#29425,#29426,#29427,#29428));
#4904=EDGE_LOOP('',(#29429,#29430,#29431,#29432));
#4905=EDGE_LOOP('',(#29433,#29434,#29435,#29436));
#4906=EDGE_LOOP('',(#29437,#29438,#29439,#29440));
#4907=EDGE_LOOP('',(#29441,#29442,#29443,#29444));
#4908=EDGE_LOOP('',(#29445,#29446,#29447,#29448));
#4909=EDGE_LOOP('',(#29449,#29450,#29451,#29452));
#4910=EDGE_LOOP('',(#29453,#29454,#29455,#29456));
#4911=EDGE_LOOP('',(#29457,#29458,#29459,#29460));
#4912=EDGE_LOOP('',(#29461,#29462,#29463,#29464));
#4913=EDGE_LOOP('',(#29465,#29466,#29467,#29468));
#4914=EDGE_LOOP('',(#29469,#29470,#29471,#29472));
#4915=EDGE_LOOP('',(#29473,#29474,#29475,#29476));
#4916=EDGE_LOOP('',(#29477,#29478,#29479,#29480));
#4917=EDGE_LOOP('',(#29481,#29482,#29483,#29484));
#4918=EDGE_LOOP('',(#29485,#29486,#29487,#29488));
#4919=EDGE_LOOP('',(#29489,#29490,#29491,#29492));
#4920=EDGE_LOOP('',(#29493,#29494,#29495,#29496));
#4921=EDGE_LOOP('',(#29497,#29498,#29499,#29500));
#4922=EDGE_LOOP('',(#29501,#29502,#29503,#29504));
#4923=EDGE_LOOP('',(#29505,#29506,#29507,#29508));
#4924=EDGE_LOOP('',(#29509,#29510,#29511,#29512));
#4925=EDGE_LOOP('',(#29513,#29514,#29515,#29516));
#4926=EDGE_LOOP('',(#29517,#29518,#29519,#29520));
#4927=EDGE_LOOP('',(#29521,#29522,#29523,#29524));
#4928=EDGE_LOOP('',(#29525,#29526,#29527,#29528));
#4929=EDGE_LOOP('',(#29529,#29530,#29531,#29532));
#4930=EDGE_LOOP('',(#29533,#29534,#29535,#29536));
#4931=EDGE_LOOP('',(#29537,#29538,#29539,#29540));
#4932=EDGE_LOOP('',(#29541,#29542,#29543,#29544,#29545,#29546));
#4933=EDGE_LOOP('',(#29547,#29548,#29549,#29550,#29551,#29552));
#4934=EDGE_LOOP('',(#29553,#29554,#29555,#29556,#29557,#29558,#29559,#29560,
#29561,#29562,#29563,#29564,#29565,#29566,#29567,#29568));
#4935=EDGE_LOOP('',(#29569,#29570,#29571,#29572,#29573,#29574,#29575,#29576,
#29577,#29578,#29579,#29580,#29581,#29582,#29583,#29584));
#4936=EDGE_LOOP('',(#29585,#29586,#29587,#29588));
#4937=EDGE_LOOP('',(#29589,#29590,#29591,#29592));
#4938=EDGE_LOOP('',(#29593,#29594,#29595,#29596));
#4939=EDGE_LOOP('',(#29597,#29598,#29599,#29600));
#4940=EDGE_LOOP('',(#29601,#29602,#29603,#29604));
#4941=EDGE_LOOP('',(#29605));
#4942=EDGE_LOOP('',(#29606,#29607,#29608,#29609));
#4943=EDGE_LOOP('',(#29610,#29611,#29612,#29613));
#4944=EDGE_LOOP('',(#29614,#29615,#29616,#29617));
#4945=EDGE_LOOP('',(#29618,#29619,#29620,#29621));
#4946=EDGE_LOOP('',(#29622,#29623,#29624,#29625));
#4947=EDGE_LOOP('',(#29626,#29627,#29628,#29629));
#4948=EDGE_LOOP('',(#29630,#29631,#29632,#29633));
#4949=EDGE_LOOP('',(#29634));
#4950=EDGE_LOOP('',(#29635,#29636,#29637,#29638));
#4951=EDGE_LOOP('',(#29639,#29640,#29641,#29642));
#4952=EDGE_LOOP('',(#29643,#29644,#29645,#29646,#29647,#29648));
#4953=EDGE_LOOP('',(#29649,#29650,#29651,#29652,#29653,#29654));
#4954=EDGE_LOOP('',(#29655,#29656,#29657,#29658,#29659,#29660,#29661,#29662,
#29663,#29664,#29665,#29666,#29667,#29668,#29669,#29670));
#4955=EDGE_LOOP('',(#29671,#29672,#29673,#29674,#29675,#29676,#29677,#29678,
#29679,#29680,#29681,#29682,#29683,#29684,#29685,#29686));
#4956=EDGE_LOOP('',(#29687,#29688,#29689,#29690));
#4957=EDGE_LOOP('',(#29691,#29692,#29693,#29694));
#4958=EDGE_LOOP('',(#29695,#29696,#29697,#29698));
#4959=EDGE_LOOP('',(#29699,#29700,#29701,#29702));
#4960=EDGE_LOOP('',(#29703,#29704,#29705,#29706));
#4961=EDGE_LOOP('',(#29707));
#4962=EDGE_LOOP('',(#29708,#29709,#29710,#29711));
#4963=EDGE_LOOP('',(#29712,#29713,#29714,#29715));
#4964=EDGE_LOOP('',(#29716,#29717,#29718,#29719));
#4965=EDGE_LOOP('',(#29720,#29721,#29722,#29723));
#4966=EDGE_LOOP('',(#29724,#29725,#29726,#29727));
#4967=EDGE_LOOP('',(#29728,#29729,#29730,#29731));
#4968=EDGE_LOOP('',(#29732,#29733,#29734,#29735));
#4969=EDGE_LOOP('',(#29736));
#4970=EDGE_LOOP('',(#29737,#29738,#29739,#29740));
#4971=EDGE_LOOP('',(#29741,#29742,#29743,#29744));
#4972=EDGE_LOOP('',(#29745,#29746,#29747,#29748));
#4973=EDGE_LOOP('',(#29749,#29750,#29751,#29752));
#4974=EDGE_LOOP('',(#29753,#29754,#29755,#29756));
#4975=EDGE_LOOP('',(#29757,#29758,#29759,#29760));
#4976=EDGE_LOOP('',(#29761,#29762,#29763,#29764));
#4977=EDGE_LOOP('',(#29765,#29766,#29767,#29768));
#4978=EDGE_LOOP('',(#29769,#29770,#29771,#29772));
#4979=EDGE_LOOP('',(#29773,#29774,#29775,#29776));
#4980=EDGE_LOOP('',(#29777,#29778,#29779,#29780));
#4981=EDGE_LOOP('',(#29781,#29782,#29783,#29784));
#4982=EDGE_LOOP('',(#29785,#29786,#29787,#29788,#29789,#29790));
#4983=EDGE_LOOP('',(#29791,#29792,#29793,#29794,#29795,#29796));
#4984=EDGE_LOOP('',(#29797,#29798,#29799,#29800));
#4985=EDGE_LOOP('',(#29801,#29802,#29803,#29804));
#4986=EDGE_LOOP('',(#29805,#29806,#29807,#29808));
#6740=LINE('',#52457,#11615);
#6741=LINE('',#52463,#11616);
#6742=LINE('',#52469,#11617);
#6743=LINE('',#52475,#11618);
#6744=LINE('',#52481,#11619);
#6745=LINE('',#52487,#11620);
#6746=LINE('',#52494,#11621);
#6747=LINE('',#52497,#11622);
#6748=LINE('',#52503,#11623);
#6749=LINE('',#52506,#11624);
#6750=LINE('',#52512,#11625);
#6751=LINE('',#52515,#11626);
#6752=LINE('',#52521,#11627);
#6753=LINE('',#52524,#11628);
#6754=LINE('',#52530,#11629);
#6755=LINE('',#52533,#11630);
#6756=LINE('',#52539,#11631);
#6757=LINE('',#52542,#11632);
#6758=LINE('',#52548,#11633);
#6759=LINE('',#52551,#11634);
#6760=LINE('',#52557,#11635);
#6761=LINE('',#52560,#11636);
#6762=LINE('',#52566,#11637);
#6763=LINE('',#52569,#11638);
#6764=LINE('',#52575,#11639);
#6765=LINE('',#52578,#11640);
#6766=LINE('',#52584,#11641);
#6767=LINE('',#52587,#11642);
#6768=LINE('',#52593,#11643);
#6769=LINE('',#52596,#11644);
#6770=LINE('',#52602,#11645);
#6771=LINE('',#52605,#11646);
#6772=LINE('',#52611,#11647);
#6773=LINE('',#52614,#11648);
#6774=LINE('',#52620,#11649);
#6775=LINE('',#52623,#11650);
#6776=LINE('',#52629,#11651);
#6777=LINE('',#52632,#11652);
#6778=LINE('',#52638,#11653);
#6779=LINE('',#52641,#11654);
#6780=LINE('',#52647,#11655);
#6781=LINE('',#52650,#11656);
#6782=LINE('',#52656,#11657);
#6783=LINE('',#52659,#11658);
#6784=LINE('',#52665,#11659);
#6785=LINE('',#52668,#11660);
#6786=LINE('',#52674,#11661);
#6787=LINE('',#52677,#11662);
#6788=LINE('',#52683,#11663);
#6789=LINE('',#52686,#11664);
#6790=LINE('',#52692,#11665);
#6791=LINE('',#52695,#11666);
#6792=LINE('',#52701,#11667);
#6793=LINE('',#52704,#11668);
#6794=LINE('',#52710,#11669);
#6795=LINE('',#52713,#11670);
#6796=LINE('',#52719,#11671);
#6797=LINE('',#52722,#11672);
#6798=LINE('',#52728,#11673);
#6799=LINE('',#52731,#11674);
#6800=LINE('',#52737,#11675);
#6801=LINE('',#52740,#11676);
#6802=LINE('',#52746,#11677);
#6803=LINE('',#52749,#11678);
#6804=LINE('',#52755,#11679);
#6805=LINE('',#52758,#11680);
#6806=LINE('',#52764,#11681);
#6807=LINE('',#52767,#11682);
#6808=LINE('',#52773,#11683);
#6809=LINE('',#52776,#11684);
#6810=LINE('',#52782,#11685);
#6811=LINE('',#52785,#11686);
#6812=LINE('',#52791,#11687);
#6813=LINE('',#52794,#11688);
#6814=LINE('',#52800,#11689);
#6815=LINE('',#52803,#11690);
#6816=LINE('',#52809,#11691);
#6817=LINE('',#52812,#11692);
#6818=LINE('',#52818,#11693);
#6819=LINE('',#52821,#11694);
#6820=LINE('',#52827,#11695);
#6821=LINE('',#52830,#11696);
#6822=LINE('',#52836,#11697);
#6823=LINE('',#52839,#11698);
#6824=LINE('',#52845,#11699);
#6825=LINE('',#52848,#11700);
#6826=LINE('',#52854,#11701);
#6827=LINE('',#52857,#11702);
#6828=LINE('',#52863,#11703);
#6829=LINE('',#52866,#11704);
#6830=LINE('',#52872,#11705);
#6831=LINE('',#52875,#11706);
#6832=LINE('',#52881,#11707);
#6833=LINE('',#52884,#11708);
#6834=LINE('',#52890,#11709);
#6835=LINE('',#52893,#11710);
#6836=LINE('',#52899,#11711);
#6837=LINE('',#52902,#11712);
#6838=LINE('',#52908,#11713);
#6839=LINE('',#52911,#11714);
#6840=LINE('',#52917,#11715);
#6841=LINE('',#52920,#11716);
#6842=LINE('',#52926,#11717);
#6843=LINE('',#52929,#11718);
#6844=LINE('',#52935,#11719);
#6845=LINE('',#52938,#11720);
#6846=LINE('',#52944,#11721);
#6847=LINE('',#52947,#11722);
#6848=LINE('',#52953,#11723);
#6849=LINE('',#52956,#11724);
#6850=LINE('',#52962,#11725);
#6851=LINE('',#52965,#11726);
#6852=LINE('',#52971,#11727);
#6853=LINE('',#52974,#11728);
#6854=LINE('',#52980,#11729);
#6855=LINE('',#52983,#11730);
#6856=LINE('',#52989,#11731);
#6857=LINE('',#52992,#11732);
#6858=LINE('',#52998,#11733);
#6859=LINE('',#53001,#11734);
#6860=LINE('',#53007,#11735);
#6861=LINE('',#53010,#11736);
#6862=LINE('',#53016,#11737);
#6863=LINE('',#53019,#11738);
#6864=LINE('',#53025,#11739);
#6865=LINE('',#53028,#11740);
#6866=LINE('',#53034,#11741);
#6867=LINE('',#53037,#11742);
#6868=LINE('',#53043,#11743);
#6869=LINE('',#53046,#11744);
#6870=LINE('',#53052,#11745);
#6871=LINE('',#53055,#11746);
#6872=LINE('',#53061,#11747);
#6873=LINE('',#53064,#11748);
#6874=LINE('',#53070,#11749);
#6875=LINE('',#53073,#11750);
#6876=LINE('',#53079,#11751);
#6877=LINE('',#53082,#11752);
#6878=LINE('',#53103,#11753);
#6879=LINE('',#53112,#11754);
#6880=LINE('',#53131,#11755);
#6881=LINE('',#53138,#11756);
#6882=LINE('',#53157,#11757);
#6883=LINE('',#53164,#11758);
#6884=LINE('',#53186,#11759);
#6885=LINE('',#53194,#11760);
#6886=LINE('',#53216,#11761);
#6887=LINE('',#53224,#11762);
#6888=LINE('',#53229,#11763);
#6889=LINE('',#53235,#11764);
#6890=LINE('',#53241,#11765);
#6891=LINE('',#53247,#11766);
#6892=LINE('',#53273,#11767);
#6893=LINE('',#53279,#11768);
#6894=LINE('',#53285,#11769);
#6895=LINE('',#53291,#11770);
#6896=LINE('',#53320,#11771);
#6897=LINE('',#53330,#11772);
#6898=LINE('',#53334,#11773);
#6899=LINE('',#53336,#11774);
#6900=LINE('',#53338,#11775);
#6901=LINE('',#53342,#11776);
#6902=LINE('',#53346,#11777);
#6903=LINE('',#53348,#11778);
#6904=LINE('',#53350,#11779);
#6905=LINE('',#53352,#11780);
#6906=LINE('',#53354,#11781);
#6907=LINE('',#53356,#11782);
#6908=LINE('',#53358,#11783);
#6909=LINE('',#53360,#11784);
#6910=LINE('',#53362,#11785);
#6911=LINE('',#53364,#11786);
#6912=LINE('',#53366,#11787);
#6913=LINE('',#53370,#11788);
#6914=LINE('',#53374,#11789);
#6915=LINE('',#53376,#11790);
#6916=LINE('',#53378,#11791);
#6917=LINE('',#53380,#11792);
#6918=LINE('',#53382,#11793);
#6919=LINE('',#53384,#11794);
#6920=LINE('',#53386,#11795);
#6921=LINE('',#53387,#11796);
#6922=LINE('',#53390,#11797);
#6923=LINE('',#53392,#11798);
#6924=LINE('',#53394,#11799);
#6925=LINE('',#53396,#11800);
#6926=LINE('',#53398,#11801);
#6927=LINE('',#53400,#11802);
#6928=LINE('',#53402,#11803);
#6929=LINE('',#53403,#11804);
#6930=LINE('',#53406,#11805);
#6931=LINE('',#53408,#11806);
#6932=LINE('',#53410,#11807);
#6933=LINE('',#53412,#11808);
#6934=LINE('',#53414,#11809);
#6935=LINE('',#53416,#11810);
#6936=LINE('',#53418,#11811);
#6937=LINE('',#53419,#11812);
#6938=LINE('',#53422,#11813);
#6939=LINE('',#53424,#11814);
#6940=LINE('',#53426,#11815);
#6941=LINE('',#53428,#11816);
#6942=LINE('',#53430,#11817);
#6943=LINE('',#53432,#11818);
#6944=LINE('',#53434,#11819);
#6945=LINE('',#53435,#11820);
#6946=LINE('',#53438,#11821);
#6947=LINE('',#53440,#11822);
#6948=LINE('',#53442,#11823);
#6949=LINE('',#53444,#11824);
#6950=LINE('',#53446,#11825);
#6951=LINE('',#53448,#11826);
#6952=LINE('',#53450,#11827);
#6953=LINE('',#53451,#11828);
#6954=LINE('',#53455,#11829);
#6955=LINE('',#53457,#11830);
#6956=LINE('',#53459,#11831);
#6957=LINE('',#53461,#11832);
#6958=LINE('',#53463,#11833);
#6959=LINE('',#53465,#11834);
#6960=LINE('',#53467,#11835);
#6961=LINE('',#53469,#11836);
#6962=LINE('',#53471,#11837);
#6963=LINE('',#53473,#11838);
#6964=LINE('',#53477,#11839);
#6965=LINE('',#53481,#11840);
#6966=LINE('',#53483,#11841);
#6967=LINE('',#53485,#11842);
#6968=LINE('',#53487,#11843);
#6969=LINE('',#53489,#11844);
#6970=LINE('',#53491,#11845);
#6971=LINE('',#53493,#11846);
#6972=LINE('',#53495,#11847);
#6973=LINE('',#53497,#11848);
#6974=LINE('',#53499,#11849);
#6975=LINE('',#53501,#11850);
#6976=LINE('',#53505,#11851);
#6977=LINE('',#53508,#11852);
#6978=LINE('',#53511,#11853);
#6979=LINE('',#53513,#11854);
#6980=LINE('',#53515,#11855);
#6981=LINE('',#53516,#11856);
#6982=LINE('',#53519,#11857);
#6983=LINE('',#53521,#11858);
#6984=LINE('',#53523,#11859);
#6985=LINE('',#53524,#11860);
#6986=LINE('',#53527,#11861);
#6987=LINE('',#53529,#11862);
#6988=LINE('',#53531,#11863);
#6989=LINE('',#53532,#11864);
#6990=LINE('',#53535,#11865);
#6991=LINE('',#53537,#11866);
#6992=LINE('',#53539,#11867);
#6993=LINE('',#53540,#11868);
#6994=LINE('',#53542,#11869);
#6995=LINE('',#53543,#11870);
#6996=LINE('',#53545,#11871);
#6997=LINE('',#53546,#11872);
#6998=LINE('',#53550,#11873);
#6999=LINE('',#53552,#11874);
#7000=LINE('',#53554,#11875);
#7001=LINE('',#53558,#11876);
#7002=LINE('',#53562,#11877);
#7003=LINE('',#53564,#11878);
#7004=LINE('',#53566,#11879);
#7005=LINE('',#53568,#11880);
#7006=LINE('',#53570,#11881);
#7007=LINE('',#53572,#11882);
#7008=LINE('',#53574,#11883);
#7009=LINE('',#53575,#11884);
#7010=LINE('',#53578,#11885);
#7011=LINE('',#53580,#11886);
#7012=LINE('',#53582,#11887);
#7013=LINE('',#53584,#11888);
#7014=LINE('',#53586,#11889);
#7015=LINE('',#53588,#11890);
#7016=LINE('',#53590,#11891);
#7017=LINE('',#53591,#11892);
#7018=LINE('',#53595,#11893);
#7019=LINE('',#53597,#11894);
#7020=LINE('',#53601,#11895);
#7021=LINE('',#53604,#11896);
#7022=LINE('',#53607,#11897);
#7023=LINE('',#53609,#11898);
#7024=LINE('',#53611,#11899);
#7025=LINE('',#53612,#11900);
#7026=LINE('',#53615,#11901);
#7027=LINE('',#53617,#11902);
#7028=LINE('',#53619,#11903);
#7029=LINE('',#53620,#11904);
#7030=LINE('',#53622,#11905);
#7031=LINE('',#53623,#11906);
#7032=LINE('',#53625,#11907);
#7033=LINE('',#53626,#11908);
#7034=LINE('',#53630,#11909);
#7035=LINE('',#53632,#11910);
#7036=LINE('',#53634,#11911);
#7037=LINE('',#53636,#11912);
#7038=LINE('',#53638,#11913);
#7039=LINE('',#53640,#11914);
#7040=LINE('',#53644,#11915);
#7041=LINE('',#53647,#11916);
#7042=LINE('',#53649,#11917);
#7043=LINE('',#53651,#11918);
#7044=LINE('',#53654,#11919);
#7045=LINE('',#53656,#11920);
#7046=LINE('',#53659,#11921);
#7047=LINE('',#53661,#11922);
#7048=LINE('',#53664,#11923);
#7049=LINE('',#53666,#11924);
#7050=LINE('',#53669,#11925);
#7051=LINE('',#53671,#11926);
#7052=LINE('',#53674,#11927);
#7053=LINE('',#53676,#11928);
#7054=LINE('',#53679,#11929);
#7055=LINE('',#53681,#11930);
#7056=LINE('',#53684,#11931);
#7057=LINE('',#53686,#11932);
#7058=LINE('',#53689,#11933);
#7059=LINE('',#53691,#11934);
#7060=LINE('',#53694,#11935);
#7061=LINE('',#53696,#11936);
#7062=LINE('',#53699,#11937);
#7063=LINE('',#53701,#11938);
#7064=LINE('',#53704,#11939);
#7065=LINE('',#53706,#11940);
#7066=LINE('',#53709,#11941);
#7067=LINE('',#53712,#11942);
#7068=LINE('',#53714,#11943);
#7069=LINE('',#53717,#11944);
#7070=LINE('',#53719,#11945);
#7071=LINE('',#53722,#11946);
#7072=LINE('',#53724,#11947);
#7073=LINE('',#53727,#11948);
#7074=LINE('',#53729,#11949);
#7075=LINE('',#53732,#11950);
#7076=LINE('',#53734,#11951);
#7077=LINE('',#53737,#11952);
#7078=LINE('',#53739,#11953);
#7079=LINE('',#53742,#11954);
#7080=LINE('',#53744,#11955);
#7081=LINE('',#53747,#11956);
#7082=LINE('',#53749,#11957);
#7083=LINE('',#53752,#11958);
#7084=LINE('',#53754,#11959);
#7085=LINE('',#53757,#11960);
#7086=LINE('',#53759,#11961);
#7087=LINE('',#53762,#11962);
#7088=LINE('',#53764,#11963);
#7089=LINE('',#53767,#11964);
#7090=LINE('',#53769,#11965);
#7091=LINE('',#53772,#11966);
#7092=LINE('',#53774,#11967);
#7093=LINE('',#53777,#11968);
#7094=LINE('',#53779,#11969);
#7095=LINE('',#53782,#11970);
#7096=LINE('',#53784,#11971);
#7097=LINE('',#53787,#11972);
#7098=LINE('',#53789,#11973);
#7099=LINE('',#53792,#11974);
#7100=LINE('',#53794,#11975);
#7101=LINE('',#53797,#11976);
#7102=LINE('',#53799,#11977);
#7103=LINE('',#53802,#11978);
#7104=LINE('',#53804,#11979);
#7105=LINE('',#53807,#11980);
#7106=LINE('',#53809,#11981);
#7107=LINE('',#53812,#11982);
#7108=LINE('',#53814,#11983);
#7109=LINE('',#53817,#11984);
#7110=LINE('',#53819,#11985);
#7111=LINE('',#53822,#11986);
#7112=LINE('',#53824,#11987);
#7113=LINE('',#53827,#11988);
#7114=LINE('',#53829,#11989);
#7115=LINE('',#53831,#11990);
#7116=LINE('',#53834,#11991);
#7117=LINE('',#53836,#11992);
#7118=LINE('',#53839,#11993);
#7119=LINE('',#53841,#11994);
#7120=LINE('',#53844,#11995);
#7121=LINE('',#53846,#11996);
#7122=LINE('',#53849,#11997);
#7123=LINE('',#53851,#11998);
#7124=LINE('',#53854,#11999);
#7125=LINE('',#53856,#12000);
#7126=LINE('',#53859,#12001);
#7127=LINE('',#53861,#12002);
#7128=LINE('',#53864,#12003);
#7129=LINE('',#53866,#12004);
#7130=LINE('',#53869,#12005);
#7131=LINE('',#53871,#12006);
#7132=LINE('',#53874,#12007);
#7133=LINE('',#53876,#12008);
#7134=LINE('',#53879,#12009);
#7135=LINE('',#53881,#12010);
#7136=LINE('',#53884,#12011);
#7137=LINE('',#53886,#12012);
#7138=LINE('',#53891,#12013);
#7139=LINE('',#53893,#12014);
#7140=LINE('',#53895,#12015);
#7141=LINE('',#53897,#12016);
#7142=LINE('',#53901,#12017);
#7143=LINE('',#53905,#12018);
#7144=LINE('',#53907,#12019);
#7145=LINE('',#53908,#12020);
#7146=LINE('',#53910,#12021);
#7147=LINE('',#53913,#12022);
#7148=LINE('',#53915,#12023);
#7149=LINE('',#53918,#12024);
#7150=LINE('',#53920,#12025);
#7151=LINE('',#53923,#12026);
#7152=LINE('',#53925,#12027);
#7153=LINE('',#53928,#12028);
#7154=LINE('',#53930,#12029);
#7155=LINE('',#53933,#12030);
#7156=LINE('',#53935,#12031);
#7157=LINE('',#53938,#12032);
#7158=LINE('',#53940,#12033);
#7159=LINE('',#53943,#12034);
#7160=LINE('',#53945,#12035);
#7161=LINE('',#53948,#12036);
#7162=LINE('',#53950,#12037);
#7163=LINE('',#53953,#12038);
#7164=LINE('',#53955,#12039);
#7165=LINE('',#53958,#12040);
#7166=LINE('',#53960,#12041);
#7167=LINE('',#53963,#12042);
#7168=LINE('',#53965,#12043);
#7169=LINE('',#53968,#12044);
#7170=LINE('',#53970,#12045);
#7171=LINE('',#53973,#12046);
#7172=LINE('',#53975,#12047);
#7173=LINE('',#53977,#12048);
#7174=LINE('',#53980,#12049);
#7175=LINE('',#53982,#12050);
#7176=LINE('',#53985,#12051);
#7177=LINE('',#53987,#12052);
#7178=LINE('',#53990,#12053);
#7179=LINE('',#53992,#12054);
#7180=LINE('',#53995,#12055);
#7181=LINE('',#53997,#12056);
#7182=LINE('',#54000,#12057);
#7183=LINE('',#54002,#12058);
#7184=LINE('',#54005,#12059);
#7185=LINE('',#54007,#12060);
#7186=LINE('',#54010,#12061);
#7187=LINE('',#54012,#12062);
#7188=LINE('',#54015,#12063);
#7189=LINE('',#54017,#12064);
#7190=LINE('',#54020,#12065);
#7191=LINE('',#54022,#12066);
#7192=LINE('',#54025,#12067);
#7193=LINE('',#54027,#12068);
#7194=LINE('',#54030,#12069);
#7195=LINE('',#54032,#12070);
#7196=LINE('',#54035,#12071);
#7197=LINE('',#54037,#12072);
#7198=LINE('',#54040,#12073);
#7199=LINE('',#54042,#12074);
#7200=LINE('',#54045,#12075);
#7201=LINE('',#54047,#12076);
#7202=LINE('',#54050,#12077);
#7203=LINE('',#54052,#12078);
#7204=LINE('',#54055,#12079);
#7205=LINE('',#54057,#12080);
#7206=LINE('',#54060,#12081);
#7207=LINE('',#54062,#12082);
#7208=LINE('',#54065,#12083);
#7209=LINE('',#54067,#12084);
#7210=LINE('',#54070,#12085);
#7211=LINE('',#54072,#12086);
#7212=LINE('',#54075,#12087);
#7213=LINE('',#54077,#12088);
#7214=LINE('',#54080,#12089);
#7215=LINE('',#54082,#12090);
#7216=LINE('',#54085,#12091);
#7217=LINE('',#54087,#12092);
#7218=LINE('',#54090,#12093);
#7219=LINE('',#54092,#12094);
#7220=LINE('',#54095,#12095);
#7221=LINE('',#54098,#12096);
#7222=LINE('',#54100,#12097);
#7223=LINE('',#54103,#12098);
#7224=LINE('',#54105,#12099);
#7225=LINE('',#54108,#12100);
#7226=LINE('',#54110,#12101);
#7227=LINE('',#54113,#12102);
#7228=LINE('',#54115,#12103);
#7229=LINE('',#54118,#12104);
#7230=LINE('',#54120,#12105);
#7231=LINE('',#54123,#12106);
#7232=LINE('',#54125,#12107);
#7233=LINE('',#54128,#12108);
#7234=LINE('',#54130,#12109);
#7235=LINE('',#54133,#12110);
#7236=LINE('',#54135,#12111);
#7237=LINE('',#54138,#12112);
#7238=LINE('',#54140,#12113);
#7239=LINE('',#54143,#12114);
#7240=LINE('',#54145,#12115);
#7241=LINE('',#54148,#12116);
#7242=LINE('',#54151,#12117);
#7243=LINE('',#54153,#12118);
#7244=LINE('',#54154,#12119);
#7245=LINE('',#54157,#12120);
#7246=LINE('',#54159,#12121);
#7247=LINE('',#54160,#12122);
#7248=LINE('',#54164,#12123);
#7249=LINE('',#54166,#12124);
#7250=LINE('',#54168,#12125);
#7251=LINE('',#54169,#12126);
#7252=LINE('',#54172,#12127);
#7253=LINE('',#54174,#12128);
#7254=LINE('',#54175,#12129);
#7255=LINE('',#54179,#12130);
#7256=LINE('',#54181,#12131);
#7257=LINE('',#54183,#12132);
#7258=LINE('',#54184,#12133);
#7259=LINE('',#54187,#12134);
#7260=LINE('',#54189,#12135);
#7261=LINE('',#54190,#12136);
#7262=LINE('',#54193,#12137);
#7263=LINE('',#54195,#12138);
#7264=LINE('',#54196,#12139);
#7265=LINE('',#54200,#12140);
#7266=LINE('',#54202,#12141);
#7267=LINE('',#54204,#12142);
#7268=LINE('',#54205,#12143);
#7269=LINE('',#54209,#12144);
#7270=LINE('',#54211,#12145);
#7271=LINE('',#54213,#12146);
#7272=LINE('',#54214,#12147);
#7273=LINE('',#54217,#12148);
#7274=LINE('',#54219,#12149);
#7275=LINE('',#54220,#12150);
#7276=LINE('',#54224,#12151);
#7277=LINE('',#54226,#12152);
#7278=LINE('',#54228,#12153);
#7279=LINE('',#54229,#12154);
#7280=LINE('',#54233,#12155);
#7281=LINE('',#54235,#12156);
#7282=LINE('',#54237,#12157);
#7283=LINE('',#54238,#12158);
#7284=LINE('',#54241,#12159);
#7285=LINE('',#54243,#12160);
#7286=LINE('',#54244,#12161);
#7287=LINE('',#54247,#12162);
#7288=LINE('',#54249,#12163);
#7289=LINE('',#54250,#12164);
#7290=LINE('',#54254,#12165);
#7291=LINE('',#54256,#12166);
#7292=LINE('',#54258,#12167);
#7293=LINE('',#54259,#12168);
#7294=LINE('',#54262,#12169);
#7295=LINE('',#54264,#12170);
#7296=LINE('',#54265,#12171);
#7297=LINE('',#54269,#12172);
#7298=LINE('',#54271,#12173);
#7299=LINE('',#54273,#12174);
#7300=LINE('',#54274,#12175);
#7301=LINE('',#54277,#12176);
#7302=LINE('',#54279,#12177);
#7303=LINE('',#54280,#12178);
#7304=LINE('',#54283,#12179);
#7305=LINE('',#54285,#12180);
#7306=LINE('',#54286,#12181);
#7307=LINE('',#54290,#12182);
#7308=LINE('',#54292,#12183);
#7309=LINE('',#54294,#12184);
#7310=LINE('',#54295,#12185);
#7311=LINE('',#54299,#12186);
#7312=LINE('',#54301,#12187);
#7313=LINE('',#54303,#12188);
#7314=LINE('',#54304,#12189);
#7315=LINE('',#54307,#12190);
#7316=LINE('',#54309,#12191);
#7317=LINE('',#54310,#12192);
#7318=LINE('',#54314,#12193);
#7319=LINE('',#54316,#12194);
#7320=LINE('',#54318,#12195);
#7321=LINE('',#54319,#12196);
#7322=LINE('',#54323,#12197);
#7323=LINE('',#54325,#12198);
#7324=LINE('',#54327,#12199);
#7325=LINE('',#54328,#12200);
#7326=LINE('',#54371,#12201);
#7327=LINE('',#54386,#12202);
#7328=LINE('',#54406,#12203);
#7329=LINE('',#54418,#12204);
#7330=LINE('',#54426,#12205);
#7331=LINE('',#54436,#12206);
#7332=LINE('',#54450,#12207);
#7333=LINE('',#54461,#12208);
#7334=LINE('',#54475,#12209);
#7335=LINE('',#54489,#12210);
#7336=LINE('',#54500,#12211);
#7337=LINE('',#54513,#12212);
#7338=LINE('',#54526,#12213);
#7339=LINE('',#54538,#12214);
#7340=LINE('',#54824,#12215);
#7341=LINE('',#54825,#12216);
#7342=LINE('',#54866,#12217);
#7343=LINE('',#54894,#12218);
#7344=LINE('',#54935,#12219);
#7345=LINE('',#54952,#12220);
#7346=LINE('',#54954,#12221);
#7347=LINE('',#54956,#12222);
#7348=LINE('',#54958,#12223);
#7349=LINE('',#54962,#12224);
#7350=LINE('',#54966,#12225);
#7351=LINE('',#54968,#12226);
#7352=LINE('',#54969,#12227);
#7353=LINE('',#54972,#12228);
#7354=LINE('',#54974,#12229);
#7355=LINE('',#54976,#12230);
#7356=LINE('',#54977,#12231);
#7357=LINE('',#54982,#12232);
#7358=LINE('',#54986,#12233);
#7359=LINE('',#54990,#12234);
#7360=LINE('',#54994,#12235);
#7361=LINE('',#54998,#12236);
#7362=LINE('',#55001,#12237);
#7363=LINE('',#55005,#12238);
#7364=LINE('',#55007,#12239);
#7365=LINE('',#55009,#12240);
#7366=LINE('',#55011,#12241);
#7367=LINE('',#55013,#12242);
#7368=LINE('',#55015,#12243);
#7369=LINE('',#55019,#12244);
#7370=LINE('',#55022,#12245);
#7371=LINE('',#55025,#12246);
#7372=LINE('',#55027,#12247);
#7373=LINE('',#55029,#12248);
#7374=LINE('',#55030,#12249);
#7375=LINE('',#55033,#12250);
#7376=LINE('',#55037,#12251);
#7377=LINE('',#55041,#12252);
#7378=LINE('',#55045,#12253);
#7379=LINE('',#55049,#12254);
#7380=LINE('',#55053,#12255);
#7381=LINE('',#55057,#12256);
#7382=LINE('',#55058,#12257);
#7383=LINE('',#55059,#12258);
#7384=LINE('',#55063,#12259);
#7385=LINE('',#55064,#12260);
#7386=LINE('',#55065,#12261);
#7387=LINE('',#55069,#12262);
#7388=LINE('',#55070,#12263);
#7389=LINE('',#55071,#12264);
#7390=LINE('',#55075,#12265);
#7391=LINE('',#55076,#12266);
#7392=LINE('',#55077,#12267);
#7393=LINE('',#55140,#12268);
#7394=LINE('',#55141,#12269);
#7395=LINE('',#55226,#12270);
#7396=LINE('',#55227,#12271);
#7397=LINE('',#55294,#12272);
#7398=LINE('',#55295,#12273);
#7399=LINE('',#55297,#12274);
#7400=LINE('',#55299,#12275);
#7401=LINE('',#55300,#12276);
#7402=LINE('',#55302,#12277);
#7403=LINE('',#55303,#12278);
#7404=LINE('',#55305,#12279);
#7405=LINE('',#55349,#12280);
#7406=LINE('',#55350,#12281);
#7407=LINE('',#55475,#12282);
#7408=LINE('',#55476,#12283);
#7409=LINE('',#55523,#12284);
#7410=LINE('',#55524,#12285);
#7411=LINE('',#55526,#12286);
#7412=LINE('',#55528,#12287);
#7413=LINE('',#55529,#12288);
#7414=LINE('',#55531,#12289);
#7415=LINE('',#55532,#12290);
#7416=LINE('',#55534,#12291);
#7417=LINE('',#55547,#12292);
#7418=LINE('',#55553,#12293);
#7419=LINE('',#55559,#12294);
#7420=LINE('',#55563,#12295);
#7421=LINE('',#55566,#12296);
#7422=LINE('',#55570,#12297);
#7423=LINE('',#55574,#12298);
#7424=LINE('',#55577,#12299);
#7425=LINE('',#55582,#12300);
#7426=LINE('',#55586,#12301);
#7427=LINE('',#55589,#12302);
#7428=LINE('',#55593,#12303);
#7429=LINE('',#55597,#12304);
#7430=LINE('',#55600,#12305);
#7431=LINE('',#55602,#12306);
#7432=LINE('',#55603,#12307);
#7433=LINE('',#55605,#12308);
#7434=LINE('',#55606,#12309);
#7435=LINE('',#55611,#12310);
#7436=LINE('',#55612,#12311);
#7437=LINE('',#55614,#12312);
#7438=LINE('',#55615,#12313);
#7439=LINE('',#55617,#12314);
#7440=LINE('',#55619,#12315);
#7441=LINE('',#55633,#12316);
#7442=LINE('',#55639,#12317);
#7443=LINE('',#55645,#12318);
#7444=LINE('',#55649,#12319);
#7445=LINE('',#55652,#12320);
#7446=LINE('',#55656,#12321);
#7447=LINE('',#55660,#12322);
#7448=LINE('',#55663,#12323);
#7449=LINE('',#55668,#12324);
#7450=LINE('',#55672,#12325);
#7451=LINE('',#55675,#12326);
#7452=LINE('',#55679,#12327);
#7453=LINE('',#55683,#12328);
#7454=LINE('',#55686,#12329);
#7455=LINE('',#55688,#12330);
#7456=LINE('',#55689,#12331);
#7457=LINE('',#55691,#12332);
#7458=LINE('',#55692,#12333);
#7459=LINE('',#55697,#12334);
#7460=LINE('',#55698,#12335);
#7461=LINE('',#55700,#12336);
#7462=LINE('',#55701,#12337);
#7463=LINE('',#55703,#12338);
#7464=LINE('',#55705,#12339);
#7465=LINE('',#55719,#12340);
#7466=LINE('',#55725,#12341);
#7467=LINE('',#55731,#12342);
#7468=LINE('',#55735,#12343);
#7469=LINE('',#55738,#12344);
#7470=LINE('',#55742,#12345);
#7471=LINE('',#55746,#12346);
#7472=LINE('',#55749,#12347);
#7473=LINE('',#55754,#12348);
#7474=LINE('',#55758,#12349);
#7475=LINE('',#55761,#12350);
#7476=LINE('',#55765,#12351);
#7477=LINE('',#55769,#12352);
#7478=LINE('',#55772,#12353);
#7479=LINE('',#55774,#12354);
#7480=LINE('',#55775,#12355);
#7481=LINE('',#55777,#12356);
#7482=LINE('',#55778,#12357);
#7483=LINE('',#55783,#12358);
#7484=LINE('',#55784,#12359);
#7485=LINE('',#55786,#12360);
#7486=LINE('',#55787,#12361);
#7487=LINE('',#55789,#12362);
#7488=LINE('',#55791,#12363);
#7489=LINE('',#55805,#12364);
#7490=LINE('',#55811,#12365);
#7491=LINE('',#55817,#12366);
#7492=LINE('',#55821,#12367);
#7493=LINE('',#55824,#12368);
#7494=LINE('',#55828,#12369);
#7495=LINE('',#55832,#12370);
#7496=LINE('',#55835,#12371);
#7497=LINE('',#55840,#12372);
#7498=LINE('',#55844,#12373);
#7499=LINE('',#55847,#12374);
#7500=LINE('',#55851,#12375);
#7501=LINE('',#55855,#12376);
#7502=LINE('',#55858,#12377);
#7503=LINE('',#55860,#12378);
#7504=LINE('',#55861,#12379);
#7505=LINE('',#55863,#12380);
#7506=LINE('',#55864,#12381);
#7507=LINE('',#55869,#12382);
#7508=LINE('',#55870,#12383);
#7509=LINE('',#55872,#12384);
#7510=LINE('',#55873,#12385);
#7511=LINE('',#55875,#12386);
#7512=LINE('',#55877,#12387);
#7513=LINE('',#55899,#12388);
#7514=LINE('',#55913,#12389);
#7515=LINE('',#55924,#12390);
#7516=LINE('',#55939,#12391);
#7517=LINE('',#55949,#12392);
#7518=LINE('',#55962,#12393);
#7519=LINE('',#55975,#12394);
#7520=LINE('',#55988,#12395);
#7521=LINE('',#56000,#12396);
#7522=LINE('',#56011,#12397);
#7523=LINE('',#56024,#12398);
#7524=LINE('',#56266,#12399);
#7525=LINE('',#56267,#12400);
#7526=LINE('',#56269,#12401);
#7527=LINE('',#56271,#12402);
#7528=LINE('',#56272,#12403);
#7529=LINE('',#56274,#12404);
#7530=LINE('',#56276,#12405);
#7531=LINE('',#56277,#12406);
#7532=LINE('',#56279,#12407);
#7533=LINE('',#56281,#12408);
#7534=LINE('',#56283,#12409);
#7535=LINE('',#56284,#12410);
#7536=LINE('',#56286,#12411);
#7537=LINE('',#56287,#12412);
#7538=LINE('',#56289,#12413);
#7539=LINE('',#56291,#12414);
#7540=LINE('',#56292,#12415);
#7541=LINE('',#56294,#12416);
#7542=LINE('',#56295,#12417);
#7543=LINE('',#56312,#12418);
#7544=LINE('',#56313,#12419);
#7545=LINE('',#56330,#12420);
#7546=LINE('',#56347,#12421);
#7547=LINE('',#56348,#12422);
#7548=LINE('',#56365,#12423);
#7549=LINE('',#56390,#12424);
#7550=LINE('',#56407,#12425);
#7551=LINE('',#56424,#12426);
#7552=LINE('',#56425,#12427);
#7553=LINE('',#56442,#12428);
#7554=LINE('',#56459,#12429);
#7555=LINE('',#56460,#12430);
#7556=LINE('',#56479,#12431);
#7557=LINE('',#56480,#12432);
#7558=LINE('',#56499,#12433);
#7559=LINE('',#56516,#12434);
#7560=LINE('',#56517,#12435);
#7561=LINE('',#56534,#12436);
#7562=LINE('',#56551,#12437);
#7563=LINE('',#56552,#12438);
#7564=LINE('',#56569,#12439);
#7565=LINE('',#56590,#12440);
#7566=LINE('',#56607,#12441);
#7567=LINE('',#56624,#12442);
#7568=LINE('',#56625,#12443);
#7569=LINE('',#56642,#12444);
#7570=LINE('',#56659,#12445);
#7571=LINE('',#56660,#12446);
#7572=LINE('',#56675,#12447);
#7573=LINE('',#56676,#12448);
#7574=LINE('',#56691,#12449);
#7575=LINE('',#56704,#12450);
#7576=LINE('',#56717,#12451);
#7577=LINE('',#56728,#12452);
#7578=LINE('',#56741,#12453);
#7579=LINE('',#56742,#12454);
#7580=LINE('',#56755,#12455);
#7581=LINE('',#56756,#12456);
#7582=LINE('',#56771,#12457);
#7583=LINE('',#56772,#12458);
#7584=LINE('',#56828,#12459);
#7585=LINE('',#56829,#12460);
#7586=LINE('',#56831,#12461);
#7587=LINE('',#56833,#12462);
#7588=LINE('',#56835,#12463);
#7589=LINE('',#56837,#12464);
#7590=LINE('',#56839,#12465);
#7591=LINE('',#56841,#12466);
#7592=LINE('',#56843,#12467);
#7593=LINE('',#56845,#12468);
#7594=LINE('',#56847,#12469);
#7595=LINE('',#56849,#12470);
#7596=LINE('',#56852,#12471);
#7597=LINE('',#56853,#12472);
#7598=LINE('',#56855,#12473);
#7599=LINE('',#56857,#12474);
#7600=LINE('',#56864,#12475);
#7601=LINE('',#56866,#12476);
#7602=LINE('',#56869,#12477);
#7603=LINE('',#56871,#12478);
#7604=LINE('',#56874,#12479);
#7605=LINE('',#56876,#12480);
#7606=LINE('',#56879,#12481);
#7607=LINE('',#56881,#12482);
#7608=LINE('',#56884,#12483);
#7609=LINE('',#56886,#12484);
#7610=LINE('',#56889,#12485);
#7611=LINE('',#56891,#12486);
#7612=LINE('',#56894,#12487);
#7613=LINE('',#56896,#12488);
#7614=LINE('',#56899,#12489);
#7615=LINE('',#56901,#12490);
#7616=LINE('',#56904,#12491);
#7617=LINE('',#56906,#12492);
#7618=LINE('',#56909,#12493);
#7619=LINE('',#56911,#12494);
#7620=LINE('',#56914,#12495);
#7621=LINE('',#56916,#12496);
#7622=LINE('',#56919,#12497);
#7623=LINE('',#56921,#12498);
#7624=LINE('',#56924,#12499);
#7625=LINE('',#56926,#12500);
#7626=LINE('',#56929,#12501);
#7627=LINE('',#56931,#12502);
#7628=LINE('',#56934,#12503);
#7629=LINE('',#56936,#12504);
#7630=LINE('',#56939,#12505);
#7631=LINE('',#56941,#12506);
#7632=LINE('',#56944,#12507);
#7633=LINE('',#56946,#12508);
#7634=LINE('',#56949,#12509);
#7635=LINE('',#56951,#12510);
#7636=LINE('',#56954,#12511);
#7637=LINE('',#56956,#12512);
#7638=LINE('',#56959,#12513);
#7639=LINE('',#56961,#12514);
#7640=LINE('',#56964,#12515);
#7641=LINE('',#56966,#12516);
#7642=LINE('',#56969,#12517);
#7643=LINE('',#56971,#12518);
#7644=LINE('',#56974,#12519);
#7645=LINE('',#56976,#12520);
#7646=LINE('',#56979,#12521);
#7647=LINE('',#56981,#12522);
#7648=LINE('',#56984,#12523);
#7649=LINE('',#56986,#12524);
#7650=LINE('',#56989,#12525);
#7651=LINE('',#56991,#12526);
#7652=LINE('',#56994,#12527);
#7653=LINE('',#56996,#12528);
#7654=LINE('',#56999,#12529);
#7655=LINE('',#57001,#12530);
#7656=LINE('',#57004,#12531);
#7657=LINE('',#57006,#12532);
#7658=LINE('',#57009,#12533);
#7659=LINE('',#57011,#12534);
#7660=LINE('',#57014,#12535);
#7661=LINE('',#57016,#12536);
#7662=LINE('',#57019,#12537);
#7663=LINE('',#57021,#12538);
#7664=LINE('',#57024,#12539);
#7665=LINE('',#57026,#12540);
#7666=LINE('',#57029,#12541);
#7667=LINE('',#57031,#12542);
#7668=LINE('',#57034,#12543);
#7669=LINE('',#57036,#12544);
#7670=LINE('',#57039,#12545);
#7671=LINE('',#57041,#12546);
#7672=LINE('',#57044,#12547);
#7673=LINE('',#57046,#12548);
#7674=LINE('',#57049,#12549);
#7675=LINE('',#57051,#12550);
#7676=LINE('',#57054,#12551);
#7677=LINE('',#57056,#12552);
#7678=LINE('',#57059,#12553);
#7679=LINE('',#57061,#12554);
#7680=LINE('',#57064,#12555);
#7681=LINE('',#57066,#12556);
#7682=LINE('',#57069,#12557);
#7683=LINE('',#57071,#12558);
#7684=LINE('',#57074,#12559);
#7685=LINE('',#57076,#12560);
#7686=LINE('',#57079,#12561);
#7687=LINE('',#57081,#12562);
#7688=LINE('',#57084,#12563);
#7689=LINE('',#57086,#12564);
#7690=LINE('',#57089,#12565);
#7691=LINE('',#57091,#12566);
#7692=LINE('',#57094,#12567);
#7693=LINE('',#57096,#12568);
#7694=LINE('',#57099,#12569);
#7695=LINE('',#57101,#12570);
#7696=LINE('',#57104,#12571);
#7697=LINE('',#57106,#12572);
#7698=LINE('',#57108,#12573);
#7699=LINE('',#57110,#12574);
#7700=LINE('',#57111,#12575);
#7701=LINE('',#57113,#12576);
#7702=LINE('',#57116,#12577);
#7703=LINE('',#57121,#12578);
#7704=LINE('',#57126,#12579);
#7705=LINE('',#57128,#12580);
#7706=LINE('',#57130,#12581);
#7707=LINE('',#57132,#12582);
#7708=LINE('',#57144,#12583);
#7709=LINE('',#57150,#12584);
#7710=LINE('',#57156,#12585);
#7711=LINE('',#57160,#12586);
#7712=LINE('',#57164,#12587);
#7713=LINE('',#57167,#12588);
#7714=LINE('',#57171,#12589);
#7715=LINE('',#57174,#12590);
#7716=LINE('',#57179,#12591);
#7717=LINE('',#57183,#12592);
#7718=LINE('',#57187,#12593);
#7719=LINE('',#57190,#12594);
#7720=LINE('',#57194,#12595);
#7721=LINE('',#57197,#12596);
#7722=LINE('',#57199,#12597);
#7723=LINE('',#57200,#12598);
#7724=LINE('',#57202,#12599);
#7725=LINE('',#57203,#12600);
#7726=LINE('',#57208,#12601);
#7727=LINE('',#57209,#12602);
#7728=LINE('',#57211,#12603);
#7729=LINE('',#57212,#12604);
#7730=LINE('',#57214,#12605);
#7731=LINE('',#57216,#12606);
#7732=LINE('',#57230,#12607);
#7733=LINE('',#57236,#12608);
#7734=LINE('',#57242,#12609);
#7735=LINE('',#57246,#12610);
#7736=LINE('',#57250,#12611);
#7737=LINE('',#57253,#12612);
#7738=LINE('',#57257,#12613);
#7739=LINE('',#57260,#12614);
#7740=LINE('',#57265,#12615);
#7741=LINE('',#57269,#12616);
#7742=LINE('',#57273,#12617);
#7743=LINE('',#57276,#12618);
#7744=LINE('',#57280,#12619);
#7745=LINE('',#57283,#12620);
#7746=LINE('',#57285,#12621);
#7747=LINE('',#57286,#12622);
#7748=LINE('',#57288,#12623);
#7749=LINE('',#57289,#12624);
#7750=LINE('',#57294,#12625);
#7751=LINE('',#57295,#12626);
#7752=LINE('',#57297,#12627);
#7753=LINE('',#57298,#12628);
#7754=LINE('',#57300,#12629);
#7755=LINE('',#57302,#12630);
#7756=LINE('',#57307,#12631);
#7757=LINE('',#57309,#12632);
#7758=LINE('',#57311,#12633);
#7759=LINE('',#57313,#12634);
#7760=LINE('',#57314,#12635);
#7761=LINE('',#57316,#12636);
#7762=LINE('',#57321,#12637);
#7763=LINE('',#57328,#12638);
#7764=LINE('',#57331,#12639);
#7765=LINE('',#57333,#12640);
#7766=LINE('',#57336,#12641);
#7767=LINE('',#57338,#12642);
#7768=LINE('',#57339,#12643);
#7769=LINE('',#57342,#12644);
#7770=LINE('',#57344,#12645);
#7771=LINE('',#57345,#12646);
#7772=LINE('',#57350,#12647);
#7773=LINE('',#57356,#12648);
#7774=LINE('',#57359,#12649);
#7775=LINE('',#57361,#12650);
#11615=VECTOR('',#42522,1.75);
#11616=VECTOR('',#42529,1.75);
#11617=VECTOR('',#42536,1.75);
#11618=VECTOR('',#42543,1.75);
#11619=VECTOR('',#42550,1.25);
#11620=VECTOR('',#42557,1.25);
#11621=VECTOR('',#42564,1000.);
#11622=VECTOR('',#42567,1000.);
#11623=VECTOR('',#42572,1000.);
#11624=VECTOR('',#42575,1000.);
#11625=VECTOR('',#42580,1000.);
#11626=VECTOR('',#42583,1000.);
#11627=VECTOR('',#42588,1000.);
#11628=VECTOR('',#42591,1000.);
#11629=VECTOR('',#42596,1000.);
#11630=VECTOR('',#42599,1000.);
#11631=VECTOR('',#42604,1000.);
#11632=VECTOR('',#42607,1000.);
#11633=VECTOR('',#42612,1000.);
#11634=VECTOR('',#42615,1000.);
#11635=VECTOR('',#42620,1000.);
#11636=VECTOR('',#42623,1000.);
#11637=VECTOR('',#42628,1000.);
#11638=VECTOR('',#42631,1000.);
#11639=VECTOR('',#42636,1000.);
#11640=VECTOR('',#42639,1000.);
#11641=VECTOR('',#42644,1000.);
#11642=VECTOR('',#42647,1000.);
#11643=VECTOR('',#42652,1000.);
#11644=VECTOR('',#42655,1000.);
#11645=VECTOR('',#42660,1000.);
#11646=VECTOR('',#42663,1000.);
#11647=VECTOR('',#42668,1000.);
#11648=VECTOR('',#42671,1000.);
#11649=VECTOR('',#42676,1000.);
#11650=VECTOR('',#42679,1000.);
#11651=VECTOR('',#42684,1000.);
#11652=VECTOR('',#42687,1000.);
#11653=VECTOR('',#42692,1000.);
#11654=VECTOR('',#42695,1000.);
#11655=VECTOR('',#42700,1000.);
#11656=VECTOR('',#42703,1000.);
#11657=VECTOR('',#42708,1000.);
#11658=VECTOR('',#42711,1000.);
#11659=VECTOR('',#42716,1000.);
#11660=VECTOR('',#42719,1000.);
#11661=VECTOR('',#42724,1000.);
#11662=VECTOR('',#42727,1000.);
#11663=VECTOR('',#42732,1000.);
#11664=VECTOR('',#42735,1000.);
#11665=VECTOR('',#42740,1000.);
#11666=VECTOR('',#42743,1000.);
#11667=VECTOR('',#42748,1000.);
#11668=VECTOR('',#42751,1000.);
#11669=VECTOR('',#42756,1000.);
#11670=VECTOR('',#42759,1000.);
#11671=VECTOR('',#42764,1000.);
#11672=VECTOR('',#42767,1000.);
#11673=VECTOR('',#42772,1000.);
#11674=VECTOR('',#42775,1000.);
#11675=VECTOR('',#42780,1000.);
#11676=VECTOR('',#42783,1000.);
#11677=VECTOR('',#42788,1000.);
#11678=VECTOR('',#42791,1000.);
#11679=VECTOR('',#42796,1000.);
#11680=VECTOR('',#42799,1000.);
#11681=VECTOR('',#42804,1000.);
#11682=VECTOR('',#42807,1000.);
#11683=VECTOR('',#42812,1000.);
#11684=VECTOR('',#42815,1000.);
#11685=VECTOR('',#42820,1000.);
#11686=VECTOR('',#42823,1000.);
#11687=VECTOR('',#42828,1000.);
#11688=VECTOR('',#42831,1000.);
#11689=VECTOR('',#42836,1000.);
#11690=VECTOR('',#42839,1000.);
#11691=VECTOR('',#42844,1000.);
#11692=VECTOR('',#42847,1000.);
#11693=VECTOR('',#42852,1000.);
#11694=VECTOR('',#42855,1000.);
#11695=VECTOR('',#42860,1000.);
#11696=VECTOR('',#42863,1000.);
#11697=VECTOR('',#42868,1000.);
#11698=VECTOR('',#42871,1000.);
#11699=VECTOR('',#42876,1000.);
#11700=VECTOR('',#42879,1000.);
#11701=VECTOR('',#42884,1000.);
#11702=VECTOR('',#42887,1000.);
#11703=VECTOR('',#42892,1000.);
#11704=VECTOR('',#42895,1000.);
#11705=VECTOR('',#42900,1000.);
#11706=VECTOR('',#42903,1000.);
#11707=VECTOR('',#42908,1000.);
#11708=VECTOR('',#42911,1000.);
#11709=VECTOR('',#42916,1000.);
#11710=VECTOR('',#42919,1000.);
#11711=VECTOR('',#42924,1000.);
#11712=VECTOR('',#42927,1000.);
#11713=VECTOR('',#42932,1000.);
#11714=VECTOR('',#42935,1000.);
#11715=VECTOR('',#42940,1000.);
#11716=VECTOR('',#42943,1000.);
#11717=VECTOR('',#42948,1000.);
#11718=VECTOR('',#42951,1000.);
#11719=VECTOR('',#42956,1000.);
#11720=VECTOR('',#42959,1000.);
#11721=VECTOR('',#42964,1000.);
#11722=VECTOR('',#42967,1000.);
#11723=VECTOR('',#42972,1000.);
#11724=VECTOR('',#42975,1000.);
#11725=VECTOR('',#42980,1000.);
#11726=VECTOR('',#42983,1000.);
#11727=VECTOR('',#42988,1000.);
#11728=VECTOR('',#42991,1000.);
#11729=VECTOR('',#42996,1000.);
#11730=VECTOR('',#42999,1000.);
#11731=VECTOR('',#43004,1000.);
#11732=VECTOR('',#43007,1000.);
#11733=VECTOR('',#43012,1000.);
#11734=VECTOR('',#43015,1000.);
#11735=VECTOR('',#43020,1000.);
#11736=VECTOR('',#43023,1000.);
#11737=VECTOR('',#43028,1000.);
#11738=VECTOR('',#43031,1000.);
#11739=VECTOR('',#43036,1000.);
#11740=VECTOR('',#43039,1000.);
#11741=VECTOR('',#43044,1000.);
#11742=VECTOR('',#43047,1000.);
#11743=VECTOR('',#43052,1000.);
#11744=VECTOR('',#43055,1000.);
#11745=VECTOR('',#43060,1000.);
#11746=VECTOR('',#43063,1000.);
#11747=VECTOR('',#43068,1000.);
#11748=VECTOR('',#43071,1000.);
#11749=VECTOR('',#43076,1000.);
#11750=VECTOR('',#43079,1000.);
#11751=VECTOR('',#43084,1000.);
#11752=VECTOR('',#43087,1000.);
#11753=VECTOR('',#43088,1000.);
#11754=VECTOR('',#43089,1000.);
#11755=VECTOR('',#43090,1000.);
#11756=VECTOR('',#43091,1000.);
#11757=VECTOR('',#43092,1000.);
#11758=VECTOR('',#43093,1000.);
#11759=VECTOR('',#43094,1000.);
#11760=VECTOR('',#43095,1000.);
#11761=VECTOR('',#43096,1000.);
#11762=VECTOR('',#43097,1000.);
#11763=VECTOR('',#43102,1.74999999999999);
#11764=VECTOR('',#43109,1.74999999999998);
#11765=VECTOR('',#43116,1.75);
#11766=VECTOR('',#43123,1.75);
#11767=VECTOR('',#43158,1.25);
#11768=VECTOR('',#43165,1.25);
#11769=VECTOR('',#43172,1.25);
#11770=VECTOR('',#43179,1.25);
#11771=VECTOR('',#43182,1000.);
#11772=VECTOR('',#43183,1000.);
#11773=VECTOR('',#43186,1000.);
#11774=VECTOR('',#43187,1000.);
#11775=VECTOR('',#43188,1000.);
#11776=VECTOR('',#43191,1000.);
#11777=VECTOR('',#43194,1000.);
#11778=VECTOR('',#43195,1000.);
#11779=VECTOR('',#43196,1000.);
#11780=VECTOR('',#43197,1000.);
#11781=VECTOR('',#43198,1000.);
#11782=VECTOR('',#43199,1000.);
#11783=VECTOR('',#43200,1000.);
#11784=VECTOR('',#43201,1000.);
#11785=VECTOR('',#43202,1000.);
#11786=VECTOR('',#43203,1000.);
#11787=VECTOR('',#43204,1000.);
#11788=VECTOR('',#43207,1000.);
#11789=VECTOR('',#43210,1000.);
#11790=VECTOR('',#43211,1000.);
#11791=VECTOR('',#43212,1000.);
#11792=VECTOR('',#43213,1000.);
#11793=VECTOR('',#43214,1000.);
#11794=VECTOR('',#43215,1000.);
#11795=VECTOR('',#43216,1000.);
#11796=VECTOR('',#43217,1000.);
#11797=VECTOR('',#43218,1000.);
#11798=VECTOR('',#43219,1000.);
#11799=VECTOR('',#43220,1000.);
#11800=VECTOR('',#43221,1000.);
#11801=VECTOR('',#43222,1000.);
#11802=VECTOR('',#43223,1000.);
#11803=VECTOR('',#43224,1000.);
#11804=VECTOR('',#43225,1000.);
#11805=VECTOR('',#43226,1000.);
#11806=VECTOR('',#43227,1000.);
#11807=VECTOR('',#43228,1000.);
#11808=VECTOR('',#43229,1000.);
#11809=VECTOR('',#43230,1000.);
#11810=VECTOR('',#43231,1000.);
#11811=VECTOR('',#43232,1000.);
#11812=VECTOR('',#43233,1000.);
#11813=VECTOR('',#43234,1000.);
#11814=VECTOR('',#43235,1000.);
#11815=VECTOR('',#43236,1000.);
#11816=VECTOR('',#43237,1000.);
#11817=VECTOR('',#43238,1000.);
#11818=VECTOR('',#43239,1000.);
#11819=VECTOR('',#43240,1000.);
#11820=VECTOR('',#43241,1000.);
#11821=VECTOR('',#43242,1000.);
#11822=VECTOR('',#43243,1000.);
#11823=VECTOR('',#43244,1000.);
#11824=VECTOR('',#43245,1000.);
#11825=VECTOR('',#43246,1000.);
#11826=VECTOR('',#43247,1000.);
#11827=VECTOR('',#43248,1000.);
#11828=VECTOR('',#43249,1000.);
#11829=VECTOR('',#43252,1000.);
#11830=VECTOR('',#43253,1000.);
#11831=VECTOR('',#43254,1000.);
#11832=VECTOR('',#43255,1000.);
#11833=VECTOR('',#43256,1000.);
#11834=VECTOR('',#43257,1000.);
#11835=VECTOR('',#43258,1000.);
#11836=VECTOR('',#43259,1000.);
#11837=VECTOR('',#43260,1000.);
#11838=VECTOR('',#43261,1000.);
#11839=VECTOR('',#43264,1000.);
#11840=VECTOR('',#43267,1000.);
#11841=VECTOR('',#43268,1000.);
#11842=VECTOR('',#43269,1000.);
#11843=VECTOR('',#43270,1000.);
#11844=VECTOR('',#43271,1000.);
#11845=VECTOR('',#43272,1000.);
#11846=VECTOR('',#43273,1000.);
#11847=VECTOR('',#43274,1000.);
#11848=VECTOR('',#43275,1000.);
#11849=VECTOR('',#43276,1000.);
#11850=VECTOR('',#43277,1000.);
#11851=VECTOR('',#43280,1000.);
#11852=VECTOR('',#43283,1000.);
#11853=VECTOR('',#43284,1000.);
#11854=VECTOR('',#43285,1000.);
#11855=VECTOR('',#43286,1000.);
#11856=VECTOR('',#43287,1000.);
#11857=VECTOR('',#43288,1000.);
#11858=VECTOR('',#43289,1000.);
#11859=VECTOR('',#43290,1000.);
#11860=VECTOR('',#43291,1000.);
#11861=VECTOR('',#43292,1000.);
#11862=VECTOR('',#43293,1000.);
#11863=VECTOR('',#43294,1000.);
#11864=VECTOR('',#43295,1000.);
#11865=VECTOR('',#43296,1000.);
#11866=VECTOR('',#43297,1000.);
#11867=VECTOR('',#43298,1000.);
#11868=VECTOR('',#43299,1000.);
#11869=VECTOR('',#43302,1000.);
#11870=VECTOR('',#43303,1000.);
#11871=VECTOR('',#43306,1000.);
#11872=VECTOR('',#43307,1000.);
#11873=VECTOR('',#43310,1000.);
#11874=VECTOR('',#43311,1000.);
#11875=VECTOR('',#43312,1000.);
#11876=VECTOR('',#43315,1000.);
#11877=VECTOR('',#43318,1000.);
#11878=VECTOR('',#43319,1000.);
#11879=VECTOR('',#43320,1000.);
#11880=VECTOR('',#43321,1000.);
#11881=VECTOR('',#43322,1000.);
#11882=VECTOR('',#43323,1000.);
#11883=VECTOR('',#43324,1000.);
#11884=VECTOR('',#43325,1000.);
#11885=VECTOR('',#43326,1000.);
#11886=VECTOR('',#43327,1000.);
#11887=VECTOR('',#43328,1000.);
#11888=VECTOR('',#43329,1000.);
#11889=VECTOR('',#43330,1000.);
#11890=VECTOR('',#43331,1000.);
#11891=VECTOR('',#43332,1000.);
#11892=VECTOR('',#43333,1000.);
#11893=VECTOR('',#43336,1000.);
#11894=VECTOR('',#43337,1000.);
#11895=VECTOR('',#43340,1000.);
#11896=VECTOR('',#43343,1000.);
#11897=VECTOR('',#43344,1000.);
#11898=VECTOR('',#43345,1000.);
#11899=VECTOR('',#43346,1000.);
#11900=VECTOR('',#43347,1000.);
#11901=VECTOR('',#43348,1000.);
#11902=VECTOR('',#43349,1000.);
#11903=VECTOR('',#43350,1000.);
#11904=VECTOR('',#43351,1000.);
#11905=VECTOR('',#43354,1000.);
#11906=VECTOR('',#43355,1000.);
#11907=VECTOR('',#43358,1000.);
#11908=VECTOR('',#43359,1000.);
#11909=VECTOR('',#43362,1000.);
#11910=VECTOR('',#43363,1000.);
#11911=VECTOR('',#43364,1000.);
#11912=VECTOR('',#43365,1000.);
#11913=VECTOR('',#43366,1000.);
#11914=VECTOR('',#43367,1000.);
#11915=VECTOR('',#43370,1000.);
#11916=VECTOR('',#43373,1000.);
#11917=VECTOR('',#43374,1000.);
#11918=VECTOR('',#43375,1000.);
#11919=VECTOR('',#43378,1000.);
#11920=VECTOR('',#43379,1000.);
#11921=VECTOR('',#43382,1000.);
#11922=VECTOR('',#43383,1000.);
#11923=VECTOR('',#43386,1000.);
#11924=VECTOR('',#43387,1000.);
#11925=VECTOR('',#43390,1000.);
#11926=VECTOR('',#43391,1000.);
#11927=VECTOR('',#43394,1000.);
#11928=VECTOR('',#43395,1000.);
#11929=VECTOR('',#43398,1000.);
#11930=VECTOR('',#43399,1000.);
#11931=VECTOR('',#43402,1000.);
#11932=VECTOR('',#43403,1000.);
#11933=VECTOR('',#43406,1000.);
#11934=VECTOR('',#43407,1000.);
#11935=VECTOR('',#43410,1000.);
#11936=VECTOR('',#43411,1000.);
#11937=VECTOR('',#43414,1000.);
#11938=VECTOR('',#43415,1000.);
#11939=VECTOR('',#43418,1000.);
#11940=VECTOR('',#43419,1000.);
#11941=VECTOR('',#43422,1000.);
#11942=VECTOR('',#43425,1000.);
#11943=VECTOR('',#43426,1000.);
#11944=VECTOR('',#43429,1000.);
#11945=VECTOR('',#43430,1000.);
#11946=VECTOR('',#43433,1000.);
#11947=VECTOR('',#43434,1000.);
#11948=VECTOR('',#43437,1000.);
#11949=VECTOR('',#43438,1000.);
#11950=VECTOR('',#43441,1000.);
#11951=VECTOR('',#43442,1000.);
#11952=VECTOR('',#43445,1000.);
#11953=VECTOR('',#43446,1000.);
#11954=VECTOR('',#43449,1000.);
#11955=VECTOR('',#43450,1000.);
#11956=VECTOR('',#43453,1000.);
#11957=VECTOR('',#43454,1000.);
#11958=VECTOR('',#43457,1000.);
#11959=VECTOR('',#43458,1000.);
#11960=VECTOR('',#43461,1000.);
#11961=VECTOR('',#43462,1000.);
#11962=VECTOR('',#43465,1000.);
#11963=VECTOR('',#43466,1000.);
#11964=VECTOR('',#43469,1000.);
#11965=VECTOR('',#43470,1000.);
#11966=VECTOR('',#43473,1000.);
#11967=VECTOR('',#43474,1000.);
#11968=VECTOR('',#43477,1000.);
#11969=VECTOR('',#43478,1000.);
#11970=VECTOR('',#43481,1000.);
#11971=VECTOR('',#43482,1000.);
#11972=VECTOR('',#43485,1000.);
#11973=VECTOR('',#43486,1000.);
#11974=VECTOR('',#43489,1000.);
#11975=VECTOR('',#43490,1000.);
#11976=VECTOR('',#43493,1000.);
#11977=VECTOR('',#43494,1000.);
#11978=VECTOR('',#43497,1000.);
#11979=VECTOR('',#43498,1000.);
#11980=VECTOR('',#43501,1000.);
#11981=VECTOR('',#43502,1000.);
#11982=VECTOR('',#43505,1000.);
#11983=VECTOR('',#43506,1000.);
#11984=VECTOR('',#43509,1000.);
#11985=VECTOR('',#43510,1000.);
#11986=VECTOR('',#43513,1000.);
#11987=VECTOR('',#43514,1000.);
#11988=VECTOR('',#43517,1000.);
#11989=VECTOR('',#43518,1000.);
#11990=VECTOR('',#43519,1000.);
#11991=VECTOR('',#43522,1000.);
#11992=VECTOR('',#43523,1000.);
#11993=VECTOR('',#43526,1000.);
#11994=VECTOR('',#43527,1000.);
#11995=VECTOR('',#43530,1000.);
#11996=VECTOR('',#43531,1000.);
#11997=VECTOR('',#43534,1000.);
#11998=VECTOR('',#43535,1000.);
#11999=VECTOR('',#43538,1000.);
#12000=VECTOR('',#43539,1000.);
#12001=VECTOR('',#43542,1000.);
#12002=VECTOR('',#43543,1000.);
#12003=VECTOR('',#43546,1000.);
#12004=VECTOR('',#43547,1000.);
#12005=VECTOR('',#43550,1000.);
#12006=VECTOR('',#43551,1000.);
#12007=VECTOR('',#43554,1000.);
#12008=VECTOR('',#43555,1000.);
#12009=VECTOR('',#43558,1000.);
#12010=VECTOR('',#43559,1000.);
#12011=VECTOR('',#43562,1000.);
#12012=VECTOR('',#43563,1000.);
#12013=VECTOR('',#43568,1000.);
#12014=VECTOR('',#43569,1000.);
#12015=VECTOR('',#43570,1000.);
#12016=VECTOR('',#43571,1000.);
#12017=VECTOR('',#43574,1000.);
#12018=VECTOR('',#43577,1000.);
#12019=VECTOR('',#43578,1000.);
#12020=VECTOR('',#43579,1000.);
#12021=VECTOR('',#43580,1000.);
#12022=VECTOR('',#43583,1000.);
#12023=VECTOR('',#43584,1000.);
#12024=VECTOR('',#43587,1000.);
#12025=VECTOR('',#43588,1000.);
#12026=VECTOR('',#43591,1000.);
#12027=VECTOR('',#43592,1000.);
#12028=VECTOR('',#43595,1000.);
#12029=VECTOR('',#43596,1000.);
#12030=VECTOR('',#43599,1000.);
#12031=VECTOR('',#43600,1000.);
#12032=VECTOR('',#43603,1000.);
#12033=VECTOR('',#43604,1000.);
#12034=VECTOR('',#43607,1000.);
#12035=VECTOR('',#43608,1000.);
#12036=VECTOR('',#43611,1000.);
#12037=VECTOR('',#43612,1000.);
#12038=VECTOR('',#43615,1000.);
#12039=VECTOR('',#43616,1000.);
#12040=VECTOR('',#43619,1000.);
#12041=VECTOR('',#43620,1000.);
#12042=VECTOR('',#43623,1000.);
#12043=VECTOR('',#43624,1000.);
#12044=VECTOR('',#43627,1000.);
#12045=VECTOR('',#43628,1000.);
#12046=VECTOR('',#43631,1000.);
#12047=VECTOR('',#43632,1000.);
#12048=VECTOR('',#43633,1000.);
#12049=VECTOR('',#43636,1000.);
#12050=VECTOR('',#43637,1000.);
#12051=VECTOR('',#43640,1000.);
#12052=VECTOR('',#43641,1000.);
#12053=VECTOR('',#43644,1000.);
#12054=VECTOR('',#43645,1000.);
#12055=VECTOR('',#43648,1000.);
#12056=VECTOR('',#43649,1000.);
#12057=VECTOR('',#43652,1000.);
#12058=VECTOR('',#43653,1000.);
#12059=VECTOR('',#43656,1000.);
#12060=VECTOR('',#43657,1000.);
#12061=VECTOR('',#43660,1000.);
#12062=VECTOR('',#43661,1000.);
#12063=VECTOR('',#43664,1000.);
#12064=VECTOR('',#43665,1000.);
#12065=VECTOR('',#43668,1000.);
#12066=VECTOR('',#43669,1000.);
#12067=VECTOR('',#43672,1000.);
#12068=VECTOR('',#43673,1000.);
#12069=VECTOR('',#43676,1000.);
#12070=VECTOR('',#43677,1000.);
#12071=VECTOR('',#43680,1000.);
#12072=VECTOR('',#43681,1000.);
#12073=VECTOR('',#43684,1000.);
#12074=VECTOR('',#43685,1000.);
#12075=VECTOR('',#43688,1000.);
#12076=VECTOR('',#43689,1000.);
#12077=VECTOR('',#43692,1000.);
#12078=VECTOR('',#43693,1000.);
#12079=VECTOR('',#43696,1000.);
#12080=VECTOR('',#43697,1000.);
#12081=VECTOR('',#43700,1000.);
#12082=VECTOR('',#43701,1000.);
#12083=VECTOR('',#43704,1000.);
#12084=VECTOR('',#43705,1000.);
#12085=VECTOR('',#43708,1000.);
#12086=VECTOR('',#43709,1000.);
#12087=VECTOR('',#43712,1000.);
#12088=VECTOR('',#43713,1000.);
#12089=VECTOR('',#43716,1000.);
#12090=VECTOR('',#43717,1000.);
#12091=VECTOR('',#43720,1000.);
#12092=VECTOR('',#43721,1000.);
#12093=VECTOR('',#43724,1000.);
#12094=VECTOR('',#43725,1000.);
#12095=VECTOR('',#43728,1000.);
#12096=VECTOR('',#43731,1000.);
#12097=VECTOR('',#43732,1000.);
#12098=VECTOR('',#43735,1000.);
#12099=VECTOR('',#43736,1000.);
#12100=VECTOR('',#43739,1000.);
#12101=VECTOR('',#43740,1000.);
#12102=VECTOR('',#43743,1000.);
#12103=VECTOR('',#43744,1000.);
#12104=VECTOR('',#43747,1000.);
#12105=VECTOR('',#43748,1000.);
#12106=VECTOR('',#43751,1000.);
#12107=VECTOR('',#43752,1000.);
#12108=VECTOR('',#43755,1000.);
#12109=VECTOR('',#43756,1000.);
#12110=VECTOR('',#43759,1000.);
#12111=VECTOR('',#43760,1000.);
#12112=VECTOR('',#43763,1000.);
#12113=VECTOR('',#43764,1000.);
#12114=VECTOR('',#43767,1000.);
#12115=VECTOR('',#43768,1000.);
#12116=VECTOR('',#43771,1000.);
#12117=VECTOR('',#43774,1000.);
#12118=VECTOR('',#43775,1000.);
#12119=VECTOR('',#43776,1000.);
#12120=VECTOR('',#43779,1000.);
#12121=VECTOR('',#43780,1000.);
#12122=VECTOR('',#43781,1000.);
#12123=VECTOR('',#43784,1000.);
#12124=VECTOR('',#43785,1000.);
#12125=VECTOR('',#43786,1000.);
#12126=VECTOR('',#43787,1000.);
#12127=VECTOR('',#43790,1000.);
#12128=VECTOR('',#43791,1000.);
#12129=VECTOR('',#43792,1000.);
#12130=VECTOR('',#43795,1000.);
#12131=VECTOR('',#43796,1000.);
#12132=VECTOR('',#43797,1000.);
#12133=VECTOR('',#43798,1000.);
#12134=VECTOR('',#43801,1000.);
#12135=VECTOR('',#43802,1000.);
#12136=VECTOR('',#43803,1000.);
#12137=VECTOR('',#43806,1000.);
#12138=VECTOR('',#43807,1000.);
#12139=VECTOR('',#43808,1000.);
#12140=VECTOR('',#43811,1000.);
#12141=VECTOR('',#43812,1000.);
#12142=VECTOR('',#43813,1000.);
#12143=VECTOR('',#43814,1000.);
#12144=VECTOR('',#43817,1000.);
#12145=VECTOR('',#43818,1000.);
#12146=VECTOR('',#43819,1000.);
#12147=VECTOR('',#43820,1000.);
#12148=VECTOR('',#43823,1000.);
#12149=VECTOR('',#43824,1000.);
#12150=VECTOR('',#43825,1000.);
#12151=VECTOR('',#43828,1000.);
#12152=VECTOR('',#43829,1000.);
#12153=VECTOR('',#43830,1000.);
#12154=VECTOR('',#43831,1000.);
#12155=VECTOR('',#43834,1000.);
#12156=VECTOR('',#43835,1000.);
#12157=VECTOR('',#43836,1000.);
#12158=VECTOR('',#43837,1000.);
#12159=VECTOR('',#43840,1000.);
#12160=VECTOR('',#43841,1000.);
#12161=VECTOR('',#43842,1000.);
#12162=VECTOR('',#43845,1000.);
#12163=VECTOR('',#43846,1000.);
#12164=VECTOR('',#43847,1000.);
#12165=VECTOR('',#43850,1000.);
#12166=VECTOR('',#43851,1000.);
#12167=VECTOR('',#43852,1000.);
#12168=VECTOR('',#43853,1000.);
#12169=VECTOR('',#43856,1000.);
#12170=VECTOR('',#43857,1000.);
#12171=VECTOR('',#43858,1000.);
#12172=VECTOR('',#43861,1000.);
#12173=VECTOR('',#43862,1000.);
#12174=VECTOR('',#43863,1000.);
#12175=VECTOR('',#43864,1000.);
#12176=VECTOR('',#43867,1000.);
#12177=VECTOR('',#43868,1000.);
#12178=VECTOR('',#43869,1000.);
#12179=VECTOR('',#43872,1000.);
#12180=VECTOR('',#43873,1000.);
#12181=VECTOR('',#43874,1000.);
#12182=VECTOR('',#43877,1000.);
#12183=VECTOR('',#43878,1000.);
#12184=VECTOR('',#43879,1000.);
#12185=VECTOR('',#43880,1000.);
#12186=VECTOR('',#43883,1000.);
#12187=VECTOR('',#43884,1000.);
#12188=VECTOR('',#43885,1000.);
#12189=VECTOR('',#43886,1000.);
#12190=VECTOR('',#43889,1000.);
#12191=VECTOR('',#43890,1000.);
#12192=VECTOR('',#43891,1000.);
#12193=VECTOR('',#43894,1000.);
#12194=VECTOR('',#43895,1000.);
#12195=VECTOR('',#43896,1000.);
#12196=VECTOR('',#43897,1000.);
#12197=VECTOR('',#43900,1000.);
#12198=VECTOR('',#43901,1000.);
#12199=VECTOR('',#43902,1000.);
#12200=VECTOR('',#43903,1000.);
#12201=VECTOR('',#43904,1000.);
#12202=VECTOR('',#43905,1000.);
#12203=VECTOR('',#43916,1000.);
#12204=VECTOR('',#43921,1000.);
#12205=VECTOR('',#43922,1000.);
#12206=VECTOR('',#43925,1000.);
#12207=VECTOR('',#43930,1000.);
#12208=VECTOR('',#43933,1000.);
#12209=VECTOR('',#43938,1000.);
#12210=VECTOR('',#43943,1000.);
#12211=VECTOR('',#43946,1000.);
#12212=VECTOR('',#43951,1000.);
#12213=VECTOR('',#43954,1000.);
#12214=VECTOR('',#43959,1000.);
#12215=VECTOR('',#44030,1000.);
#12216=VECTOR('',#44031,1000.);
#12217=VECTOR('',#44032,1000.);
#12218=VECTOR('',#44033,1000.);
#12219=VECTOR('',#44034,1000.);
#12220=VECTOR('',#44037,1000.);
#12221=VECTOR('',#44038,1000.);
#12222=VECTOR('',#44039,1000.);
#12223=VECTOR('',#44040,1000.);
#12224=VECTOR('',#44043,1000.);
#12225=VECTOR('',#44046,1000.);
#12226=VECTOR('',#44047,1000.);
#12227=VECTOR('',#44048,1000.);
#12228=VECTOR('',#44049,1000.);
#12229=VECTOR('',#44050,1000.);
#12230=VECTOR('',#44051,1000.);
#12231=VECTOR('',#44052,1000.);
#12232=VECTOR('',#44055,1000.);
#12233=VECTOR('',#44058,1000.);
#12234=VECTOR('',#44061,1000.);
#12235=VECTOR('',#44064,1000.);
#12236=VECTOR('',#44067,1000.);
#12237=VECTOR('',#44070,1000.);
#12238=VECTOR('',#44073,1000.);
#12239=VECTOR('',#44074,1000.);
#12240=VECTOR('',#44075,1000.);
#12241=VECTOR('',#44076,1000.);
#12242=VECTOR('',#44077,1000.);
#12243=VECTOR('',#44078,1000.);
#12244=VECTOR('',#44081,1000.);
#12245=VECTOR('',#44084,1000.);
#12246=VECTOR('',#44085,1000.);
#12247=VECTOR('',#44086,1000.);
#12248=VECTOR('',#44087,1000.);
#12249=VECTOR('',#44088,1000.);
#12250=VECTOR('',#44089,1000.);
#12251=VECTOR('',#44092,1000.);
#12252=VECTOR('',#44095,1000.);
#12253=VECTOR('',#44098,1000.);
#12254=VECTOR('',#44101,1000.);
#12255=VECTOR('',#44104,1000.);
#12256=VECTOR('',#44109,10.);
#12257=VECTOR('',#44110,1000.);
#12258=VECTOR('',#44111,10.);
#12259=VECTOR('',#44116,10.);
#12260=VECTOR('',#44117,1000.);
#12261=VECTOR('',#44118,10.);
#12262=VECTOR('',#44123,10.);
#12263=VECTOR('',#44124,1000.);
#12264=VECTOR('',#44125,10.);
#12265=VECTOR('',#44130,10.);
#12266=VECTOR('',#44131,1000.);
#12267=VECTOR('',#44132,10.);
#12268=VECTOR('',#44135,10.);
#12269=VECTOR('',#44136,10.);
#12270=VECTOR('',#44137,10.);
#12271=VECTOR('',#44138,10.);
#12272=VECTOR('',#44145,1000.);
#12273=VECTOR('',#44146,1000.);
#12274=VECTOR('',#44149,1000.);
#12275=VECTOR('',#44152,1000.);
#12276=VECTOR('',#44153,1000.);
#12277=VECTOR('',#44156,1000.);
#12278=VECTOR('',#44157,1000.);
#12279=VECTOR('',#44160,1000.);
#12280=VECTOR('',#44165,10.);
#12281=VECTOR('',#44166,10.);
#12282=VECTOR('',#44167,10.);
#12283=VECTOR('',#44168,10.);
#12284=VECTOR('',#44175,1000.);
#12285=VECTOR('',#44176,1000.);
#12286=VECTOR('',#44179,1000.);
#12287=VECTOR('',#44182,1000.);
#12288=VECTOR('',#44183,1000.);
#12289=VECTOR('',#44186,1000.);
#12290=VECTOR('',#44187,1000.);
#12291=VECTOR('',#44190,1000.);
#12292=VECTOR('',#44211,1000.);
#12293=VECTOR('',#44218,1000.);
#12294=VECTOR('',#44225,1000.);
#12295=VECTOR('',#44228,1000.);
#12296=VECTOR('',#44231,1000.);
#12297=VECTOR('',#44234,1000.);
#12298=VECTOR('',#44237,1000.);
#12299=VECTOR('',#44240,1000.);
#12300=VECTOR('',#44245,1000.);
#12301=VECTOR('',#44248,1000.);
#12302=VECTOR('',#44251,1000.);
#12303=VECTOR('',#44254,1000.);
#12304=VECTOR('',#44257,1000.);
#12305=VECTOR('',#44260,1000.);
#12306=VECTOR('',#44263,1000.);
#12307=VECTOR('',#44264,1000.);
#12308=VECTOR('',#44267,1000.);
#12309=VECTOR('',#44268,1000.);
#12310=VECTOR('',#44277,1000.);
#12311=VECTOR('',#44278,1000.);
#12312=VECTOR('',#44281,1000.);
#12313=VECTOR('',#44282,1000.);
#12314=VECTOR('',#44285,1000.);
#12315=VECTOR('',#44288,1000.);
#12316=VECTOR('',#44311,1000.);
#12317=VECTOR('',#44318,1000.);
#12318=VECTOR('',#44325,1000.);
#12319=VECTOR('',#44328,1000.);
#12320=VECTOR('',#44331,1000.);
#12321=VECTOR('',#44334,1000.);
#12322=VECTOR('',#44337,1000.);
#12323=VECTOR('',#44340,1000.);
#12324=VECTOR('',#44345,1000.);
#12325=VECTOR('',#44348,1000.);
#12326=VECTOR('',#44351,1000.);
#12327=VECTOR('',#44354,1000.);
#12328=VECTOR('',#44357,1000.);
#12329=VECTOR('',#44360,1000.);
#12330=VECTOR('',#44363,1000.);
#12331=VECTOR('',#44364,1000.);
#12332=VECTOR('',#44367,1000.);
#12333=VECTOR('',#44368,1000.);
#12334=VECTOR('',#44377,1000.);
#12335=VECTOR('',#44378,1000.);
#12336=VECTOR('',#44381,1000.);
#12337=VECTOR('',#44382,1000.);
#12338=VECTOR('',#44385,1000.);
#12339=VECTOR('',#44388,1000.);
#12340=VECTOR('',#44411,1000.);
#12341=VECTOR('',#44418,1000.);
#12342=VECTOR('',#44425,1000.);
#12343=VECTOR('',#44428,1000.);
#12344=VECTOR('',#44431,1000.);
#12345=VECTOR('',#44434,1000.);
#12346=VECTOR('',#44437,1000.);
#12347=VECTOR('',#44440,1000.);
#12348=VECTOR('',#44445,1000.);
#12349=VECTOR('',#44448,1000.);
#12350=VECTOR('',#44451,1000.);
#12351=VECTOR('',#44454,1000.);
#12352=VECTOR('',#44457,1000.);
#12353=VECTOR('',#44460,1000.);
#12354=VECTOR('',#44463,1000.);
#12355=VECTOR('',#44464,1000.);
#12356=VECTOR('',#44467,1000.);
#12357=VECTOR('',#44468,1000.);
#12358=VECTOR('',#44477,1000.);
#12359=VECTOR('',#44478,1000.);
#12360=VECTOR('',#44481,1000.);
#12361=VECTOR('',#44482,1000.);
#12362=VECTOR('',#44485,1000.);
#12363=VECTOR('',#44488,1000.);
#12364=VECTOR('',#44511,1000.);
#12365=VECTOR('',#44518,1000.);
#12366=VECTOR('',#44525,1000.);
#12367=VECTOR('',#44528,1000.);
#12368=VECTOR('',#44531,1000.);
#12369=VECTOR('',#44534,1000.);
#12370=VECTOR('',#44537,1000.);
#12371=VECTOR('',#44540,1000.);
#12372=VECTOR('',#44545,1000.);
#12373=VECTOR('',#44548,1000.);
#12374=VECTOR('',#44551,1000.);
#12375=VECTOR('',#44554,1000.);
#12376=VECTOR('',#44557,1000.);
#12377=VECTOR('',#44560,1000.);
#12378=VECTOR('',#44563,1000.);
#12379=VECTOR('',#44564,1000.);
#12380=VECTOR('',#44567,1000.);
#12381=VECTOR('',#44568,1000.);
#12382=VECTOR('',#44577,1000.);
#12383=VECTOR('',#44578,1000.);
#12384=VECTOR('',#44581,1000.);
#12385=VECTOR('',#44582,1000.);
#12386=VECTOR('',#44585,1000.);
#12387=VECTOR('',#44588,1000.);
#12388=VECTOR('',#44601,1000.);
#12389=VECTOR('',#44606,1000.);
#12390=VECTOR('',#44609,1000.);
#12391=VECTOR('',#44614,1000.);
#12392=VECTOR('',#44617,1000.);
#12393=VECTOR('',#44622,1000.);
#12394=VECTOR('',#44627,1000.);
#12395=VECTOR('',#44630,1000.);
#12396=VECTOR('',#44635,1000.);
#12397=VECTOR('',#44636,1000.);
#12398=VECTOR('',#44641,1000.);
#12399=VECTOR('',#44716,1000.);
#12400=VECTOR('',#44717,1000.);
#12401=VECTOR('',#44720,1000.);
#12402=VECTOR('',#44723,1000.);
#12403=VECTOR('',#44724,1000.);
#12404=VECTOR('',#44727,1000.);
#12405=VECTOR('',#44730,1000.);
#12406=VECTOR('',#44731,1000.);
#12407=VECTOR('',#44734,1000.);
#12408=VECTOR('',#44737,1000.);
#12409=VECTOR('',#44740,1000.);
#12410=VECTOR('',#44741,1000.);
#12411=VECTOR('',#44744,1000.);
#12412=VECTOR('',#44745,1000.);
#12413=VECTOR('',#44748,1000.);
#12414=VECTOR('',#44751,1000.);
#12415=VECTOR('',#44752,1000.);
#12416=VECTOR('',#44755,1000.);
#12417=VECTOR('',#44756,1000.);
#12418=VECTOR('',#44757,1000.);
#12419=VECTOR('',#44758,1000.);
#12420=VECTOR('',#44759,1000.);
#12421=VECTOR('',#44760,1000.);
#12422=VECTOR('',#44761,1000.);
#12423=VECTOR('',#44762,1000.);
#12424=VECTOR('',#44763,1000.);
#12425=VECTOR('',#44764,1000.);
#12426=VECTOR('',#44765,1000.);
#12427=VECTOR('',#44766,1000.);
#12428=VECTOR('',#44767,1000.);
#12429=VECTOR('',#44768,1000.);
#12430=VECTOR('',#44769,1000.);
#12431=VECTOR('',#44770,1000.);
#12432=VECTOR('',#44771,1000.);
#12433=VECTOR('',#44772,1000.);
#12434=VECTOR('',#44773,1000.);
#12435=VECTOR('',#44774,1000.);
#12436=VECTOR('',#44775,1000.);
#12437=VECTOR('',#44776,1000.);
#12438=VECTOR('',#44777,1000.);
#12439=VECTOR('',#44778,1000.);
#12440=VECTOR('',#44779,1000.);
#12441=VECTOR('',#44780,1000.);
#12442=VECTOR('',#44781,1000.);
#12443=VECTOR('',#44782,1000.);
#12444=VECTOR('',#44783,1000.);
#12445=VECTOR('',#44784,1000.);
#12446=VECTOR('',#44785,1000.);
#12447=VECTOR('',#44786,1000.);
#12448=VECTOR('',#44787,1000.);
#12449=VECTOR('',#44788,1000.);
#12450=VECTOR('',#44789,1000.);
#12451=VECTOR('',#44790,1000.);
#12452=VECTOR('',#44791,1000.);
#12453=VECTOR('',#44792,1000.);
#12454=VECTOR('',#44793,1000.);
#12455=VECTOR('',#44794,1000.);
#12456=VECTOR('',#44795,1000.);
#12457=VECTOR('',#44796,1000.);
#12458=VECTOR('',#44797,1000.);
#12459=VECTOR('',#44908,1000.);
#12460=VECTOR('',#44909,1000.);
#12461=VECTOR('',#44912,1000.);
#12462=VECTOR('',#44915,1000.);
#12463=VECTOR('',#44918,1000.);
#12464=VECTOR('',#44921,1000.);
#12465=VECTOR('',#44924,1000.);
#12466=VECTOR('',#44927,1000.);
#12467=VECTOR('',#44930,1000.);
#12468=VECTOR('',#44933,1000.);
#12469=VECTOR('',#44936,1000.);
#12470=VECTOR('',#44939,1000.);
#12471=VECTOR('',#44944,1000.);
#12472=VECTOR('',#44945,1000.);
#12473=VECTOR('',#44948,1000.);
#12474=VECTOR('',#44951,1000.);
#12475=VECTOR('',#44964,1000.);
#12476=VECTOR('',#44967,1000.);
#12477=VECTOR('',#44972,1000.);
#12478=VECTOR('',#44975,1000.);
#12479=VECTOR('',#44980,1000.);
#12480=VECTOR('',#44983,1000.);
#12481=VECTOR('',#44988,1000.);
#12482=VECTOR('',#44991,1000.);
#12483=VECTOR('',#44996,1000.);
#12484=VECTOR('',#44999,1000.);
#12485=VECTOR('',#45004,1000.);
#12486=VECTOR('',#45007,1000.);
#12487=VECTOR('',#45012,1000.);
#12488=VECTOR('',#45015,1000.);
#12489=VECTOR('',#45020,1000.);
#12490=VECTOR('',#45023,1000.);
#12491=VECTOR('',#45028,1000.);
#12492=VECTOR('',#45031,1000.);
#12493=VECTOR('',#45036,1000.);
#12494=VECTOR('',#45039,1000.);
#12495=VECTOR('',#45044,1000.);
#12496=VECTOR('',#45047,1000.);
#12497=VECTOR('',#45052,1000.);
#12498=VECTOR('',#45055,1000.);
#12499=VECTOR('',#45060,1000.);
#12500=VECTOR('',#45063,1000.);
#12501=VECTOR('',#45068,1000.);
#12502=VECTOR('',#45071,1000.);
#12503=VECTOR('',#45076,1000.);
#12504=VECTOR('',#45079,1000.);
#12505=VECTOR('',#45084,1000.);
#12506=VECTOR('',#45087,1000.);
#12507=VECTOR('',#45092,1000.);
#12508=VECTOR('',#45095,1000.);
#12509=VECTOR('',#45100,1000.);
#12510=VECTOR('',#45103,1000.);
#12511=VECTOR('',#45108,1000.);
#12512=VECTOR('',#45111,1000.);
#12513=VECTOR('',#45116,1000.);
#12514=VECTOR('',#45119,1000.);
#12515=VECTOR('',#45124,1000.);
#12516=VECTOR('',#45127,1000.);
#12517=VECTOR('',#45132,1000.);
#12518=VECTOR('',#45135,1000.);
#12519=VECTOR('',#45140,1000.);
#12520=VECTOR('',#45143,1000.);
#12521=VECTOR('',#45148,1000.);
#12522=VECTOR('',#45151,1000.);
#12523=VECTOR('',#45156,1000.);
#12524=VECTOR('',#45159,1000.);
#12525=VECTOR('',#45164,1000.);
#12526=VECTOR('',#45167,1000.);
#12527=VECTOR('',#45172,1000.);
#12528=VECTOR('',#45175,1000.);
#12529=VECTOR('',#45180,1000.);
#12530=VECTOR('',#45183,1000.);
#12531=VECTOR('',#45188,1000.);
#12532=VECTOR('',#45191,1000.);
#12533=VECTOR('',#45196,1000.);
#12534=VECTOR('',#45199,1000.);
#12535=VECTOR('',#45204,1000.);
#12536=VECTOR('',#45207,1000.);
#12537=VECTOR('',#45212,1000.);
#12538=VECTOR('',#45215,1000.);
#12539=VECTOR('',#45220,1000.);
#12540=VECTOR('',#45223,1000.);
#12541=VECTOR('',#45228,1000.);
#12542=VECTOR('',#45231,1000.);
#12543=VECTOR('',#45236,1000.);
#12544=VECTOR('',#45239,1000.);
#12545=VECTOR('',#45244,1000.);
#12546=VECTOR('',#45247,1000.);
#12547=VECTOR('',#45252,1000.);
#12548=VECTOR('',#45255,1000.);
#12549=VECTOR('',#45260,1000.);
#12550=VECTOR('',#45263,1000.);
#12551=VECTOR('',#45268,1000.);
#12552=VECTOR('',#45271,1000.);
#12553=VECTOR('',#45276,1000.);
#12554=VECTOR('',#45279,1000.);
#12555=VECTOR('',#45284,1000.);
#12556=VECTOR('',#45287,1000.);
#12557=VECTOR('',#45292,1000.);
#12558=VECTOR('',#45295,1000.);
#12559=VECTOR('',#45300,1000.);
#12560=VECTOR('',#45303,1000.);
#12561=VECTOR('',#45308,1000.);
#12562=VECTOR('',#45311,1000.);
#12563=VECTOR('',#45316,1000.);
#12564=VECTOR('',#45319,1000.);
#12565=VECTOR('',#45324,1000.);
#12566=VECTOR('',#45327,1000.);
#12567=VECTOR('',#45332,1000.);
#12568=VECTOR('',#45335,1000.);
#12569=VECTOR('',#45340,1000.);
#12570=VECTOR('',#45343,1000.);
#12571=VECTOR('',#45348,1000.);
#12572=VECTOR('',#45351,1000.);
#12573=VECTOR('',#45354,1000.);
#12574=VECTOR('',#45357,1000.);
#12575=VECTOR('',#45358,1000.);
#12576=VECTOR('',#45361,1000.);
#12577=VECTOR('',#45366,1000.);
#12578=VECTOR('',#45375,1000.);
#12579=VECTOR('',#45384,1000.);
#12580=VECTOR('',#45387,1000.);
#12581=VECTOR('',#45390,1000.);
#12582=VECTOR('',#45393,1000.);
#12583=VECTOR('',#45412,1000.);
#12584=VECTOR('',#45419,1000.);
#12585=VECTOR('',#45426,1000.);
#12586=VECTOR('',#45429,1000.);
#12587=VECTOR('',#45432,1000.);
#12588=VECTOR('',#45435,1000.);
#12589=VECTOR('',#45438,1000.);
#12590=VECTOR('',#45441,1000.);
#12591=VECTOR('',#45446,1000.);
#12592=VECTOR('',#45449,1000.);
#12593=VECTOR('',#45452,1000.);
#12594=VECTOR('',#45455,1000.);
#12595=VECTOR('',#45458,1000.);
#12596=VECTOR('',#45461,1000.);
#12597=VECTOR('',#45464,1000.);
#12598=VECTOR('',#45465,1000.);
#12599=VECTOR('',#45468,1000.);
#12600=VECTOR('',#45469,1000.);
#12601=VECTOR('',#45478,1000.);
#12602=VECTOR('',#45479,1000.);
#12603=VECTOR('',#45482,1000.);
#12604=VECTOR('',#45483,1000.);
#12605=VECTOR('',#45486,1000.);
#12606=VECTOR('',#45489,1000.);
#12607=VECTOR('',#45512,1000.);
#12608=VECTOR('',#45519,1000.);
#12609=VECTOR('',#45526,1000.);
#12610=VECTOR('',#45529,1000.);
#12611=VECTOR('',#45532,1000.);
#12612=VECTOR('',#45535,1000.);
#12613=VECTOR('',#45538,1000.);
#12614=VECTOR('',#45541,1000.);
#12615=VECTOR('',#45546,1000.);
#12616=VECTOR('',#45549,1000.);
#12617=VECTOR('',#45552,1000.);
#12618=VECTOR('',#45555,1000.);
#12619=VECTOR('',#45558,1000.);
#12620=VECTOR('',#45561,1000.);
#12621=VECTOR('',#45564,1000.);
#12622=VECTOR('',#45565,1000.);
#12623=VECTOR('',#45568,1000.);
#12624=VECTOR('',#45569,1000.);
#12625=VECTOR('',#45578,1000.);
#12626=VECTOR('',#45579,1000.);
#12627=VECTOR('',#45582,1000.);
#12628=VECTOR('',#45583,1000.);
#12629=VECTOR('',#45586,1000.);
#12630=VECTOR('',#45589,1000.);
#12631=VECTOR('',#45598,1000.);
#12632=VECTOR('',#45601,1000.);
#12633=VECTOR('',#45604,1000.);
#12634=VECTOR('',#45607,1000.);
#12635=VECTOR('',#45608,1000.);
#12636=VECTOR('',#45611,1000.);
#12637=VECTOR('',#45616,1000.);
#12638=VECTOR('',#45625,1000.);
#12639=VECTOR('',#45630,1000.);
#12640=VECTOR('',#45633,1000.);
#12641=VECTOR('',#45636,1000.);
#12642=VECTOR('',#45637,1000.);
#12643=VECTOR('',#45638,1000.);
#12644=VECTOR('',#45641,1000.);
#12645=VECTOR('',#45642,1000.);
#12646=VECTOR('',#45643,1000.);
#12647=VECTOR('',#45648,1000.);
#12648=VECTOR('',#45655,1000.);
#12649=VECTOR('',#45660,1000.);
#12650=VECTOR('',#45663,1000.);
#16490=CIRCLE('',#39986,1.75);
#16491=CIRCLE('',#39987,1.75);
#16492=CIRCLE('',#39989,1.75);
#16493=CIRCLE('',#39990,1.75);
#16494=CIRCLE('',#39992,1.75);
#16495=CIRCLE('',#39993,1.75);
#16496=CIRCLE('',#39995,1.75);
#16497=CIRCLE('',#39996,1.75);
#16498=CIRCLE('',#39998,1.25);
#16499=CIRCLE('',#39999,1.25);
#16500=CIRCLE('',#40001,1.25);
#16501=CIRCLE('',#40002,1.25);
#16502=CIRCLE('',#40004,1.5);
#16503=CIRCLE('',#40005,1.5);
#16504=CIRCLE('',#40007,1.5);
#16505=CIRCLE('',#40008,1.5);
#16506=CIRCLE('',#40010,1.5);
#16507=CIRCLE('',#40011,1.5);
#16508=CIRCLE('',#40013,1.5);
#16509=CIRCLE('',#40014,1.5);
#16510=CIRCLE('',#40016,1.5);
#16511=CIRCLE('',#40017,1.5);
#16512=CIRCLE('',#40019,1.5);
#16513=CIRCLE('',#40020,1.5);
#16514=CIRCLE('',#40022,1.5);
#16515=CIRCLE('',#40023,1.5);
#16516=CIRCLE('',#40025,1.5);
#16517=CIRCLE('',#40026,1.5);
#16518=CIRCLE('',#40028,1.5);
#16519=CIRCLE('',#40029,1.5);
#16520=CIRCLE('',#40031,1.5);
#16521=CIRCLE('',#40032,1.5);
#16522=CIRCLE('',#40034,1.5);
#16523=CIRCLE('',#40035,1.5);
#16524=CIRCLE('',#40037,1.5);
#16525=CIRCLE('',#40038,1.5);
#16526=CIRCLE('',#40040,1.5);
#16527=CIRCLE('',#40041,1.5);
#16528=CIRCLE('',#40043,1.5);
#16529=CIRCLE('',#40044,1.5);
#16530=CIRCLE('',#40046,1.5);
#16531=CIRCLE('',#40047,1.5);
#16532=CIRCLE('',#40049,1.5);
#16533=CIRCLE('',#40050,1.5);
#16534=CIRCLE('',#40052,1.5);
#16535=CIRCLE('',#40053,1.5);
#16536=CIRCLE('',#40055,1.5);
#16537=CIRCLE('',#40056,1.5);
#16538=CIRCLE('',#40058,1.5);
#16539=CIRCLE('',#40059,1.5);
#16540=CIRCLE('',#40061,1.5);
#16541=CIRCLE('',#40062,1.5);
#16542=CIRCLE('',#40064,1.5);
#16543=CIRCLE('',#40065,1.5);
#16544=CIRCLE('',#40067,1.5);
#16545=CIRCLE('',#40068,1.5);
#16546=CIRCLE('',#40070,1.5);
#16547=CIRCLE('',#40071,1.5);
#16548=CIRCLE('',#40073,1.5);
#16549=CIRCLE('',#40074,1.5);
#16550=CIRCLE('',#40076,1.5);
#16551=CIRCLE('',#40077,1.5);
#16552=CIRCLE('',#40079,1.5);
#16553=CIRCLE('',#40080,1.5);
#16554=CIRCLE('',#40082,1.5);
#16555=CIRCLE('',#40083,1.5);
#16556=CIRCLE('',#40085,1.5);
#16557=CIRCLE('',#40086,1.5);
#16558=CIRCLE('',#40088,1.5);
#16559=CIRCLE('',#40089,1.5);
#16560=CIRCLE('',#40091,1.5);
#16561=CIRCLE('',#40092,1.5);
#16562=CIRCLE('',#40094,1.5);
#16563=CIRCLE('',#40095,1.5);
#16564=CIRCLE('',#40097,1.5);
#16565=CIRCLE('',#40098,1.5);
#16566=CIRCLE('',#40100,1.5);
#16567=CIRCLE('',#40101,1.5);
#16568=CIRCLE('',#40103,1.5);
#16569=CIRCLE('',#40104,1.5);
#16570=CIRCLE('',#40106,1.5);
#16571=CIRCLE('',#40107,1.5);
#16572=CIRCLE('',#40109,1.5);
#16573=CIRCLE('',#40110,1.5);
#16574=CIRCLE('',#40112,1.5);
#16575=CIRCLE('',#40113,1.5);
#16576=CIRCLE('',#40115,1.5);
#16577=CIRCLE('',#40116,1.5);
#16578=CIRCLE('',#40118,1.5);
#16579=CIRCLE('',#40119,1.5);
#16580=CIRCLE('',#40121,1.5);
#16581=CIRCLE('',#40122,1.5);
#16582=CIRCLE('',#40124,1.5);
#16583=CIRCLE('',#40125,1.5);
#16584=CIRCLE('',#40127,1.5);
#16585=CIRCLE('',#40128,1.5);
#16586=CIRCLE('',#40130,1.5);
#16587=CIRCLE('',#40131,1.5);
#16588=CIRCLE('',#40133,1.5);
#16589=CIRCLE('',#40134,1.5);
#16590=CIRCLE('',#40136,1.5);
#16591=CIRCLE('',#40137,1.5);
#16592=CIRCLE('',#40139,1.5);
#16593=CIRCLE('',#40140,1.5);
#16594=CIRCLE('',#40142,1.5);
#16595=CIRCLE('',#40143,1.5);
#16596=CIRCLE('',#40145,1.5);
#16597=CIRCLE('',#40146,1.5);
#16598=CIRCLE('',#40148,1.5);
#16599=CIRCLE('',#40149,1.5);
#16600=CIRCLE('',#40151,1.5);
#16601=CIRCLE('',#40152,1.5);
#16602=CIRCLE('',#40154,1.5);
#16603=CIRCLE('',#40155,1.5);
#16604=CIRCLE('',#40157,1.5);
#16605=CIRCLE('',#40158,1.5);
#16606=CIRCLE('',#40160,1.5);
#16607=CIRCLE('',#40161,1.5);
#16608=CIRCLE('',#40163,1.5);
#16609=CIRCLE('',#40164,1.5);
#16610=CIRCLE('',#40166,1.5);
#16611=CIRCLE('',#40167,1.5);
#16612=CIRCLE('',#40169,1.5);
#16613=CIRCLE('',#40170,1.5);
#16614=CIRCLE('',#40172,1.5);
#16615=CIRCLE('',#40173,1.5);
#16616=CIRCLE('',#40175,1.5);
#16617=CIRCLE('',#40176,1.5);
#16618=CIRCLE('',#40178,1.5);
#16619=CIRCLE('',#40179,1.5);
#16620=CIRCLE('',#40181,1.5);
#16621=CIRCLE('',#40182,1.5);
#16622=CIRCLE('',#40184,1.5);
#16623=CIRCLE('',#40185,1.5);
#16624=CIRCLE('',#40187,1.5);
#16625=CIRCLE('',#40188,1.5);
#16626=CIRCLE('',#40190,1.5);
#16627=CIRCLE('',#40191,1.5);
#16628=CIRCLE('',#40193,1.5);
#16629=CIRCLE('',#40194,1.5);
#16630=CIRCLE('',#40196,1.5);
#16631=CIRCLE('',#40197,1.5);
#16632=CIRCLE('',#40199,1.5);
#16633=CIRCLE('',#40200,1.5);
#16634=CIRCLE('',#40202,1.74999999999999);
#16635=CIRCLE('',#40203,1.74999999999999);
#16636=CIRCLE('',#40205,1.74999999999998);
#16637=CIRCLE('',#40206,1.74999999999998);
#16638=CIRCLE('',#40208,1.75);
#16639=CIRCLE('',#40209,1.75);
#16640=CIRCLE('',#40211,1.75);
#16641=CIRCLE('',#40212,1.75);
#16642=CIRCLE('',#40214,42.4898979485563);
#16643=CIRCLE('',#40215,0.5);
#16644=CIRCLE('',#40216,42.);
#16645=CIRCLE('',#40218,43.2737346662473);
#16646=CIRCLE('',#40219,1.2);
#16647=CIRCLE('',#40220,44.4494897427832);
#16648=CIRCLE('',#40222,42.);
#16649=CIRCLE('',#40223,1.3);
#16650=CIRCLE('',#40225,44.4494897427832);
#16651=CIRCLE('',#40226,2.);
#16652=CIRCLE('',#40228,1.25);
#16653=CIRCLE('',#40229,1.25);
#16654=CIRCLE('',#40231,1.25);
#16655=CIRCLE('',#40232,1.25);
#16656=CIRCLE('',#40234,1.25);
#16657=CIRCLE('',#40235,1.25);
#16658=CIRCLE('',#40237,1.25);
#16659=CIRCLE('',#40238,1.25);
#16660=CIRCLE('',#40240,1.5);
#16661=CIRCLE('',#40241,1.5);
#16662=CIRCLE('',#40242,1.5);
#16663=CIRCLE('',#40243,1.5);
#16664=CIRCLE('',#40245,1.5);
#16665=CIRCLE('',#40246,1.5);
#16666=CIRCLE('',#40247,1.5);
#16667=CIRCLE('',#40248,1.5);
#16668=CIRCLE('',#40252,4.);
#16669=CIRCLE('',#40253,4.);
#16670=CIRCLE('',#40255,4.);
#16671=CIRCLE('',#40256,4.);
#16672=CIRCLE('',#40260,1.5);
#16673=CIRCLE('',#40261,1.5);
#16674=CIRCLE('',#40262,1.5);
#16675=CIRCLE('',#40263,1.5);
#16676=CIRCLE('',#40264,1.5);
#16677=CIRCLE('',#40265,1.5);
#16678=CIRCLE('',#40266,1.5);
#16679=CIRCLE('',#40267,1.5);
#16680=CIRCLE('',#40268,1.5);
#16681=CIRCLE('',#40269,1.5);
#16682=CIRCLE('',#40270,1.5);
#16683=CIRCLE('',#40271,1.5);
#16684=CIRCLE('',#40272,1.5);
#16685=CIRCLE('',#40273,1.5);
#16686=CIRCLE('',#40274,1.5);
#16687=CIRCLE('',#40275,1.5);
#16688=CIRCLE('',#40276,1.5);
#16689=CIRCLE('',#40277,1.5);
#16690=CIRCLE('',#40278,1.5);
#16691=CIRCLE('',#40279,1.5);
#16692=CIRCLE('',#40280,1.5);
#16693=CIRCLE('',#40281,1.5);
#16694=CIRCLE('',#40282,1.5);
#16695=CIRCLE('',#40283,1.5);
#16696=CIRCLE('',#40284,1.5);
#16697=CIRCLE('',#40285,1.5);
#16698=CIRCLE('',#40286,1.5);
#16699=CIRCLE('',#40287,1.5);
#16700=CIRCLE('',#40288,1.5);
#16701=CIRCLE('',#40289,1.5);
#16702=CIRCLE('',#40290,1.5);
#16703=CIRCLE('',#40291,1.5);
#16704=CIRCLE('',#40292,1.5);
#16705=CIRCLE('',#40293,1.5);
#16706=CIRCLE('',#40294,1.5);
#16707=CIRCLE('',#40295,1.5);
#16708=CIRCLE('',#40296,1.5);
#16709=CIRCLE('',#40297,1.5);
#16710=CIRCLE('',#40298,1.5);
#16711=CIRCLE('',#40299,1.5);
#16712=CIRCLE('',#40300,1.5);
#16713=CIRCLE('',#40301,1.5);
#16714=CIRCLE('',#40302,1.5);
#16715=CIRCLE('',#40303,1.5);
#16716=CIRCLE('',#40304,1.5);
#16717=CIRCLE('',#40305,1.5);
#16718=CIRCLE('',#40306,1.5);
#16719=CIRCLE('',#40307,1.5);
#16720=CIRCLE('',#40308,1.5);
#16721=CIRCLE('',#40309,1.5);
#16722=CIRCLE('',#40311,1.5);
#16723=CIRCLE('',#40312,1.5);
#16724=CIRCLE('',#40313,1.5);
#16725=CIRCLE('',#40314,1.5);
#16726=CIRCLE('',#40315,1.5);
#16727=CIRCLE('',#40316,1.5);
#16728=CIRCLE('',#40317,1.5);
#16729=CIRCLE('',#40318,1.5);
#16730=CIRCLE('',#40319,1.5);
#16731=CIRCLE('',#40320,1.5);
#16732=CIRCLE('',#40321,1.5);
#16733=CIRCLE('',#40322,1.5);
#16734=CIRCLE('',#40323,1.5);
#16735=CIRCLE('',#40324,1.5);
#16736=CIRCLE('',#40325,1.5);
#16737=CIRCLE('',#40326,1.5);
#16738=CIRCLE('',#40327,1.5);
#16739=CIRCLE('',#40328,1.5);
#16740=CIRCLE('',#40329,1.5);
#16741=CIRCLE('',#40330,1.5);
#16742=CIRCLE('',#40331,1.5);
#16743=CIRCLE('',#40332,1.5);
#16744=CIRCLE('',#40333,1.5);
#16745=CIRCLE('',#40334,1.5);
#16746=CIRCLE('',#40335,1.5);
#16747=CIRCLE('',#40336,1.5);
#16748=CIRCLE('',#40337,1.5);
#16749=CIRCLE('',#40338,1.5);
#16750=CIRCLE('',#40339,1.5);
#16751=CIRCLE('',#40340,1.5);
#16752=CIRCLE('',#40341,1.5);
#16753=CIRCLE('',#40342,1.5);
#16754=CIRCLE('',#40343,1.5);
#16755=CIRCLE('',#40344,1.5);
#16756=CIRCLE('',#40345,1.5);
#16757=CIRCLE('',#40346,1.5);
#16758=CIRCLE('',#40347,1.5);
#16759=CIRCLE('',#40348,1.5);
#16760=CIRCLE('',#40349,1.5);
#16761=CIRCLE('',#40350,1.5);
#16762=CIRCLE('',#40351,1.5);
#16763=CIRCLE('',#40352,1.5);
#16764=CIRCLE('',#40353,1.5);
#16765=CIRCLE('',#40354,1.5);
#16766=CIRCLE('',#40355,1.5);
#16767=CIRCLE('',#40356,1.5);
#16768=CIRCLE('',#40357,1.5);
#16769=CIRCLE('',#40358,1.5);
#16770=CIRCLE('',#40359,1.5);
#16771=CIRCLE('',#40360,1.5);
#16772=CIRCLE('',#40386,1.5);
#16773=CIRCLE('',#40387,1.5);
#16774=CIRCLE('',#40388,1.5);
#16775=CIRCLE('',#40389,1.5);
#16776=CIRCLE('',#40390,1.5);
#16777=CIRCLE('',#40391,1.5);
#16778=CIRCLE('',#40392,1.5);
#16779=CIRCLE('',#40393,1.5);
#16780=CIRCLE('',#40394,1.5);
#16781=CIRCLE('',#40395,1.5);
#16782=CIRCLE('',#40396,1.5);
#16783=CIRCLE('',#40397,1.5);
#16784=CIRCLE('',#40398,1.5);
#16785=CIRCLE('',#40399,1.5);
#16786=CIRCLE('',#40400,1.5);
#16787=CIRCLE('',#40401,1.5);
#16788=CIRCLE('',#40402,1.5);
#16789=CIRCLE('',#40403,1.5);
#16790=CIRCLE('',#40404,1.5);
#16791=CIRCLE('',#40405,1.5);
#16792=CIRCLE('',#40406,1.5);
#16793=CIRCLE('',#40407,1.5);
#16794=CIRCLE('',#40408,1.5);
#16795=CIRCLE('',#40409,1.5);
#16796=CIRCLE('',#40410,1.5);
#16797=CIRCLE('',#40411,1.5);
#16798=CIRCLE('',#40412,1.5);
#16799=CIRCLE('',#40413,1.5);
#16800=CIRCLE('',#40414,1.5);
#16801=CIRCLE('',#40415,1.5);
#16802=CIRCLE('',#40416,1.5);
#16803=CIRCLE('',#40417,1.5);
#16804=CIRCLE('',#40418,1.5);
#16805=CIRCLE('',#40419,1.5);
#16806=CIRCLE('',#40420,1.5);
#16807=CIRCLE('',#40421,1.5);
#16808=CIRCLE('',#40422,1.5);
#16809=CIRCLE('',#40423,1.5);
#16810=CIRCLE('',#40424,1.5);
#16811=CIRCLE('',#40425,1.5);
#16812=CIRCLE('',#40426,1.5);
#16813=CIRCLE('',#40427,1.5);
#16814=CIRCLE('',#40428,1.5);
#16815=CIRCLE('',#40429,1.5);
#16816=CIRCLE('',#40430,1.5);
#16817=CIRCLE('',#40431,1.5);
#16818=CIRCLE('',#40432,1.5);
#16819=CIRCLE('',#40433,1.5);
#16820=CIRCLE('',#40434,1.5);
#16821=CIRCLE('',#40435,1.5);
#16822=CIRCLE('',#40436,1.5);
#16823=CIRCLE('',#40437,1.5);
#16824=CIRCLE('',#40438,1.5);
#16825=CIRCLE('',#40439,1.5);
#16826=CIRCLE('',#40442,1.5);
#16827=CIRCLE('',#40443,1.5);
#16828=CIRCLE('',#40444,2.667);
#16829=CIRCLE('',#40445,2.667);
#16830=CIRCLE('',#40446,2.66699999999999);
#16831=CIRCLE('',#40447,2.667);
#16832=CIRCLE('',#40448,2.667);
#16833=CIRCLE('',#40449,2.667);
#16834=CIRCLE('',#40451,1.5);
#16835=CIRCLE('',#40452,1.5);
#16836=CIRCLE('',#40453,2.667);
#16837=CIRCLE('',#40454,2.667);
#16838=CIRCLE('',#40455,2.667);
#16839=CIRCLE('',#40456,2.667);
#16840=CIRCLE('',#40457,2.66699999999999);
#16841=CIRCLE('',#40458,2.667);
#16842=CIRCLE('',#40486,2.);
#16843=CIRCLE('',#40487,2.);
#16844=CIRCLE('',#40489,2.);
#16845=CIRCLE('',#40490,2.);
#16846=CIRCLE('',#40492,2.);
#16847=CIRCLE('',#40493,2.);
#16848=CIRCLE('',#40495,2.);
#16849=CIRCLE('',#40496,2.);
#16850=CIRCLE('',#40498,1.2);
#16851=CIRCLE('',#40499,1.5);
#16852=CIRCLE('',#40500,1.5);
#16853=CIRCLE('',#40501,1.20000000000001);
#16854=CIRCLE('',#40502,2.3);
#16855=CIRCLE('',#40503,2.3);
#16856=CIRCLE('',#40505,1.20000000000001);
#16857=CIRCLE('',#40506,1.5);
#16858=CIRCLE('',#40507,1.5);
#16859=CIRCLE('',#40508,1.2);
#16860=CIRCLE('',#40509,2.3);
#16861=CIRCLE('',#40510,2.3);
#16862=CIRCLE('',#40524,2.);
#16863=CIRCLE('',#40525,2.);
#16864=CIRCLE('',#40527,2.);
#16865=CIRCLE('',#40528,2.);
#16866=CIRCLE('',#40530,2.);
#16867=CIRCLE('',#40531,2.);
#16868=CIRCLE('',#40533,2.);
#16869=CIRCLE('',#40534,2.);
#16870=CIRCLE('',#40536,1.2);
#16871=CIRCLE('',#40537,1.5);
#16872=CIRCLE('',#40538,1.5);
#16873=CIRCLE('',#40539,1.20000000000001);
#16874=CIRCLE('',#40540,2.3);
#16875=CIRCLE('',#40541,2.3);
#16876=CIRCLE('',#40543,1.20000000000001);
#16877=CIRCLE('',#40544,1.5);
#16878=CIRCLE('',#40545,1.5);
#16879=CIRCLE('',#40546,1.2);
#16880=CIRCLE('',#40547,2.3);
#16881=CIRCLE('',#40548,2.3);
#16882=CIRCLE('',#40562,2.);
#16883=CIRCLE('',#40563,2.);
#16884=CIRCLE('',#40565,2.);
#16885=CIRCLE('',#40566,2.);
#16886=CIRCLE('',#40568,2.);
#16887=CIRCLE('',#40569,2.);
#16888=CIRCLE('',#40571,2.);
#16889=CIRCLE('',#40572,2.);
#16890=CIRCLE('',#40574,1.2);
#16891=CIRCLE('',#40575,1.5);
#16892=CIRCLE('',#40576,1.5);
#16893=CIRCLE('',#40577,1.2);
#16894=CIRCLE('',#40578,2.3);
#16895=CIRCLE('',#40579,2.3);
#16896=CIRCLE('',#40581,1.2);
#16897=CIRCLE('',#40582,1.5);
#16898=CIRCLE('',#40583,1.5);
#16899=CIRCLE('',#40584,1.2);
#16900=CIRCLE('',#40585,2.3);
#16901=CIRCLE('',#40586,2.3);
#16902=CIRCLE('',#40600,2.);
#16903=CIRCLE('',#40601,2.);
#16904=CIRCLE('',#40603,2.);
#16905=CIRCLE('',#40604,2.);
#16906=CIRCLE('',#40606,2.);
#16907=CIRCLE('',#40607,2.);
#16908=CIRCLE('',#40609,2.);
#16909=CIRCLE('',#40610,2.);
#16910=CIRCLE('',#40612,1.2);
#16911=CIRCLE('',#40613,1.5);
#16912=CIRCLE('',#40614,1.5);
#16913=CIRCLE('',#40615,1.2);
#16914=CIRCLE('',#40616,2.3);
#16915=CIRCLE('',#40617,2.3);
#16916=CIRCLE('',#40619,1.2);
#16917=CIRCLE('',#40620,1.5);
#16918=CIRCLE('',#40621,1.5);
#16919=CIRCLE('',#40622,1.2);
#16920=CIRCLE('',#40623,2.3);
#16921=CIRCLE('',#40624,2.3);
#16922=CIRCLE('',#40638,1.5);
#16923=CIRCLE('',#40639,1.5);
#16924=CIRCLE('',#40640,1.5);
#16925=CIRCLE('',#40641,1.5);
#16926=CIRCLE('',#40642,1.5);
#16927=CIRCLE('',#40643,1.5);
#16928=CIRCLE('',#40644,1.5);
#16929=CIRCLE('',#40645,1.5);
#16930=CIRCLE('',#40646,1.5);
#16931=CIRCLE('',#40647,1.5);
#16932=CIRCLE('',#40648,1.5);
#16933=CIRCLE('',#40649,1.5);
#16934=CIRCLE('',#40650,1.5);
#16935=CIRCLE('',#40651,1.5);
#16936=CIRCLE('',#40652,1.5);
#16937=CIRCLE('',#40653,1.5);
#16938=CIRCLE('',#40654,1.5);
#16939=CIRCLE('',#40655,1.5);
#16940=CIRCLE('',#40656,1.5);
#16941=CIRCLE('',#40657,1.5);
#16942=CIRCLE('',#40658,1.5);
#16943=CIRCLE('',#40659,1.5);
#16944=CIRCLE('',#40660,1.5);
#16945=CIRCLE('',#40661,1.5);
#16946=CIRCLE('',#40662,1.5);
#16947=CIRCLE('',#40663,1.5);
#16948=CIRCLE('',#40664,1.5);
#16949=CIRCLE('',#40665,1.5);
#16950=CIRCLE('',#40666,1.5);
#16951=CIRCLE('',#40667,1.5);
#16952=CIRCLE('',#40668,1.5);
#16953=CIRCLE('',#40669,1.5);
#16954=CIRCLE('',#40670,1.5);
#16955=CIRCLE('',#40671,1.5);
#16956=CIRCLE('',#40672,1.5);
#16957=CIRCLE('',#40673,1.5);
#16958=CIRCLE('',#40674,1.5);
#16959=CIRCLE('',#40675,1.5);
#16960=CIRCLE('',#40676,1.5);
#16961=CIRCLE('',#40677,1.5);
#16962=CIRCLE('',#40678,1.5);
#16963=CIRCLE('',#40679,1.5);
#16964=CIRCLE('',#40680,1.5);
#16965=CIRCLE('',#40681,1.5);
#16966=CIRCLE('',#40682,1.5);
#16967=CIRCLE('',#40683,1.5);
#16968=CIRCLE('',#40684,1.5);
#16969=CIRCLE('',#40685,1.5);
#16970=CIRCLE('',#40686,1.5);
#16971=CIRCLE('',#40687,1.5);
#16972=CIRCLE('',#40688,1.5);
#16973=CIRCLE('',#40689,1.5);
#16974=CIRCLE('',#40690,1.5);
#16975=CIRCLE('',#40691,1.5);
#16976=CIRCLE('',#40928,0.799999999999995);
#16977=CIRCLE('',#40929,1.59999999999999);
#16978=CIRCLE('',#40931,0.799999999999995);
#16979=CIRCLE('',#40932,1.59999999999999);
#16980=CIRCLE('',#40941,2.);
#16981=CIRCLE('',#40942,2.);
#16982=CIRCLE('',#40944,2.);
#16983=CIRCLE('',#40945,2.);
#16984=CIRCLE('',#40947,2.);
#16985=CIRCLE('',#40948,2.);
#16986=CIRCLE('',#40950,2.);
#16987=CIRCLE('',#40951,2.);
#16988=CIRCLE('',#40953,1.20000000000001);
#16989=CIRCLE('',#40954,2.3);
#16990=CIRCLE('',#40955,2.3);
#16991=CIRCLE('',#40956,1.20000000000001);
#16992=CIRCLE('',#40957,1.5);
#16993=CIRCLE('',#40958,1.5);
#16994=CIRCLE('',#40960,1.20000000000001);
#16995=CIRCLE('',#40961,2.3);
#16996=CIRCLE('',#40962,2.3);
#16997=CIRCLE('',#40963,1.20000000000001);
#16998=CIRCLE('',#40964,1.5);
#16999=CIRCLE('',#40965,1.5);
#17000=CIRCLE('',#40979,2.);
#17001=CIRCLE('',#40980,2.);
#17002=CIRCLE('',#40982,2.);
#17003=CIRCLE('',#40983,2.);
#17004=CIRCLE('',#40985,2.);
#17005=CIRCLE('',#40986,2.);
#17006=CIRCLE('',#40988,2.);
#17007=CIRCLE('',#40989,2.);
#17008=CIRCLE('',#40991,1.2);
#17009=CIRCLE('',#40992,2.3);
#17010=CIRCLE('',#40993,2.3);
#17011=CIRCLE('',#40994,1.2);
#17012=CIRCLE('',#40995,1.5);
#17013=CIRCLE('',#40996,1.5);
#17014=CIRCLE('',#40998,1.2);
#17015=CIRCLE('',#40999,2.3);
#17016=CIRCLE('',#41000,2.3);
#17017=CIRCLE('',#41001,1.2);
#17018=CIRCLE('',#41002,1.5);
#17019=CIRCLE('',#41003,1.5);
#17020=CIRCLE('',#41023,0.799999999999995);
#17021=CIRCLE('',#41024,1.59999999999999);
#17022=CIRCLE('',#41026,0.799999999999995);
#17023=CIRCLE('',#41027,1.59999999999999);
#17024=CIRCLE('',#41033,4.);
#17025=CIRCLE('',#41034,4.);
#17026=CIRCLE('',#41036,4.);
#17027=CIRCLE('',#41037,4.);
#17144=VERTEX_POINT('',#52454);
#17145=VERTEX_POINT('',#52456);
#17146=VERTEX_POINT('',#52460);
#17147=VERTEX_POINT('',#52462);
#17148=VERTEX_POINT('',#52466);
#17149=VERTEX_POINT('',#52468);
#17150=VERTEX_POINT('',#52472);
#17151=VERTEX_POINT('',#52474);
#17152=VERTEX_POINT('',#52478);
#17153=VERTEX_POINT('',#52480);
#17154=VERTEX_POINT('',#52484);
#17155=VERTEX_POINT('',#52486);
#17156=VERTEX_POINT('',#52490);
#17157=VERTEX_POINT('',#52491);
#17158=VERTEX_POINT('',#52493);
#17159=VERTEX_POINT('',#52495);
#17160=VERTEX_POINT('',#52499);
#17161=VERTEX_POINT('',#52500);
#17162=VERTEX_POINT('',#52502);
#17163=VERTEX_POINT('',#52504);
#17164=VERTEX_POINT('',#52508);
#17165=VERTEX_POINT('',#52509);
#17166=VERTEX_POINT('',#52511);
#17167=VERTEX_POINT('',#52513);
#17168=VERTEX_POINT('',#52517);
#17169=VERTEX_POINT('',#52518);
#17170=VERTEX_POINT('',#52520);
#17171=VERTEX_POINT('',#52522);
#17172=VERTEX_POINT('',#52526);
#17173=VERTEX_POINT('',#52527);
#17174=VERTEX_POINT('',#52529);
#17175=VERTEX_POINT('',#52531);
#17176=VERTEX_POINT('',#52535);
#17177=VERTEX_POINT('',#52536);
#17178=VERTEX_POINT('',#52538);
#17179=VERTEX_POINT('',#52540);
#17180=VERTEX_POINT('',#52544);
#17181=VERTEX_POINT('',#52545);
#17182=VERTEX_POINT('',#52547);
#17183=VERTEX_POINT('',#52549);
#17184=VERTEX_POINT('',#52553);
#17185=VERTEX_POINT('',#52554);
#17186=VERTEX_POINT('',#52556);
#17187=VERTEX_POINT('',#52558);
#17188=VERTEX_POINT('',#52562);
#17189=VERTEX_POINT('',#52563);
#17190=VERTEX_POINT('',#52565);
#17191=VERTEX_POINT('',#52567);
#17192=VERTEX_POINT('',#52571);
#17193=VERTEX_POINT('',#52572);
#17194=VERTEX_POINT('',#52574);
#17195=VERTEX_POINT('',#52576);
#17196=VERTEX_POINT('',#52580);
#17197=VERTEX_POINT('',#52581);
#17198=VERTEX_POINT('',#52583);
#17199=VERTEX_POINT('',#52585);
#17200=VERTEX_POINT('',#52589);
#17201=VERTEX_POINT('',#52590);
#17202=VERTEX_POINT('',#52592);
#17203=VERTEX_POINT('',#52594);
#17204=VERTEX_POINT('',#52598);
#17205=VERTEX_POINT('',#52599);
#17206=VERTEX_POINT('',#52601);
#17207=VERTEX_POINT('',#52603);
#17208=VERTEX_POINT('',#52607);
#17209=VERTEX_POINT('',#52608);
#17210=VERTEX_POINT('',#52610);
#17211=VERTEX_POINT('',#52612);
#17212=VERTEX_POINT('',#52616);
#17213=VERTEX_POINT('',#52617);
#17214=VERTEX_POINT('',#52619);
#17215=VERTEX_POINT('',#52621);
#17216=VERTEX_POINT('',#52625);
#17217=VERTEX_POINT('',#52626);
#17218=VERTEX_POINT('',#52628);
#17219=VERTEX_POINT('',#52630);
#17220=VERTEX_POINT('',#52634);
#17221=VERTEX_POINT('',#52635);
#17222=VERTEX_POINT('',#52637);
#17223=VERTEX_POINT('',#52639);
#17224=VERTEX_POINT('',#52643);
#17225=VERTEX_POINT('',#52644);
#17226=VERTEX_POINT('',#52646);
#17227=VERTEX_POINT('',#52648);
#17228=VERTEX_POINT('',#52652);
#17229=VERTEX_POINT('',#52653);
#17230=VERTEX_POINT('',#52655);
#17231=VERTEX_POINT('',#52657);
#17232=VERTEX_POINT('',#52661);
#17233=VERTEX_POINT('',#52662);
#17234=VERTEX_POINT('',#52664);
#17235=VERTEX_POINT('',#52666);
#17236=VERTEX_POINT('',#52670);
#17237=VERTEX_POINT('',#52671);
#17238=VERTEX_POINT('',#52673);
#17239=VERTEX_POINT('',#52675);
#17240=VERTEX_POINT('',#52679);
#17241=VERTEX_POINT('',#52680);
#17242=VERTEX_POINT('',#52682);
#17243=VERTEX_POINT('',#52684);
#17244=VERTEX_POINT('',#52688);
#17245=VERTEX_POINT('',#52689);
#17246=VERTEX_POINT('',#52691);
#17247=VERTEX_POINT('',#52693);
#17248=VERTEX_POINT('',#52697);
#17249=VERTEX_POINT('',#52698);
#17250=VERTEX_POINT('',#52700);
#17251=VERTEX_POINT('',#52702);
#17252=VERTEX_POINT('',#52706);
#17253=VERTEX_POINT('',#52707);
#17254=VERTEX_POINT('',#52709);
#17255=VERTEX_POINT('',#52711);
#17256=VERTEX_POINT('',#52715);
#17257=VERTEX_POINT('',#52716);
#17258=VERTEX_POINT('',#52718);
#17259=VERTEX_POINT('',#52720);
#17260=VERTEX_POINT('',#52724);
#17261=VERTEX_POINT('',#52725);
#17262=VERTEX_POINT('',#52727);
#17263=VERTEX_POINT('',#52729);
#17264=VERTEX_POINT('',#52733);
#17265=VERTEX_POINT('',#52734);
#17266=VERTEX_POINT('',#52736);
#17267=VERTEX_POINT('',#52738);
#17268=VERTEX_POINT('',#52742);
#17269=VERTEX_POINT('',#52743);
#17270=VERTEX_POINT('',#52745);
#17271=VERTEX_POINT('',#52747);
#17272=VERTEX_POINT('',#52751);
#17273=VERTEX_POINT('',#52752);
#17274=VERTEX_POINT('',#52754);
#17275=VERTEX_POINT('',#52756);
#17276=VERTEX_POINT('',#52760);
#17277=VERTEX_POINT('',#52761);
#17278=VERTEX_POINT('',#52763);
#17279=VERTEX_POINT('',#52765);
#17280=VERTEX_POINT('',#52769);
#17281=VERTEX_POINT('',#52770);
#17282=VERTEX_POINT('',#52772);
#17283=VERTEX_POINT('',#52774);
#17284=VERTEX_POINT('',#52778);
#17285=VERTEX_POINT('',#52779);
#17286=VERTEX_POINT('',#52781);
#17287=VERTEX_POINT('',#52783);
#17288=VERTEX_POINT('',#52787);
#17289=VERTEX_POINT('',#52788);
#17290=VERTEX_POINT('',#52790);
#17291=VERTEX_POINT('',#52792);
#17292=VERTEX_POINT('',#52796);
#17293=VERTEX_POINT('',#52797);
#17294=VERTEX_POINT('',#52799);
#17295=VERTEX_POINT('',#52801);
#17296=VERTEX_POINT('',#52805);
#17297=VERTEX_POINT('',#52806);
#17298=VERTEX_POINT('',#52808);
#17299=VERTEX_POINT('',#52810);
#17300=VERTEX_POINT('',#52814);
#17301=VERTEX_POINT('',#52815);
#17302=VERTEX_POINT('',#52817);
#17303=VERTEX_POINT('',#52819);
#17304=VERTEX_POINT('',#52823);
#17305=VERTEX_POINT('',#52824);
#17306=VERTEX_POINT('',#52826);
#17307=VERTEX_POINT('',#52828);
#17308=VERTEX_POINT('',#52832);
#17309=VERTEX_POINT('',#52833);
#17310=VERTEX_POINT('',#52835);
#17311=VERTEX_POINT('',#52837);
#17312=VERTEX_POINT('',#52841);
#17313=VERTEX_POINT('',#52842);
#17314=VERTEX_POINT('',#52844);
#17315=VERTEX_POINT('',#52846);
#17316=VERTEX_POINT('',#52850);
#17317=VERTEX_POINT('',#52851);
#17318=VERTEX_POINT('',#52853);
#17319=VERTEX_POINT('',#52855);
#17320=VERTEX_POINT('',#52859);
#17321=VERTEX_POINT('',#52860);
#17322=VERTEX_POINT('',#52862);
#17323=VERTEX_POINT('',#52864);
#17324=VERTEX_POINT('',#52868);
#17325=VERTEX_POINT('',#52869);
#17326=VERTEX_POINT('',#52871);
#17327=VERTEX_POINT('',#52873);
#17328=VERTEX_POINT('',#52877);
#17329=VERTEX_POINT('',#52878);
#17330=VERTEX_POINT('',#52880);
#17331=VERTEX_POINT('',#52882);
#17332=VERTEX_POINT('',#52886);
#17333=VERTEX_POINT('',#52887);
#17334=VERTEX_POINT('',#52889);
#17335=VERTEX_POINT('',#52891);
#17336=VERTEX_POINT('',#52895);
#17337=VERTEX_POINT('',#52896);
#17338=VERTEX_POINT('',#52898);
#17339=VERTEX_POINT('',#52900);
#17340=VERTEX_POINT('',#52904);
#17341=VERTEX_POINT('',#52905);
#17342=VERTEX_POINT('',#52907);
#17343=VERTEX_POINT('',#52909);
#17344=VERTEX_POINT('',#52913);
#17345=VERTEX_POINT('',#52914);
#17346=VERTEX_POINT('',#52916);
#17347=VERTEX_POINT('',#52918);
#17348=VERTEX_POINT('',#52922);
#17349=VERTEX_POINT('',#52923);
#17350=VERTEX_POINT('',#52925);
#17351=VERTEX_POINT('',#52927);
#17352=VERTEX_POINT('',#52931);
#17353=VERTEX_POINT('',#52932);
#17354=VERTEX_POINT('',#52934);
#17355=VERTEX_POINT('',#52936);
#17356=VERTEX_POINT('',#52940);
#17357=VERTEX_POINT('',#52941);
#17358=VERTEX_POINT('',#52943);
#17359=VERTEX_POINT('',#52945);
#17360=VERTEX_POINT('',#52949);
#17361=VERTEX_POINT('',#52950);
#17362=VERTEX_POINT('',#52952);
#17363=VERTEX_POINT('',#52954);
#17364=VERTEX_POINT('',#52958);
#17365=VERTEX_POINT('',#52959);
#17366=VERTEX_POINT('',#52961);
#17367=VERTEX_POINT('',#52963);
#17368=VERTEX_POINT('',#52967);
#17369=VERTEX_POINT('',#52968);
#17370=VERTEX_POINT('',#52970);
#17371=VERTEX_POINT('',#52972);
#17372=VERTEX_POINT('',#52976);
#17373=VERTEX_POINT('',#52977);
#17374=VERTEX_POINT('',#52979);
#17375=VERTEX_POINT('',#52981);
#17376=VERTEX_POINT('',#52985);
#17377=VERTEX_POINT('',#52986);
#17378=VERTEX_POINT('',#52988);
#17379=VERTEX_POINT('',#52990);
#17380=VERTEX_POINT('',#52994);
#17381=VERTEX_POINT('',#52995);
#17382=VERTEX_POINT('',#52997);
#17383=VERTEX_POINT('',#52999);
#17384=VERTEX_POINT('',#53003);
#17385=VERTEX_POINT('',#53004);
#17386=VERTEX_POINT('',#53006);
#17387=VERTEX_POINT('',#53008);
#17388=VERTEX_POINT('',#53012);
#17389=VERTEX_POINT('',#53013);
#17390=VERTEX_POINT('',#53015);
#17391=VERTEX_POINT('',#53017);
#17392=VERTEX_POINT('',#53021);
#17393=VERTEX_POINT('',#53022);
#17394=VERTEX_POINT('',#53024);
#17395=VERTEX_POINT('',#53026);
#17396=VERTEX_POINT('',#53030);
#17397=VERTEX_POINT('',#53031);
#17398=VERTEX_POINT('',#53033);
#17399=VERTEX_POINT('',#53035);
#17400=VERTEX_POINT('',#53039);
#17401=VERTEX_POINT('',#53040);
#17402=VERTEX_POINT('',#53042);
#17403=VERTEX_POINT('',#53044);
#17404=VERTEX_POINT('',#53048);
#17405=VERTEX_POINT('',#53049);
#17406=VERTEX_POINT('',#53051);
#17407=VERTEX_POINT('',#53053);
#17408=VERTEX_POINT('',#53057);
#17409=VERTEX_POINT('',#53058);
#17410=VERTEX_POINT('',#53060);
#17411=VERTEX_POINT('',#53062);
#17412=VERTEX_POINT('',#53066);
#17413=VERTEX_POINT('',#53067);
#17414=VERTEX_POINT('',#53069);
#17415=VERTEX_POINT('',#53071);
#17416=VERTEX_POINT('',#53075);
#17417=VERTEX_POINT('',#53076);
#17418=VERTEX_POINT('',#53078);
#17419=VERTEX_POINT('',#53080);
#17420=VERTEX_POINT('',#53093);
#17421=VERTEX_POINT('',#53094);
#17422=VERTEX_POINT('',#53102);
#17423=VERTEX_POINT('',#53104);
#17424=VERTEX_POINT('',#53123);
#17425=VERTEX_POINT('',#53124);
#17426=VERTEX_POINT('',#53130);
#17427=VERTEX_POINT('',#53132);
#17428=VERTEX_POINT('',#53149);
#17429=VERTEX_POINT('',#53150);
#17430=VERTEX_POINT('',#53156);
#17431=VERTEX_POINT('',#53158);
#17432=VERTEX_POINT('',#53177);
#17433=VERTEX_POINT('',#53178);
#17434=VERTEX_POINT('',#53185);
#17435=VERTEX_POINT('',#53187);
#17436=VERTEX_POINT('',#53207);
#17437=VERTEX_POINT('',#53208);
#17438=VERTEX_POINT('',#53215);
#17439=VERTEX_POINT('',#53217);
#17440=VERTEX_POINT('',#53226);
#17441=VERTEX_POINT('',#53228);
#17442=VERTEX_POINT('',#53232);
#17443=VERTEX_POINT('',#53234);
#17444=VERTEX_POINT('',#53238);
#17445=VERTEX_POINT('',#53240);
#17446=VERTEX_POINT('',#53244);
#17447=VERTEX_POINT('',#53246);
#17448=VERTEX_POINT('',#53250);
#17449=VERTEX_POINT('',#53252);
#17450=VERTEX_POINT('',#53256);
#17451=VERTEX_POINT('',#53258);
#17452=VERTEX_POINT('',#53262);
#17453=VERTEX_POINT('',#53266);
#17454=VERTEX_POINT('',#53270);
#17455=VERTEX_POINT('',#53272);
#17456=VERTEX_POINT('',#53276);
#17457=VERTEX_POINT('',#53278);
#17458=VERTEX_POINT('',#53282);
#17459=VERTEX_POINT('',#53284);
#17460=VERTEX_POINT('',#53288);
#17461=VERTEX_POINT('',#53290);
#17462=VERTEX_POINT('',#53309);
#17463=VERTEX_POINT('',#53310);
#17464=VERTEX_POINT('',#53319);
#17465=VERTEX_POINT('',#53321);
#17466=VERTEX_POINT('',#53332);
#17467=VERTEX_POINT('',#53333);
#17468=VERTEX_POINT('',#53335);
#17469=VERTEX_POINT('',#53337);
#17470=VERTEX_POINT('',#53339);
#17471=VERTEX_POINT('',#53341);
#17472=VERTEX_POINT('',#53343);
#17473=VERTEX_POINT('',#53345);
#17474=VERTEX_POINT('',#53347);
#17475=VERTEX_POINT('',#53349);
#17476=VERTEX_POINT('',#53351);
#17477=VERTEX_POINT('',#53353);
#17478=VERTEX_POINT('',#53355);
#17479=VERTEX_POINT('',#53357);
#17480=VERTEX_POINT('',#53359);
#17481=VERTEX_POINT('',#53361);
#17482=VERTEX_POINT('',#53363);
#17483=VERTEX_POINT('',#53365);
#17484=VERTEX_POINT('',#53367);
#17485=VERTEX_POINT('',#53369);
#17486=VERTEX_POINT('',#53371);
#17487=VERTEX_POINT('',#53373);
#17488=VERTEX_POINT('',#53375);
#17489=VERTEX_POINT('',#53377);
#17490=VERTEX_POINT('',#53379);
#17491=VERTEX_POINT('',#53381);
#17492=VERTEX_POINT('',#53383);
#17493=VERTEX_POINT('',#53385);
#17494=VERTEX_POINT('',#53388);
#17495=VERTEX_POINT('',#53389);
#17496=VERTEX_POINT('',#53391);
#17497=VERTEX_POINT('',#53393);
#17498=VERTEX_POINT('',#53395);
#17499=VERTEX_POINT('',#53397);
#17500=VERTEX_POINT('',#53399);
#17501=VERTEX_POINT('',#53401);
#17502=VERTEX_POINT('',#53404);
#17503=VERTEX_POINT('',#53405);
#17504=VERTEX_POINT('',#53407);
#17505=VERTEX_POINT('',#53409);
#17506=VERTEX_POINT('',#53411);
#17507=VERTEX_POINT('',#53413);
#17508=VERTEX_POINT('',#53415);
#17509=VERTEX_POINT('',#53417);
#17510=VERTEX_POINT('',#53420);
#17511=VERTEX_POINT('',#53421);
#17512=VERTEX_POINT('',#53423);
#17513=VERTEX_POINT('',#53425);
#17514=VERTEX_POINT('',#53427);
#17515=VERTEX_POINT('',#53429);
#17516=VERTEX_POINT('',#53431);
#17517=VERTEX_POINT('',#53433);
#17518=VERTEX_POINT('',#53436);
#17519=VERTEX_POINT('',#53437);
#17520=VERTEX_POINT('',#53439);
#17521=VERTEX_POINT('',#53441);
#17522=VERTEX_POINT('',#53443);
#17523=VERTEX_POINT('',#53445);
#17524=VERTEX_POINT('',#53447);
#17525=VERTEX_POINT('',#53449);
#17526=VERTEX_POINT('',#53453);
#17527=VERTEX_POINT('',#53454);
#17528=VERTEX_POINT('',#53456);
#17529=VERTEX_POINT('',#53458);
#17530=VERTEX_POINT('',#53460);
#17531=VERTEX_POINT('',#53462);
#17532=VERTEX_POINT('',#53464);
#17533=VERTEX_POINT('',#53466);
#17534=VERTEX_POINT('',#53468);
#17535=VERTEX_POINT('',#53470);
#17536=VERTEX_POINT('',#53472);
#17537=VERTEX_POINT('',#53474);
#17538=VERTEX_POINT('',#53476);
#17539=VERTEX_POINT('',#53478);
#17540=VERTEX_POINT('',#53480);
#17541=VERTEX_POINT('',#53482);
#17542=VERTEX_POINT('',#53484);
#17543=VERTEX_POINT('',#53486);
#17544=VERTEX_POINT('',#53488);
#17545=VERTEX_POINT('',#53490);
#17546=VERTEX_POINT('',#53492);
#17547=VERTEX_POINT('',#53494);
#17548=VERTEX_POINT('',#53496);
#17549=VERTEX_POINT('',#53498);
#17550=VERTEX_POINT('',#53500);
#17551=VERTEX_POINT('',#53502);
#17552=VERTEX_POINT('',#53504);
#17553=VERTEX_POINT('',#53506);
#17554=VERTEX_POINT('',#53509);
#17555=VERTEX_POINT('',#53510);
#17556=VERTEX_POINT('',#53512);
#17557=VERTEX_POINT('',#53514);
#17558=VERTEX_POINT('',#53517);
#17559=VERTEX_POINT('',#53518);
#17560=VERTEX_POINT('',#53520);
#17561=VERTEX_POINT('',#53522);
#17562=VERTEX_POINT('',#53525);
#17563=VERTEX_POINT('',#53526);
#17564=VERTEX_POINT('',#53528);
#17565=VERTEX_POINT('',#53530);
#17566=VERTEX_POINT('',#53533);
#17567=VERTEX_POINT('',#53534);
#17568=VERTEX_POINT('',#53536);
#17569=VERTEX_POINT('',#53538);
#17570=VERTEX_POINT('',#53548);
#17571=VERTEX_POINT('',#53549);
#17572=VERTEX_POINT('',#53551);
#17573=VERTEX_POINT('',#53553);
#17574=VERTEX_POINT('',#53555);
#17575=VERTEX_POINT('',#53557);
#17576=VERTEX_POINT('',#53560);
#17577=VERTEX_POINT('',#53561);
#17578=VERTEX_POINT('',#53563);
#17579=VERTEX_POINT('',#53565);
#17580=VERTEX_POINT('',#53567);
#17581=VERTEX_POINT('',#53569);
#17582=VERTEX_POINT('',#53571);
#17583=VERTEX_POINT('',#53573);
#17584=VERTEX_POINT('',#53576);
#17585=VERTEX_POINT('',#53577);
#17586=VERTEX_POINT('',#53579);
#17587=VERTEX_POINT('',#53581);
#17588=VERTEX_POINT('',#53583);
#17589=VERTEX_POINT('',#53585);
#17590=VERTEX_POINT('',#53587);
#17591=VERTEX_POINT('',#53589);
#17592=VERTEX_POINT('',#53593);
#17593=VERTEX_POINT('',#53594);
#17594=VERTEX_POINT('',#53596);
#17595=VERTEX_POINT('',#53598);
#17596=VERTEX_POINT('',#53600);
#17597=VERTEX_POINT('',#53602);
#17598=VERTEX_POINT('',#53605);
#17599=VERTEX_POINT('',#53606);
#17600=VERTEX_POINT('',#53608);
#17601=VERTEX_POINT('',#53610);
#17602=VERTEX_POINT('',#53613);
#17603=VERTEX_POINT('',#53614);
#17604=VERTEX_POINT('',#53616);
#17605=VERTEX_POINT('',#53618);
#17606=VERTEX_POINT('',#53628);
#17607=VERTEX_POINT('',#53629);
#17608=VERTEX_POINT('',#53631);
#17609=VERTEX_POINT('',#53633);
#17610=VERTEX_POINT('',#53635);
#17611=VERTEX_POINT('',#53637);
#17612=VERTEX_POINT('',#53639);
#17613=VERTEX_POINT('',#53641);
#17614=VERTEX_POINT('',#53643);
#17615=VERTEX_POINT('',#53645);
#17616=VERTEX_POINT('',#53648);
#17617=VERTEX_POINT('',#53650);
#17618=VERTEX_POINT('',#53653);
#17619=VERTEX_POINT('',#53655);
#17620=VERTEX_POINT('',#53658);
#17621=VERTEX_POINT('',#53660);
#17622=VERTEX_POINT('',#53663);
#17623=VERTEX_POINT('',#53665);
#17624=VERTEX_POINT('',#53668);
#17625=VERTEX_POINT('',#53670);
#17626=VERTEX_POINT('',#53673);
#17627=VERTEX_POINT('',#53675);
#17628=VERTEX_POINT('',#53678);
#17629=VERTEX_POINT('',#53680);
#17630=VERTEX_POINT('',#53683);
#17631=VERTEX_POINT('',#53685);
#17632=VERTEX_POINT('',#53688);
#17633=VERTEX_POINT('',#53690);
#17634=VERTEX_POINT('',#53693);
#17635=VERTEX_POINT('',#53695);
#17636=VERTEX_POINT('',#53698);
#17637=VERTEX_POINT('',#53700);
#17638=VERTEX_POINT('',#53703);
#17639=VERTEX_POINT('',#53705);
#17640=VERTEX_POINT('',#53708);
#17641=VERTEX_POINT('',#53710);
#17642=VERTEX_POINT('',#53713);
#17643=VERTEX_POINT('',#53715);
#17644=VERTEX_POINT('',#53718);
#17645=VERTEX_POINT('',#53720);
#17646=VERTEX_POINT('',#53723);
#17647=VERTEX_POINT('',#53725);
#17648=VERTEX_POINT('',#53728);
#17649=VERTEX_POINT('',#53730);
#17650=VERTEX_POINT('',#53733);
#17651=VERTEX_POINT('',#53735);
#17652=VERTEX_POINT('',#53738);
#17653=VERTEX_POINT('',#53740);
#17654=VERTEX_POINT('',#53743);
#17655=VERTEX_POINT('',#53745);
#17656=VERTEX_POINT('',#53748);
#17657=VERTEX_POINT('',#53750);
#17658=VERTEX_POINT('',#53753);
#17659=VERTEX_POINT('',#53755);
#17660=VERTEX_POINT('',#53758);
#17661=VERTEX_POINT('',#53760);
#17662=VERTEX_POINT('',#53763);
#17663=VERTEX_POINT('',#53765);
#17664=VERTEX_POINT('',#53768);
#17665=VERTEX_POINT('',#53770);
#17666=VERTEX_POINT('',#53773);
#17667=VERTEX_POINT('',#53775);
#17668=VERTEX_POINT('',#53778);
#17669=VERTEX_POINT('',#53780);
#17670=VERTEX_POINT('',#53783);
#17671=VERTEX_POINT('',#53785);
#17672=VERTEX_POINT('',#53788);
#17673=VERTEX_POINT('',#53790);
#17674=VERTEX_POINT('',#53793);
#17675=VERTEX_POINT('',#53795);
#17676=VERTEX_POINT('',#53798);
#17677=VERTEX_POINT('',#53800);
#17678=VERTEX_POINT('',#53803);
#17679=VERTEX_POINT('',#53805);
#17680=VERTEX_POINT('',#53808);
#17681=VERTEX_POINT('',#53810);
#17682=VERTEX_POINT('',#53813);
#17683=VERTEX_POINT('',#53815);
#17684=VERTEX_POINT('',#53818);
#17685=VERTEX_POINT('',#53820);
#17686=VERTEX_POINT('',#53823);
#17687=VERTEX_POINT('',#53825);
#17688=VERTEX_POINT('',#53828);
#17689=VERTEX_POINT('',#53830);
#17690=VERTEX_POINT('',#53833);
#17691=VERTEX_POINT('',#53835);
#17692=VERTEX_POINT('',#53838);
#17693=VERTEX_POINT('',#53840);
#17694=VERTEX_POINT('',#53843);
#17695=VERTEX_POINT('',#53845);
#17696=VERTEX_POINT('',#53848);
#17697=VERTEX_POINT('',#53850);
#17698=VERTEX_POINT('',#53853);
#17699=VERTEX_POINT('',#53855);
#17700=VERTEX_POINT('',#53858);
#17701=VERTEX_POINT('',#53860);
#17702=VERTEX_POINT('',#53863);
#17703=VERTEX_POINT('',#53865);
#17704=VERTEX_POINT('',#53868);
#17705=VERTEX_POINT('',#53870);
#17706=VERTEX_POINT('',#53873);
#17707=VERTEX_POINT('',#53875);
#17708=VERTEX_POINT('',#53878);
#17709=VERTEX_POINT('',#53880);
#17710=VERTEX_POINT('',#53883);
#17711=VERTEX_POINT('',#53885);
#17712=VERTEX_POINT('',#53889);
#17713=VERTEX_POINT('',#53890);
#17714=VERTEX_POINT('',#53892);
#17715=VERTEX_POINT('',#53894);
#17716=VERTEX_POINT('',#53896);
#17717=VERTEX_POINT('',#53898);
#17718=VERTEX_POINT('',#53900);
#17719=VERTEX_POINT('',#53902);
#17720=VERTEX_POINT('',#53904);
#17721=VERTEX_POINT('',#53906);
#17722=VERTEX_POINT('',#53909);
#17723=VERTEX_POINT('',#53911);
#17724=VERTEX_POINT('',#53914);
#17725=VERTEX_POINT('',#53916);
#17726=VERTEX_POINT('',#53919);
#17727=VERTEX_POINT('',#53921);
#17728=VERTEX_POINT('',#53924);
#17729=VERTEX_POINT('',#53926);
#17730=VERTEX_POINT('',#53929);
#17731=VERTEX_POINT('',#53931);
#17732=VERTEX_POINT('',#53934);
#17733=VERTEX_POINT('',#53936);
#17734=VERTEX_POINT('',#53939);
#17735=VERTEX_POINT('',#53941);
#17736=VERTEX_POINT('',#53944);
#17737=VERTEX_POINT('',#53946);
#17738=VERTEX_POINT('',#53949);
#17739=VERTEX_POINT('',#53951);
#17740=VERTEX_POINT('',#53954);
#17741=VERTEX_POINT('',#53956);
#17742=VERTEX_POINT('',#53959);
#17743=VERTEX_POINT('',#53961);
#17744=VERTEX_POINT('',#53964);
#17745=VERTEX_POINT('',#53966);
#17746=VERTEX_POINT('',#53969);
#17747=VERTEX_POINT('',#53971);
#17748=VERTEX_POINT('',#53974);
#17749=VERTEX_POINT('',#53976);
#17750=VERTEX_POINT('',#53979);
#17751=VERTEX_POINT('',#53981);
#17752=VERTEX_POINT('',#53984);
#17753=VERTEX_POINT('',#53986);
#17754=VERTEX_POINT('',#53989);
#17755=VERTEX_POINT('',#53991);
#17756=VERTEX_POINT('',#53994);
#17757=VERTEX_POINT('',#53996);
#17758=VERTEX_POINT('',#53999);
#17759=VERTEX_POINT('',#54001);
#17760=VERTEX_POINT('',#54004);
#17761=VERTEX_POINT('',#54006);
#17762=VERTEX_POINT('',#54009);
#17763=VERTEX_POINT('',#54011);
#17764=VERTEX_POINT('',#54014);
#17765=VERTEX_POINT('',#54016);
#17766=VERTEX_POINT('',#54019);
#17767=VERTEX_POINT('',#54021);
#17768=VERTEX_POINT('',#54024);
#17769=VERTEX_POINT('',#54026);
#17770=VERTEX_POINT('',#54029);
#17771=VERTEX_POINT('',#54031);
#17772=VERTEX_POINT('',#54034);
#17773=VERTEX_POINT('',#54036);
#17774=VERTEX_POINT('',#54039);
#17775=VERTEX_POINT('',#54041);
#17776=VERTEX_POINT('',#54044);
#17777=VERTEX_POINT('',#54046);
#17778=VERTEX_POINT('',#54049);
#17779=VERTEX_POINT('',#54051);
#17780=VERTEX_POINT('',#54054);
#17781=VERTEX_POINT('',#54056);
#17782=VERTEX_POINT('',#54059);
#17783=VERTEX_POINT('',#54061);
#17784=VERTEX_POINT('',#54064);
#17785=VERTEX_POINT('',#54066);
#17786=VERTEX_POINT('',#54069);
#17787=VERTEX_POINT('',#54071);
#17788=VERTEX_POINT('',#54074);
#17789=VERTEX_POINT('',#54076);
#17790=VERTEX_POINT('',#54079);
#17791=VERTEX_POINT('',#54081);
#17792=VERTEX_POINT('',#54084);
#17793=VERTEX_POINT('',#54086);
#17794=VERTEX_POINT('',#54089);
#17795=VERTEX_POINT('',#54091);
#17796=VERTEX_POINT('',#54094);
#17797=VERTEX_POINT('',#54096);
#17798=VERTEX_POINT('',#54099);
#17799=VERTEX_POINT('',#54101);
#17800=VERTEX_POINT('',#54104);
#17801=VERTEX_POINT('',#54106);
#17802=VERTEX_POINT('',#54109);
#17803=VERTEX_POINT('',#54111);
#17804=VERTEX_POINT('',#54114);
#17805=VERTEX_POINT('',#54116);
#17806=VERTEX_POINT('',#54119);
#17807=VERTEX_POINT('',#54121);
#17808=VERTEX_POINT('',#54124);
#17809=VERTEX_POINT('',#54126);
#17810=VERTEX_POINT('',#54129);
#17811=VERTEX_POINT('',#54131);
#17812=VERTEX_POINT('',#54134);
#17813=VERTEX_POINT('',#54136);
#17814=VERTEX_POINT('',#54139);
#17815=VERTEX_POINT('',#54141);
#17816=VERTEX_POINT('',#54144);
#17817=VERTEX_POINT('',#54146);
#17818=VERTEX_POINT('',#54150);
#17819=VERTEX_POINT('',#54152);
#17820=VERTEX_POINT('',#54156);
#17821=VERTEX_POINT('',#54158);
#17822=VERTEX_POINT('',#54162);
#17823=VERTEX_POINT('',#54163);
#17824=VERTEX_POINT('',#54165);
#17825=VERTEX_POINT('',#54167);
#17826=VERTEX_POINT('',#54171);
#17827=VERTEX_POINT('',#54173);
#17828=VERTEX_POINT('',#54177);
#17829=VERTEX_POINT('',#54178);
#17830=VERTEX_POINT('',#54180);
#17831=VERTEX_POINT('',#54182);
#17832=VERTEX_POINT('',#54186);
#17833=VERTEX_POINT('',#54188);
#17834=VERTEX_POINT('',#54192);
#17835=VERTEX_POINT('',#54194);
#17836=VERTEX_POINT('',#54198);
#17837=VERTEX_POINT('',#54199);
#17838=VERTEX_POINT('',#54201);
#17839=VERTEX_POINT('',#54203);
#17840=VERTEX_POINT('',#54207);
#17841=VERTEX_POINT('',#54208);
#17842=VERTEX_POINT('',#54210);
#17843=VERTEX_POINT('',#54212);
#17844=VERTEX_POINT('',#54216);
#17845=VERTEX_POINT('',#54218);
#17846=VERTEX_POINT('',#54222);
#17847=VERTEX_POINT('',#54223);
#17848=VERTEX_POINT('',#54225);
#17849=VERTEX_POINT('',#54227);
#17850=VERTEX_POINT('',#54231);
#17851=VERTEX_POINT('',#54232);
#17852=VERTEX_POINT('',#54234);
#17853=VERTEX_POINT('',#54236);
#17854=VERTEX_POINT('',#54240);
#17855=VERTEX_POINT('',#54242);
#17856=VERTEX_POINT('',#54246);
#17857=VERTEX_POINT('',#54248);
#17858=VERTEX_POINT('',#54252);
#17859=VERTEX_POINT('',#54253);
#17860=VERTEX_POINT('',#54255);
#17861=VERTEX_POINT('',#54257);
#17862=VERTEX_POINT('',#54261);
#17863=VERTEX_POINT('',#54263);
#17864=VERTEX_POINT('',#54267);
#17865=VERTEX_POINT('',#54268);
#17866=VERTEX_POINT('',#54270);
#17867=VERTEX_POINT('',#54272);
#17868=VERTEX_POINT('',#54276);
#17869=VERTEX_POINT('',#54278);
#17870=VERTEX_POINT('',#54282);
#17871=VERTEX_POINT('',#54284);
#17872=VERTEX_POINT('',#54288);
#17873=VERTEX_POINT('',#54289);
#17874=VERTEX_POINT('',#54291);
#17875=VERTEX_POINT('',#54293);
#17876=VERTEX_POINT('',#54297);
#17877=VERTEX_POINT('',#54298);
#17878=VERTEX_POINT('',#54300);
#17879=VERTEX_POINT('',#54302);
#17880=VERTEX_POINT('',#54306);
#17881=VERTEX_POINT('',#54308);
#17882=VERTEX_POINT('',#54312);
#17883=VERTEX_POINT('',#54313);
#17884=VERTEX_POINT('',#54315);
#17885=VERTEX_POINT('',#54317);
#17886=VERTEX_POINT('',#54321);
#17887=VERTEX_POINT('',#54322);
#17888=VERTEX_POINT('',#54324);
#17889=VERTEX_POINT('',#54326);
#17890=VERTEX_POINT('',#54355);
#17891=VERTEX_POINT('',#54356);
#17892=VERTEX_POINT('',#54370);
#17893=VERTEX_POINT('',#54372);
#17894=VERTEX_POINT('',#54389);
#17895=VERTEX_POINT('',#54403);
#17896=VERTEX_POINT('',#54405);
#17897=VERTEX_POINT('',#54407);
#17898=VERTEX_POINT('',#54416);
#17899=VERTEX_POINT('',#54424);
#17900=VERTEX_POINT('',#54425);
#17901=VERTEX_POINT('',#54427);
#17902=VERTEX_POINT('',#54435);
#17903=VERTEX_POINT('',#54437);
#17904=VERTEX_POINT('',#54439);
#17905=VERTEX_POINT('',#54449);
#17906=VERTEX_POINT('',#54451);
#17907=VERTEX_POINT('',#54458);
#17908=VERTEX_POINT('',#54460);
#17909=VERTEX_POINT('',#54462);
#17910=VERTEX_POINT('',#54464);
#17911=VERTEX_POINT('',#54474);
#17912=VERTEX_POINT('',#54476);
#17913=VERTEX_POINT('',#54478);
#17914=VERTEX_POINT('',#54486);
#17915=VERTEX_POINT('',#54488);
#17916=VERTEX_POINT('',#54490);
#17917=VERTEX_POINT('',#54499);
#17918=VERTEX_POINT('',#54501);
#17919=VERTEX_POINT('',#54503);
#17920=VERTEX_POINT('',#54510);
#17921=VERTEX_POINT('',#54512);
#17922=VERTEX_POINT('',#54514);
#17923=VERTEX_POINT('',#54524);
#17924=VERTEX_POINT('',#54525);
#17925=VERTEX_POINT('',#54527);
#17926=VERTEX_POINT('',#54529);
#17927=VERTEX_POINT('',#54536);
#17928=VERTEX_POINT('',#54539);
#17929=VERTEX_POINT('',#54549);
#17930=VERTEX_POINT('',#54559);
#17931=VERTEX_POINT('',#54561);
#17932=VERTEX_POINT('',#54571);
#17933=VERTEX_POINT('',#54581);
#17934=VERTEX_POINT('',#54583);
#17935=VERTEX_POINT('',#54593);
#17936=VERTEX_POINT('',#54595);
#17937=VERTEX_POINT('',#54604);
#17938=VERTEX_POINT('',#54615);
#17939=VERTEX_POINT('',#54617);
#17940=VERTEX_POINT('',#54627);
#17941=VERTEX_POINT('',#54637);
#17942=VERTEX_POINT('',#54639);
#17943=VERTEX_POINT('',#54649);
#17944=VERTEX_POINT('',#54659);
#17945=VERTEX_POINT('',#54671);
#17946=VERTEX_POINT('',#54681);
#17947=VERTEX_POINT('',#54683);
#17948=VERTEX_POINT('',#54698);
#17949=VERTEX_POINT('',#54700);
#17950=VERTEX_POINT('',#54711);
#17951=VERTEX_POINT('',#54726);
#17952=VERTEX_POINT('',#54728);
#17953=VERTEX_POINT('',#54738);
#17954=VERTEX_POINT('',#54753);
#17955=VERTEX_POINT('',#54755);
#17956=VERTEX_POINT('',#54765);
#17957=VERTEX_POINT('',#54781);
#17958=VERTEX_POINT('',#54823);
#17959=VERTEX_POINT('',#54852);
#17960=VERTEX_POINT('',#54893);
#17961=VERTEX_POINT('',#54934);
#17962=VERTEX_POINT('',#54950);
#17963=VERTEX_POINT('',#54951);
#17964=VERTEX_POINT('',#54953);
#17965=VERTEX_POINT('',#54955);
#17966=VERTEX_POINT('',#54957);
#17967=VERTEX_POINT('',#54959);
#17968=VERTEX_POINT('',#54961);
#17969=VERTEX_POINT('',#54963);
#17970=VERTEX_POINT('',#54965);
#17971=VERTEX_POINT('',#54967);
#17972=VERTEX_POINT('',#54970);
#17973=VERTEX_POINT('',#54971);
#17974=VERTEX_POINT('',#54973);
#17975=VERTEX_POINT('',#54975);
#17976=VERTEX_POINT('',#54978);
#17977=VERTEX_POINT('',#54979);
#17978=VERTEX_POINT('',#54981);
#17979=VERTEX_POINT('',#54983);
#17980=VERTEX_POINT('',#54985);
#17981=VERTEX_POINT('',#54987);
#17982=VERTEX_POINT('',#54989);
#17983=VERTEX_POINT('',#54991);
#17984=VERTEX_POINT('',#54993);
#17985=VERTEX_POINT('',#54995);
#17986=VERTEX_POINT('',#54997);
#17987=VERTEX_POINT('',#54999);
#17988=VERTEX_POINT('',#55003);
#17989=VERTEX_POINT('',#55004);
#17990=VERTEX_POINT('',#55006);
#17991=VERTEX_POINT('',#55008);
#17992=VERTEX_POINT('',#55010);
#17993=VERTEX_POINT('',#55012);
#17994=VERTEX_POINT('',#55014);
#17995=VERTEX_POINT('',#55016);
#17996=VERTEX_POINT('',#55018);
#17997=VERTEX_POINT('',#55020);
#17998=VERTEX_POINT('',#55023);
#17999=VERTEX_POINT('',#55024);
#18000=VERTEX_POINT('',#55026);
#18001=VERTEX_POINT('',#55028);
#18002=VERTEX_POINT('',#55031);
#18003=VERTEX_POINT('',#55032);
#18004=VERTEX_POINT('',#55034);
#18005=VERTEX_POINT('',#55036);
#18006=VERTEX_POINT('',#55038);
#18007=VERTEX_POINT('',#55040);
#18008=VERTEX_POINT('',#55042);
#18009=VERTEX_POINT('',#55044);
#18010=VERTEX_POINT('',#55046);
#18011=VERTEX_POINT('',#55048);
#18012=VERTEX_POINT('',#55050);
#18013=VERTEX_POINT('',#55052);
#18014=VERTEX_POINT('',#55056);
#18015=VERTEX_POINT('',#55062);
#18016=VERTEX_POINT('',#55068);
#18017=VERTEX_POINT('',#55074);
#18018=VERTEX_POINT('',#55139);
#18019=VERTEX_POINT('',#55225);
#18020=VERTEX_POINT('',#55348);
#18021=VERTEX_POINT('',#55474);
#18022=VERTEX_POINT('',#55544);
#18023=VERTEX_POINT('',#55546);
#18024=VERTEX_POINT('',#55550);
#18025=VERTEX_POINT('',#55552);
#18026=VERTEX_POINT('',#55556);
#18027=VERTEX_POINT('',#55558);
#18028=VERTEX_POINT('',#55560);
#18029=VERTEX_POINT('',#55562);
#18030=VERTEX_POINT('',#55564);
#18031=VERTEX_POINT('',#55567);
#18032=VERTEX_POINT('',#55569);
#18033=VERTEX_POINT('',#55571);
#18034=VERTEX_POINT('',#55573);
#18035=VERTEX_POINT('',#55575);
#18036=VERTEX_POINT('',#55579);
#18037=VERTEX_POINT('',#55581);
#18038=VERTEX_POINT('',#55583);
#18039=VERTEX_POINT('',#55585);
#18040=VERTEX_POINT('',#55587);
#18041=VERTEX_POINT('',#55590);
#18042=VERTEX_POINT('',#55592);
#18043=VERTEX_POINT('',#55594);
#18044=VERTEX_POINT('',#55596);
#18045=VERTEX_POINT('',#55598);
#18046=VERTEX_POINT('',#55630);
#18047=VERTEX_POINT('',#55632);
#18048=VERTEX_POINT('',#55636);
#18049=VERTEX_POINT('',#55638);
#18050=VERTEX_POINT('',#55642);
#18051=VERTEX_POINT('',#55644);
#18052=VERTEX_POINT('',#55646);
#18053=VERTEX_POINT('',#55648);
#18054=VERTEX_POINT('',#55650);
#18055=VERTEX_POINT('',#55653);
#18056=VERTEX_POINT('',#55655);
#18057=VERTEX_POINT('',#55657);
#18058=VERTEX_POINT('',#55659);
#18059=VERTEX_POINT('',#55661);
#18060=VERTEX_POINT('',#55665);
#18061=VERTEX_POINT('',#55667);
#18062=VERTEX_POINT('',#55669);
#18063=VERTEX_POINT('',#55671);
#18064=VERTEX_POINT('',#55673);
#18065=VERTEX_POINT('',#55676);
#18066=VERTEX_POINT('',#55678);
#18067=VERTEX_POINT('',#55680);
#18068=VERTEX_POINT('',#55682);
#18069=VERTEX_POINT('',#55684);
#18070=VERTEX_POINT('',#55716);
#18071=VERTEX_POINT('',#55718);
#18072=VERTEX_POINT('',#55722);
#18073=VERTEX_POINT('',#55724);
#18074=VERTEX_POINT('',#55728);
#18075=VERTEX_POINT('',#55730);
#18076=VERTEX_POINT('',#55732);
#18077=VERTEX_POINT('',#55734);
#18078=VERTEX_POINT('',#55736);
#18079=VERTEX_POINT('',#55739);
#18080=VERTEX_POINT('',#55741);
#18081=VERTEX_POINT('',#55743);
#18082=VERTEX_POINT('',#55745);
#18083=VERTEX_POINT('',#55747);
#18084=VERTEX_POINT('',#55751);
#18085=VERTEX_POINT('',#55753);
#18086=VERTEX_POINT('',#55755);
#18087=VERTEX_POINT('',#55757);
#18088=VERTEX_POINT('',#55759);
#18089=VERTEX_POINT('',#55762);
#18090=VERTEX_POINT('',#55764);
#18091=VERTEX_POINT('',#55766);
#18092=VERTEX_POINT('',#55768);
#18093=VERTEX_POINT('',#55770);
#18094=VERTEX_POINT('',#55802);
#18095=VERTEX_POINT('',#55804);
#18096=VERTEX_POINT('',#55808);
#18097=VERTEX_POINT('',#55810);
#18098=VERTEX_POINT('',#55814);
#18099=VERTEX_POINT('',#55816);
#18100=VERTEX_POINT('',#55818);
#18101=VERTEX_POINT('',#55820);
#18102=VERTEX_POINT('',#55822);
#18103=VERTEX_POINT('',#55825);
#18104=VERTEX_POINT('',#55827);
#18105=VERTEX_POINT('',#55829);
#18106=VERTEX_POINT('',#55831);
#18107=VERTEX_POINT('',#55833);
#18108=VERTEX_POINT('',#55837);
#18109=VERTEX_POINT('',#55839);
#18110=VERTEX_POINT('',#55841);
#18111=VERTEX_POINT('',#55843);
#18112=VERTEX_POINT('',#55845);
#18113=VERTEX_POINT('',#55848);
#18114=VERTEX_POINT('',#55850);
#18115=VERTEX_POINT('',#55852);
#18116=VERTEX_POINT('',#55854);
#18117=VERTEX_POINT('',#55856);
#18118=VERTEX_POINT('',#55888);
#18119=VERTEX_POINT('',#55896);
#18120=VERTEX_POINT('',#55898);
#18121=VERTEX_POINT('',#55901);
#18122=VERTEX_POINT('',#55902);
#18123=VERTEX_POINT('',#55911);
#18124=VERTEX_POINT('',#55914);
#18125=VERTEX_POINT('',#55921);
#18126=VERTEX_POINT('',#55923);
#18127=VERTEX_POINT('',#55926);
#18128=VERTEX_POINT('',#55927);
#18129=VERTEX_POINT('',#55936);
#18130=VERTEX_POINT('',#55938);
#18131=VERTEX_POINT('',#55940);
#18132=VERTEX_POINT('',#55948);
#18133=VERTEX_POINT('',#55951);
#18134=VERTEX_POINT('',#55959);
#18135=VERTEX_POINT('',#55961);
#18136=VERTEX_POINT('',#55963);
#18137=VERTEX_POINT('',#55965);
#18138=VERTEX_POINT('',#55973);
#18139=VERTEX_POINT('',#55976);
#18140=VERTEX_POINT('',#55985);
#18141=VERTEX_POINT('',#55987);
#18142=VERTEX_POINT('',#55989);
#18143=VERTEX_POINT('',#55991);
#18144=VERTEX_POINT('',#55998);
#18145=VERTEX_POINT('',#56001);
#18146=VERTEX_POINT('',#56010);
#18147=VERTEX_POINT('',#56012);
#18148=VERTEX_POINT('',#56014);
#18149=VERTEX_POINT('',#56021);
#18150=VERTEX_POINT('',#56023);
#18151=VERTEX_POINT('',#56033);
#18152=VERTEX_POINT('',#56041);
#18153=VERTEX_POINT('',#56042);
#18154=VERTEX_POINT('',#56052);
#18155=VERTEX_POINT('',#56063);
#18156=VERTEX_POINT('',#56064);
#18157=VERTEX_POINT('',#56074);
#18158=VERTEX_POINT('',#56085);
#18159=VERTEX_POINT('',#56096);
#18160=VERTEX_POINT('',#56098);
#18161=VERTEX_POINT('',#56107);
#18162=VERTEX_POINT('',#56117);
#18163=VERTEX_POINT('',#56119);
#18164=VERTEX_POINT('',#56129);
#18165=VERTEX_POINT('',#56138);
#18166=VERTEX_POINT('',#56140);
#18167=VERTEX_POINT('',#56152);
#18168=VERTEX_POINT('',#56162);
#18169=VERTEX_POINT('',#56173);
#18170=VERTEX_POINT('',#56174);
#18171=VERTEX_POINT('',#56189);
#18172=VERTEX_POINT('',#56201);
#18173=VERTEX_POINT('',#56203);
#18174=VERTEX_POINT('',#56215);
#18175=VERTEX_POINT('',#56217);
#18176=VERTEX_POINT('',#56227);
#18177=VERTEX_POINT('',#56229);
#18178=VERTEX_POINT('',#57141);
#18179=VERTEX_POINT('',#57143);
#18180=VERTEX_POINT('',#57147);
#18181=VERTEX_POINT('',#57149);
#18182=VERTEX_POINT('',#57153);
#18183=VERTEX_POINT('',#57155);
#18184=VERTEX_POINT('',#57157);
#18185=VERTEX_POINT('',#57159);
#18186=VERTEX_POINT('',#57161);
#18187=VERTEX_POINT('',#57163);
#18188=VERTEX_POINT('',#57166);
#18189=VERTEX_POINT('',#57168);
#18190=VERTEX_POINT('',#57170);
#18191=VERTEX_POINT('',#57172);
#18192=VERTEX_POINT('',#57176);
#18193=VERTEX_POINT('',#57178);
#18194=VERTEX_POINT('',#57180);
#18195=VERTEX_POINT('',#57182);
#18196=VERTEX_POINT('',#57184);
#18197=VERTEX_POINT('',#57186);
#18198=VERTEX_POINT('',#57189);
#18199=VERTEX_POINT('',#57191);
#18200=VERTEX_POINT('',#57193);
#18201=VERTEX_POINT('',#57195);
#18202=VERTEX_POINT('',#57227);
#18203=VERTEX_POINT('',#57229);
#18204=VERTEX_POINT('',#57233);
#18205=VERTEX_POINT('',#57235);
#18206=VERTEX_POINT('',#57239);
#18207=VERTEX_POINT('',#57241);
#18208=VERTEX_POINT('',#57243);
#18209=VERTEX_POINT('',#57245);
#18210=VERTEX_POINT('',#57247);
#18211=VERTEX_POINT('',#57249);
#18212=VERTEX_POINT('',#57252);
#18213=VERTEX_POINT('',#57254);
#18214=VERTEX_POINT('',#57256);
#18215=VERTEX_POINT('',#57258);
#18216=VERTEX_POINT('',#57262);
#18217=VERTEX_POINT('',#57264);
#18218=VERTEX_POINT('',#57266);
#18219=VERTEX_POINT('',#57268);
#18220=VERTEX_POINT('',#57270);
#18221=VERTEX_POINT('',#57272);
#18222=VERTEX_POINT('',#57275);
#18223=VERTEX_POINT('',#57277);
#18224=VERTEX_POINT('',#57279);
#18225=VERTEX_POINT('',#57281);
#18226=VERTEX_POINT('',#57319);
#18227=VERTEX_POINT('',#57320);
#18228=VERTEX_POINT('',#57325);
#18229=VERTEX_POINT('',#57327);
#18230=VERTEX_POINT('',#57335);
#18231=VERTEX_POINT('',#57337);
#18232=VERTEX_POINT('',#57341);
#18233=VERTEX_POINT('',#57343);
#18234=VERTEX_POINT('',#57347);
#18235=VERTEX_POINT('',#57349);
#18236=VERTEX_POINT('',#57353);
#18237=VERTEX_POINT('',#57355);
#20856=EDGE_CURVE('',#17144,#17144,#16490,.T.);
#20857=EDGE_CURVE('',#17144,#17145,#6740,.T.);
#20858=EDGE_CURVE('',#17145,#17145,#16491,.T.);
#20859=EDGE_CURVE('',#17146,#17146,#16492,.T.);
#20860=EDGE_CURVE('',#17146,#17147,#6741,.T.);
#20861=EDGE_CURVE('',#17147,#17147,#16493,.T.);
#20862=EDGE_CURVE('',#17148,#17148,#16494,.T.);
#20863=EDGE_CURVE('',#17148,#17149,#6742,.T.);
#20864=EDGE_CURVE('',#17149,#17149,#16495,.T.);
#20865=EDGE_CURVE('',#17150,#17150,#16496,.T.);
#20866=EDGE_CURVE('',#17150,#17151,#6743,.T.);
#20867=EDGE_CURVE('',#17151,#17151,#16497,.T.);
#20868=EDGE_CURVE('',#17152,#17152,#16498,.T.);
#20869=EDGE_CURVE('',#17152,#17153,#6744,.T.);
#20870=EDGE_CURVE('',#17153,#17153,#16499,.T.);
#20871=EDGE_CURVE('',#17154,#17154,#16500,.T.);
#20872=EDGE_CURVE('',#17154,#17155,#6745,.T.);
#20873=EDGE_CURVE('',#17155,#17155,#16501,.T.);
#20874=EDGE_CURVE('',#17156,#17157,#16502,.T.);
#20875=EDGE_CURVE('',#17156,#17158,#6746,.T.);
#20876=EDGE_CURVE('',#17158,#17159,#16503,.T.);
#20877=EDGE_CURVE('',#17157,#17159,#6747,.T.);
#20878=EDGE_CURVE('',#17160,#17161,#16504,.T.);
#20879=EDGE_CURVE('',#17161,#17162,#6748,.T.);
#20880=EDGE_CURVE('',#17163,#17162,#16505,.T.);
#20881=EDGE_CURVE('',#17160,#17163,#6749,.T.);
#20882=EDGE_CURVE('',#17164,#17165,#16506,.T.);
#20883=EDGE_CURVE('',#17165,#17166,#6750,.T.);
#20884=EDGE_CURVE('',#17167,#17166,#16507,.T.);
#20885=EDGE_CURVE('',#17164,#17167,#6751,.T.);
#20886=EDGE_CURVE('',#17168,#17169,#16508,.T.);
#20887=EDGE_CURVE('',#17169,#17170,#6752,.T.);
#20888=EDGE_CURVE('',#17171,#17170,#16509,.T.);
#20889=EDGE_CURVE('',#17168,#17171,#6753,.T.);
#20890=EDGE_CURVE('',#17172,#17173,#16510,.T.);
#20891=EDGE_CURVE('',#17173,#17174,#6754,.T.);
#20892=EDGE_CURVE('',#17175,#17174,#16511,.T.);
#20893=EDGE_CURVE('',#17172,#17175,#6755,.T.);
#20894=EDGE_CURVE('',#17176,#17177,#16512,.T.);
#20895=EDGE_CURVE('',#17177,#17178,#6756,.T.);
#20896=EDGE_CURVE('',#17179,#17178,#16513,.T.);
#20897=EDGE_CURVE('',#17176,#17179,#6757,.T.);
#20898=EDGE_CURVE('',#17180,#17181,#16514,.T.);
#20899=EDGE_CURVE('',#17180,#17182,#6758,.T.);
#20900=EDGE_CURVE('',#17182,#17183,#16515,.T.);
#20901=EDGE_CURVE('',#17181,#17183,#6759,.T.);
#20902=EDGE_CURVE('',#17184,#17185,#16516,.T.);
#20903=EDGE_CURVE('',#17184,#17186,#6760,.T.);
#20904=EDGE_CURVE('',#17186,#17187,#16517,.T.);
#20905=EDGE_CURVE('',#17185,#17187,#6761,.T.);
#20906=EDGE_CURVE('',#17188,#17189,#16518,.T.);
#20907=EDGE_CURVE('',#17188,#17190,#6762,.T.);
#20908=EDGE_CURVE('',#17190,#17191,#16519,.T.);
#20909=EDGE_CURVE('',#17189,#17191,#6763,.T.);
#20910=EDGE_CURVE('',#17192,#17193,#16520,.T.);
#20911=EDGE_CURVE('',#17192,#17194,#6764,.T.);
#20912=EDGE_CURVE('',#17194,#17195,#16521,.T.);
#20913=EDGE_CURVE('',#17193,#17195,#6765,.T.);
#20914=EDGE_CURVE('',#17196,#17197,#16522,.T.);
#20915=EDGE_CURVE('',#17196,#17198,#6766,.T.);
#20916=EDGE_CURVE('',#17198,#17199,#16523,.T.);
#20917=EDGE_CURVE('',#17197,#17199,#6767,.T.);
#20918=EDGE_CURVE('',#17200,#17201,#16524,.T.);
#20919=EDGE_CURVE('',#17200,#17202,#6768,.T.);
#20920=EDGE_CURVE('',#17202,#17203,#16525,.T.);
#20921=EDGE_CURVE('',#17201,#17203,#6769,.T.);
#20922=EDGE_CURVE('',#17204,#17205,#16526,.T.);
#20923=EDGE_CURVE('',#17204,#17206,#6770,.T.);
#20924=EDGE_CURVE('',#17206,#17207,#16527,.T.);
#20925=EDGE_CURVE('',#17205,#17207,#6771,.T.);
#20926=EDGE_CURVE('',#17208,#17209,#16528,.T.);
#20927=EDGE_CURVE('',#17209,#17210,#6772,.T.);
#20928=EDGE_CURVE('',#17211,#17210,#16529,.T.);
#20929=EDGE_CURVE('',#17208,#17211,#6773,.T.);
#20930=EDGE_CURVE('',#17212,#17213,#16530,.T.);
#20931=EDGE_CURVE('',#17213,#17214,#6774,.T.);
#20932=EDGE_CURVE('',#17215,#17214,#16531,.T.);
#20933=EDGE_CURVE('',#17212,#17215,#6775,.T.);
#20934=EDGE_CURVE('',#17216,#17217,#16532,.T.);
#20935=EDGE_CURVE('',#17217,#17218,#6776,.T.);
#20936=EDGE_CURVE('',#17219,#17218,#16533,.T.);
#20937=EDGE_CURVE('',#17216,#17219,#6777,.T.);
#20938=EDGE_CURVE('',#17220,#17221,#16534,.T.);
#20939=EDGE_CURVE('',#17221,#17222,#6778,.T.);
#20940=EDGE_CURVE('',#17223,#17222,#16535,.T.);
#20941=EDGE_CURVE('',#17220,#17223,#6779,.T.);
#20942=EDGE_CURVE('',#17224,#17225,#16536,.T.);
#20943=EDGE_CURVE('',#17224,#17226,#6780,.T.);
#20944=EDGE_CURVE('',#17226,#17227,#16537,.T.);
#20945=EDGE_CURVE('',#17225,#17227,#6781,.T.);
#20946=EDGE_CURVE('',#17228,#17229,#16538,.T.);
#20947=EDGE_CURVE('',#17228,#17230,#6782,.T.);
#20948=EDGE_CURVE('',#17230,#17231,#16539,.T.);
#20949=EDGE_CURVE('',#17229,#17231,#6783,.T.);
#20950=EDGE_CURVE('',#17232,#17233,#16540,.T.);
#20951=EDGE_CURVE('',#17233,#17234,#6784,.T.);
#20952=EDGE_CURVE('',#17235,#17234,#16541,.T.);
#20953=EDGE_CURVE('',#17232,#17235,#6785,.T.);
#20954=EDGE_CURVE('',#17236,#17237,#16542,.T.);
#20955=EDGE_CURVE('',#17236,#17238,#6786,.T.);
#20956=EDGE_CURVE('',#17238,#17239,#16543,.T.);
#20957=EDGE_CURVE('',#17237,#17239,#6787,.T.);
#20958=EDGE_CURVE('',#17240,#17241,#16544,.T.);
#20959=EDGE_CURVE('',#17241,#17242,#6788,.T.);
#20960=EDGE_CURVE('',#17243,#17242,#16545,.T.);
#20961=EDGE_CURVE('',#17240,#17243,#6789,.T.);
#20962=EDGE_CURVE('',#17244,#17245,#16546,.T.);
#20963=EDGE_CURVE('',#17245,#17246,#6790,.T.);
#20964=EDGE_CURVE('',#17247,#17246,#16547,.T.);
#20965=EDGE_CURVE('',#17244,#17247,#6791,.T.);
#20966=EDGE_CURVE('',#17248,#17249,#16548,.T.);
#20967=EDGE_CURVE('',#17248,#17250,#6792,.T.);
#20968=EDGE_CURVE('',#17250,#17251,#16549,.T.);
#20969=EDGE_CURVE('',#17249,#17251,#6793,.T.);
#20970=EDGE_CURVE('',#17252,#17253,#16550,.T.);
#20971=EDGE_CURVE('',#17253,#17254,#6794,.T.);
#20972=EDGE_CURVE('',#17255,#17254,#16551,.T.);
#20973=EDGE_CURVE('',#17252,#17255,#6795,.T.);
#20974=EDGE_CURVE('',#17256,#17257,#16552,.T.);
#20975=EDGE_CURVE('',#17256,#17258,#6796,.T.);
#20976=EDGE_CURVE('',#17258,#17259,#16553,.T.);
#20977=EDGE_CURVE('',#17257,#17259,#6797,.T.);
#20978=EDGE_CURVE('',#17260,#17261,#16554,.T.);
#20979=EDGE_CURVE('',#17260,#17262,#6798,.T.);
#20980=EDGE_CURVE('',#17262,#17263,#16555,.T.);
#20981=EDGE_CURVE('',#17261,#17263,#6799,.T.);
#20982=EDGE_CURVE('',#17264,#17265,#16556,.T.);
#20983=EDGE_CURVE('',#17264,#17266,#6800,.T.);
#20984=EDGE_CURVE('',#17266,#17267,#16557,.T.);
#20985=EDGE_CURVE('',#17265,#17267,#6801,.T.);
#20986=EDGE_CURVE('',#17268,#17269,#16558,.T.);
#20987=EDGE_CURVE('',#17268,#17270,#6802,.T.);
#20988=EDGE_CURVE('',#17270,#17271,#16559,.T.);
#20989=EDGE_CURVE('',#17269,#17271,#6803,.T.);
#20990=EDGE_CURVE('',#17272,#17273,#16560,.T.);
#20991=EDGE_CURVE('',#17272,#17274,#6804,.T.);
#20992=EDGE_CURVE('',#17274,#17275,#16561,.T.);
#20993=EDGE_CURVE('',#17273,#17275,#6805,.T.);
#20994=EDGE_CURVE('',#17276,#17277,#16562,.T.);
#20995=EDGE_CURVE('',#17277,#17278,#6806,.T.);
#20996=EDGE_CURVE('',#17279,#17278,#16563,.T.);
#20997=EDGE_CURVE('',#17276,#17279,#6807,.T.);
#20998=EDGE_CURVE('',#17280,#17281,#16564,.T.);
#20999=EDGE_CURVE('',#17281,#17282,#6808,.T.);
#21000=EDGE_CURVE('',#17283,#17282,#16565,.T.);
#21001=EDGE_CURVE('',#17280,#17283,#6809,.T.);
#21002=EDGE_CURVE('',#17284,#17285,#16566,.T.);
#21003=EDGE_CURVE('',#17285,#17286,#6810,.T.);
#21004=EDGE_CURVE('',#17287,#17286,#16567,.T.);
#21005=EDGE_CURVE('',#17284,#17287,#6811,.T.);
#21006=EDGE_CURVE('',#17288,#17289,#16568,.T.);
#21007=EDGE_CURVE('',#17289,#17290,#6812,.T.);
#21008=EDGE_CURVE('',#17291,#17290,#16569,.T.);
#21009=EDGE_CURVE('',#17288,#17291,#6813,.T.);
#21010=EDGE_CURVE('',#17292,#17293,#16570,.T.);
#21011=EDGE_CURVE('',#17293,#17294,#6814,.T.);
#21012=EDGE_CURVE('',#17295,#17294,#16571,.T.);
#21013=EDGE_CURVE('',#17292,#17295,#6815,.T.);
#21014=EDGE_CURVE('',#17296,#17297,#16572,.T.);
#21015=EDGE_CURVE('',#17297,#17298,#6816,.T.);
#21016=EDGE_CURVE('',#17299,#17298,#16573,.T.);
#21017=EDGE_CURVE('',#17296,#17299,#6817,.T.);
#21018=EDGE_CURVE('',#17300,#17301,#16574,.T.);
#21019=EDGE_CURVE('',#17301,#17302,#6818,.T.);
#21020=EDGE_CURVE('',#17303,#17302,#16575,.T.);
#21021=EDGE_CURVE('',#17300,#17303,#6819,.T.);
#21022=EDGE_CURVE('',#17304,#17305,#16576,.T.);
#21023=EDGE_CURVE('',#17304,#17306,#6820,.T.);
#21024=EDGE_CURVE('',#17306,#17307,#16577,.T.);
#21025=EDGE_CURVE('',#17305,#17307,#6821,.T.);
#21026=EDGE_CURVE('',#17308,#17309,#16578,.T.);
#21027=EDGE_CURVE('',#17308,#17310,#6822,.T.);
#21028=EDGE_CURVE('',#17310,#17311,#16579,.T.);
#21029=EDGE_CURVE('',#17309,#17311,#6823,.T.);
#21030=EDGE_CURVE('',#17312,#17313,#16580,.T.);
#21031=EDGE_CURVE('',#17312,#17314,#6824,.T.);
#21032=EDGE_CURVE('',#17314,#17315,#16581,.T.);
#21033=EDGE_CURVE('',#17313,#17315,#6825,.T.);
#21034=EDGE_CURVE('',#17316,#17317,#16582,.T.);
#21035=EDGE_CURVE('',#17316,#17318,#6826,.T.);
#21036=EDGE_CURVE('',#17318,#17319,#16583,.T.);
#21037=EDGE_CURVE('',#17317,#17319,#6827,.T.);
#21038=EDGE_CURVE('',#17320,#17321,#16584,.T.);
#21039=EDGE_CURVE('',#17321,#17322,#6828,.T.);
#21040=EDGE_CURVE('',#17323,#17322,#16585,.T.);
#21041=EDGE_CURVE('',#17320,#17323,#6829,.T.);
#21042=EDGE_CURVE('',#17324,#17325,#16586,.T.);
#21043=EDGE_CURVE('',#17325,#17326,#6830,.T.);
#21044=EDGE_CURVE('',#17327,#17326,#16587,.T.);
#21045=EDGE_CURVE('',#17324,#17327,#6831,.T.);
#21046=EDGE_CURVE('',#17328,#17329,#16588,.T.);
#21047=EDGE_CURVE('',#17328,#17330,#6832,.T.);
#21048=EDGE_CURVE('',#17330,#17331,#16589,.T.);
#21049=EDGE_CURVE('',#17329,#17331,#6833,.T.);
#21050=EDGE_CURVE('',#17332,#17333,#16590,.T.);
#21051=EDGE_CURVE('',#17333,#17334,#6834,.T.);
#21052=EDGE_CURVE('',#17335,#17334,#16591,.T.);
#21053=EDGE_CURVE('',#17332,#17335,#6835,.T.);
#21054=EDGE_CURVE('',#17336,#17337,#16592,.T.);
#21055=EDGE_CURVE('',#17336,#17338,#6836,.T.);
#21056=EDGE_CURVE('',#17338,#17339,#16593,.T.);
#21057=EDGE_CURVE('',#17337,#17339,#6837,.T.);
#21058=EDGE_CURVE('',#17340,#17341,#16594,.T.);
#21059=EDGE_CURVE('',#17340,#17342,#6838,.T.);
#21060=EDGE_CURVE('',#17342,#17343,#16595,.T.);
#21061=EDGE_CURVE('',#17341,#17343,#6839,.T.);
#21062=EDGE_CURVE('',#17344,#17345,#16596,.T.);
#21063=EDGE_CURVE('',#17345,#17346,#6840,.T.);
#21064=EDGE_CURVE('',#17347,#17346,#16597,.T.);
#21065=EDGE_CURVE('',#17344,#17347,#6841,.T.);
#21066=EDGE_CURVE('',#17348,#17349,#16598,.T.);
#21067=EDGE_CURVE('',#17350,#17348,#6842,.T.);
#21068=EDGE_CURVE('',#17351,#17350,#16599,.T.);
#21069=EDGE_CURVE('',#17349,#17351,#6843,.T.);
#21070=EDGE_CURVE('',#17352,#17353,#16600,.T.);
#21071=EDGE_CURVE('',#17354,#17352,#6844,.T.);
#21072=EDGE_CURVE('',#17355,#17354,#16601,.T.);
#21073=EDGE_CURVE('',#17353,#17355,#6845,.T.);
#21074=EDGE_CURVE('',#17356,#17357,#16602,.T.);
#21075=EDGE_CURVE('',#17358,#17356,#6846,.T.);
#21076=EDGE_CURVE('',#17359,#17358,#16603,.T.);
#21077=EDGE_CURVE('',#17357,#17359,#6847,.T.);
#21078=EDGE_CURVE('',#17360,#17361,#16604,.T.);
#21079=EDGE_CURVE('',#17362,#17360,#6848,.T.);
#21080=EDGE_CURVE('',#17363,#17362,#16605,.T.);
#21081=EDGE_CURVE('',#17361,#17363,#6849,.T.);
#21082=EDGE_CURVE('',#17364,#17365,#16606,.T.);
#21083=EDGE_CURVE('',#17366,#17364,#6850,.T.);
#21084=EDGE_CURVE('',#17367,#17366,#16607,.T.);
#21085=EDGE_CURVE('',#17365,#17367,#6851,.T.);
#21086=EDGE_CURVE('',#17368,#17369,#16608,.T.);
#21087=EDGE_CURVE('',#17370,#17368,#6852,.T.);
#21088=EDGE_CURVE('',#17371,#17370,#16609,.T.);
#21089=EDGE_CURVE('',#17369,#17371,#6853,.T.);
#21090=EDGE_CURVE('',#17372,#17373,#16610,.T.);
#21091=EDGE_CURVE('',#17374,#17372,#6854,.T.);
#21092=EDGE_CURVE('',#17375,#17374,#16611,.T.);
#21093=EDGE_CURVE('',#17373,#17375,#6855,.T.);
#21094=EDGE_CURVE('',#17376,#17377,#16612,.T.);
#21095=EDGE_CURVE('',#17378,#17376,#6856,.T.);
#21096=EDGE_CURVE('',#17379,#17378,#16613,.T.);
#21097=EDGE_CURVE('',#17377,#17379,#6857,.T.);
#21098=EDGE_CURVE('',#17380,#17381,#16614,.T.);
#21099=EDGE_CURVE('',#17382,#17380,#6858,.T.);
#21100=EDGE_CURVE('',#17383,#17382,#16615,.T.);
#21101=EDGE_CURVE('',#17381,#17383,#6859,.T.);
#21102=EDGE_CURVE('',#17384,#17385,#16616,.T.);
#21103=EDGE_CURVE('',#17386,#17384,#6860,.T.);
#21104=EDGE_CURVE('',#17387,#17386,#16617,.T.);
#21105=EDGE_CURVE('',#17385,#17387,#6861,.T.);
#21106=EDGE_CURVE('',#17388,#17389,#16618,.T.);
#21107=EDGE_CURVE('',#17390,#17388,#6862,.T.);
#21108=EDGE_CURVE('',#17391,#17390,#16619,.T.);
#21109=EDGE_CURVE('',#17389,#17391,#6863,.T.);
#21110=EDGE_CURVE('',#17392,#17393,#16620,.T.);
#21111=EDGE_CURVE('',#17394,#17392,#6864,.T.);
#21112=EDGE_CURVE('',#17395,#17394,#16621,.T.);
#21113=EDGE_CURVE('',#17393,#17395,#6865,.T.);
#21114=EDGE_CURVE('',#17396,#17397,#16622,.T.);
#21115=EDGE_CURVE('',#17398,#17396,#6866,.T.);
#21116=EDGE_CURVE('',#17399,#17398,#16623,.T.);
#21117=EDGE_CURVE('',#17397,#17399,#6867,.T.);
#21118=EDGE_CURVE('',#17400,#17401,#16624,.T.);
#21119=EDGE_CURVE('',#17402,#17400,#6868,.T.);
#21120=EDGE_CURVE('',#17403,#17402,#16625,.T.);
#21121=EDGE_CURVE('',#17401,#17403,#6869,.T.);
#21122=EDGE_CURVE('',#17404,#17405,#16626,.T.);
#21123=EDGE_CURVE('',#17406,#17404,#6870,.T.);
#21124=EDGE_CURVE('',#17407,#17406,#16627,.T.);
#21125=EDGE_CURVE('',#17405,#17407,#6871,.T.);
#21126=EDGE_CURVE('',#17408,#17409,#16628,.T.);
#21127=EDGE_CURVE('',#17410,#17408,#6872,.T.);
#21128=EDGE_CURVE('',#17411,#17410,#16629,.T.);
#21129=EDGE_CURVE('',#17409,#17411,#6873,.T.);
#21130=EDGE_CURVE('',#17412,#17413,#16630,.T.);
#21131=EDGE_CURVE('',#17414,#17412,#6874,.T.);
#21132=EDGE_CURVE('',#17415,#17414,#16631,.T.);
#21133=EDGE_CURVE('',#17413,#17415,#6875,.T.);
#21134=EDGE_CURVE('',#17416,#17417,#16632,.T.);
#21135=EDGE_CURVE('',#17418,#17416,#6876,.T.);
#21136=EDGE_CURVE('',#17419,#17418,#16633,.T.);
#21137=EDGE_CURVE('',#17417,#17419,#6877,.T.);
#21138=EDGE_CURVE('',#17420,#17421,#2193,.T.);
#21139=EDGE_CURVE('',#17420,#17422,#6878,.T.);
#21140=EDGE_CURVE('',#17423,#17422,#2194,.T.);
#21141=EDGE_CURVE('',#17423,#17421,#6879,.T.);
#21142=EDGE_CURVE('',#17424,#17425,#2195,.T.);
#21143=EDGE_CURVE('',#17424,#17426,#6880,.T.);
#21144=EDGE_CURVE('',#17427,#17426,#2196,.T.);
#21145=EDGE_CURVE('',#17427,#17425,#6881,.T.);
#21146=EDGE_CURVE('',#17428,#17429,#2197,.T.);
#21147=EDGE_CURVE('',#17429,#17430,#6882,.T.);
#21148=EDGE_CURVE('',#17431,#17430,#2198,.T.);
#21149=EDGE_CURVE('',#17431,#17428,#6883,.T.);
#21150=EDGE_CURVE('',#17432,#17433,#2199,.T.);
#21151=EDGE_CURVE('',#17432,#17434,#6884,.T.);
#21152=EDGE_CURVE('',#17435,#17434,#2200,.T.);
#21153=EDGE_CURVE('',#17435,#17433,#6885,.T.);
#21154=EDGE_CURVE('',#17436,#17437,#2201,.T.);
#21155=EDGE_CURVE('',#17437,#17438,#6886,.T.);
#21156=EDGE_CURVE('',#17439,#17438,#2202,.T.);
#21157=EDGE_CURVE('',#17439,#17436,#6887,.T.);
#21158=EDGE_CURVE('',#17440,#17440,#16634,.T.);
#21159=EDGE_CURVE('',#17440,#17441,#6888,.T.);
#21160=EDGE_CURVE('',#17441,#17441,#16635,.T.);
#21161=EDGE_CURVE('',#17442,#17442,#16636,.T.);
#21162=EDGE_CURVE('',#17442,#17443,#6889,.T.);
#21163=EDGE_CURVE('',#17443,#17443,#16637,.T.);
#21164=EDGE_CURVE('',#17444,#17444,#16638,.T.);
#21165=EDGE_CURVE('',#17444,#17445,#6890,.T.);
#21166=EDGE_CURVE('',#17445,#17445,#16639,.T.);
#21167=EDGE_CURVE('',#17446,#17446,#16640,.T.);
#21168=EDGE_CURVE('',#17446,#17447,#6891,.T.);
#21169=EDGE_CURVE('',#17447,#17447,#16641,.T.);
#21170=EDGE_CURVE('',#17448,#17448,#16642,.T.);
#21171=EDGE_CURVE('',#17448,#17449,#16643,.T.);
#21172=EDGE_CURVE('',#17449,#17449,#16644,.T.);
#21173=EDGE_CURVE('',#17450,#17450,#16645,.T.);
#21174=EDGE_CURVE('',#17450,#17451,#16646,.T.);
#21175=EDGE_CURVE('',#17451,#17451,#16647,.T.);
#21176=EDGE_CURVE('',#17452,#17452,#16648,.T.);
#21177=EDGE_CURVE('',#17452,#17450,#16649,.T.);
#21178=EDGE_CURVE('',#17453,#17453,#16650,.T.);
#21179=EDGE_CURVE('',#17453,#17448,#16651,.T.);
#21180=EDGE_CURVE('',#17454,#17454,#16652,.T.);
#21181=EDGE_CURVE('',#17454,#17455,#6892,.T.);
#21182=EDGE_CURVE('',#17455,#17455,#16653,.T.);
#21183=EDGE_CURVE('',#17456,#17456,#16654,.T.);
#21184=EDGE_CURVE('',#17456,#17457,#6893,.T.);
#21185=EDGE_CURVE('',#17457,#17457,#16655,.T.);
#21186=EDGE_CURVE('',#17458,#17458,#16656,.T.);
#21187=EDGE_CURVE('',#17458,#17459,#6894,.T.);
#21188=EDGE_CURVE('',#17459,#17459,#16657,.T.);
#21189=EDGE_CURVE('',#17460,#17460,#16658,.T.);
#21190=EDGE_CURVE('',#17460,#17461,#6895,.T.);
#21191=EDGE_CURVE('',#17461,#17461,#16659,.T.);
#21192=EDGE_CURVE('',#17462,#17463,#2203,.T.);
#21193=EDGE_CURVE('',#17463,#17464,#6896,.T.);
#21194=EDGE_CURVE('',#17465,#17464,#2204,.T.);
#21195=EDGE_CURVE('',#17465,#17462,#6897,.T.);
#21196=EDGE_CURVE('',#17466,#17467,#6898,.T.);
#21197=EDGE_CURVE('',#17466,#17468,#6899,.T.);
#21198=EDGE_CURVE('',#17469,#17468,#6900,.T.);
#21199=EDGE_CURVE('',#17470,#17469,#16660,.T.);
#21200=EDGE_CURVE('',#17471,#17470,#6901,.T.);
#21201=EDGE_CURVE('',#17472,#17471,#16661,.T.);
#21202=EDGE_CURVE('',#17473,#17472,#6902,.T.);
#21203=EDGE_CURVE('',#17474,#17473,#6903,.T.);
#21204=EDGE_CURVE('',#17475,#17474,#6904,.T.);
#21205=EDGE_CURVE('',#17476,#17475,#6905,.T.);
#21206=EDGE_CURVE('',#17477,#17476,#6906,.T.);
#21207=EDGE_CURVE('',#17478,#17477,#6907,.T.);
#21208=EDGE_CURVE('',#17479,#17478,#6908,.T.);
#21209=EDGE_CURVE('',#17480,#17479,#6909,.T.);
#21210=EDGE_CURVE('',#17481,#17480,#6910,.T.);
#21211=EDGE_CURVE('',#17482,#17481,#6911,.T.);
#21212=EDGE_CURVE('',#17483,#17482,#6912,.T.);
#21213=EDGE_CURVE('',#17484,#17483,#16662,.T.);
#21214=EDGE_CURVE('',#17484,#17485,#6913,.T.);
#21215=EDGE_CURVE('',#17486,#17485,#16663,.T.);
#21216=EDGE_CURVE('',#17487,#17486,#6914,.T.);
#21217=EDGE_CURVE('',#17487,#17488,#6915,.T.);
#21218=EDGE_CURVE('',#17489,#17488,#6916,.T.);
#21219=EDGE_CURVE('',#17490,#17489,#6917,.T.);
#21220=EDGE_CURVE('',#17491,#17490,#6918,.T.);
#21221=EDGE_CURVE('',#17492,#17491,#6919,.T.);
#21222=EDGE_CURVE('',#17493,#17492,#6920,.T.);
#21223=EDGE_CURVE('',#17467,#17493,#6921,.T.);
#21224=EDGE_CURVE('',#17494,#17495,#6922,.T.);
#21225=EDGE_CURVE('',#17494,#17496,#6923,.T.);
#21226=EDGE_CURVE('',#17497,#17496,#6924,.T.);
#21227=EDGE_CURVE('',#17497,#17498,#6925,.T.);
#21228=EDGE_CURVE('',#17499,#17498,#6926,.T.);
#21229=EDGE_CURVE('',#17500,#17499,#6927,.T.);
#21230=EDGE_CURVE('',#17501,#17500,#6928,.T.);
#21231=EDGE_CURVE('',#17501,#17495,#6929,.T.);
#21232=EDGE_CURVE('',#17502,#17503,#6930,.T.);
#21233=EDGE_CURVE('',#17502,#17504,#6931,.T.);
#21234=EDGE_CURVE('',#17505,#17504,#6932,.T.);
#21235=EDGE_CURVE('',#17505,#17506,#6933,.T.);
#21236=EDGE_CURVE('',#17507,#17506,#6934,.T.);
#21237=EDGE_CURVE('',#17508,#17507,#6935,.T.);
#21238=EDGE_CURVE('',#17509,#17508,#6936,.T.);
#21239=EDGE_CURVE('',#17509,#17503,#6937,.T.);
#21240=EDGE_CURVE('',#17510,#17511,#6938,.T.);
#21241=EDGE_CURVE('',#17510,#17512,#6939,.T.);
#21242=EDGE_CURVE('',#17513,#17512,#6940,.T.);
#21243=EDGE_CURVE('',#17513,#17514,#6941,.T.);
#21244=EDGE_CURVE('',#17515,#17514,#6942,.T.);
#21245=EDGE_CURVE('',#17516,#17515,#6943,.T.);
#21246=EDGE_CURVE('',#17517,#17516,#6944,.T.);
#21247=EDGE_CURVE('',#17517,#17511,#6945,.T.);
#21248=EDGE_CURVE('',#17518,#17519,#6946,.T.);
#21249=EDGE_CURVE('',#17518,#17520,#6947,.T.);
#21250=EDGE_CURVE('',#17521,#17520,#6948,.T.);
#21251=EDGE_CURVE('',#17521,#17522,#6949,.T.);
#21252=EDGE_CURVE('',#17523,#17522,#6950,.T.);
#21253=EDGE_CURVE('',#17524,#17523,#6951,.T.);
#21254=EDGE_CURVE('',#17525,#17524,#6952,.T.);
#21255=EDGE_CURVE('',#17525,#17519,#6953,.T.);
#21256=EDGE_CURVE('',#17526,#17527,#6954,.T.);
#21257=EDGE_CURVE('',#17526,#17528,#6955,.T.);
#21258=EDGE_CURVE('',#17528,#17529,#6956,.T.);
#21259=EDGE_CURVE('',#17529,#17530,#6957,.T.);
#21260=EDGE_CURVE('',#17530,#17531,#6958,.T.);
#21261=EDGE_CURVE('',#17531,#17532,#6959,.T.);
#21262=EDGE_CURVE('',#17532,#17533,#6960,.T.);
#21263=EDGE_CURVE('',#17533,#17534,#6961,.T.);
#21264=EDGE_CURVE('',#17535,#17534,#6962,.T.);
#21265=EDGE_CURVE('',#17536,#17535,#6963,.T.);
#21266=EDGE_CURVE('',#17537,#17536,#16664,.T.);
#21267=EDGE_CURVE('',#17538,#17537,#6964,.T.);
#21268=EDGE_CURVE('',#17539,#17538,#16665,.T.);
#21269=EDGE_CURVE('',#17540,#17539,#6965,.T.);
#21270=EDGE_CURVE('',#17540,#17541,#6966,.T.);
#21271=EDGE_CURVE('',#17541,#17542,#6967,.T.);
#21272=EDGE_CURVE('',#17542,#17543,#6968,.T.);
#21273=EDGE_CURVE('',#17543,#17544,#6969,.T.);
#21274=EDGE_CURVE('',#17544,#17545,#6970,.T.);
#21275=EDGE_CURVE('',#17545,#17546,#6971,.T.);
#21276=EDGE_CURVE('',#17546,#17547,#6972,.T.);
#21277=EDGE_CURVE('',#17547,#17548,#6973,.T.);
#21278=EDGE_CURVE('',#17548,#17549,#6974,.T.);
#21279=EDGE_CURVE('',#17550,#17549,#6975,.T.);
#21280=EDGE_CURVE('',#17551,#17550,#16666,.T.);
#21281=EDGE_CURVE('',#17551,#17552,#6976,.T.);
#21282=EDGE_CURVE('',#17553,#17552,#16667,.T.);
#21283=EDGE_CURVE('',#17527,#17553,#6977,.T.);
#21284=EDGE_CURVE('',#17554,#17555,#6978,.T.);
#21285=EDGE_CURVE('',#17556,#17554,#6979,.T.);
#21286=EDGE_CURVE('',#17556,#17557,#6980,.T.);
#21287=EDGE_CURVE('',#17555,#17557,#6981,.T.);
#21288=EDGE_CURVE('',#17558,#17559,#6982,.T.);
#21289=EDGE_CURVE('',#17560,#17558,#6983,.T.);
#21290=EDGE_CURVE('',#17560,#17561,#6984,.T.);
#21291=EDGE_CURVE('',#17559,#17561,#6985,.T.);
#21292=EDGE_CURVE('',#17562,#17563,#6986,.T.);
#21293=EDGE_CURVE('',#17564,#17562,#6987,.T.);
#21294=EDGE_CURVE('',#17564,#17565,#6988,.T.);
#21295=EDGE_CURVE('',#17563,#17565,#6989,.T.);
#21296=EDGE_CURVE('',#17566,#17567,#6990,.T.);
#21297=EDGE_CURVE('',#17568,#17566,#6991,.T.);
#21298=EDGE_CURVE('',#17568,#17569,#6992,.T.);
#21299=EDGE_CURVE('',#17567,#17569,#6993,.T.);
#21300=EDGE_CURVE('',#17466,#17526,#6994,.T.);
#21301=EDGE_CURVE('',#17468,#17527,#6995,.T.);
#21302=EDGE_CURVE('',#17488,#17534,#6996,.T.);
#21303=EDGE_CURVE('',#17535,#17487,#6997,.T.);
#21304=EDGE_CURVE('',#17570,#17571,#6998,.T.);
#21305=EDGE_CURVE('',#17572,#17570,#6999,.T.);
#21306=EDGE_CURVE('',#17573,#17572,#7000,.T.);
#21307=EDGE_CURVE('',#17574,#17573,#16668,.T.);
#21308=EDGE_CURVE('',#17575,#17574,#7001,.T.);
#21309=EDGE_CURVE('',#17571,#17575,#16669,.T.);
#21310=EDGE_CURVE('',#17576,#17577,#7002,.T.);
#21311=EDGE_CURVE('',#17577,#17578,#7003,.T.);
#21312=EDGE_CURVE('',#17579,#17578,#7004,.T.);
#21313=EDGE_CURVE('',#17579,#17580,#7005,.T.);
#21314=EDGE_CURVE('',#17580,#17581,#7006,.T.);
#21315=EDGE_CURVE('',#17581,#17582,#7007,.T.);
#21316=EDGE_CURVE('',#17582,#17583,#7008,.T.);
#21317=EDGE_CURVE('',#17583,#17576,#7009,.T.);
#21318=EDGE_CURVE('',#17584,#17585,#7010,.T.);
#21319=EDGE_CURVE('',#17584,#17586,#7011,.T.);
#21320=EDGE_CURVE('',#17587,#17586,#7012,.T.);
#21321=EDGE_CURVE('',#17587,#17588,#7013,.T.);
#21322=EDGE_CURVE('',#17589,#17588,#7014,.T.);
#21323=EDGE_CURVE('',#17589,#17590,#7015,.T.);
#21324=EDGE_CURVE('',#17590,#17591,#7016,.T.);
#21325=EDGE_CURVE('',#17591,#17585,#7017,.T.);
#21326=EDGE_CURVE('',#17592,#17593,#7018,.T.);
#21327=EDGE_CURVE('',#17592,#17594,#7019,.T.);
#21328=EDGE_CURVE('',#17594,#17595,#16670,.T.);
#21329=EDGE_CURVE('',#17595,#17596,#7020,.T.);
#21330=EDGE_CURVE('',#17596,#17597,#16671,.T.);
#21331=EDGE_CURVE('',#17597,#17593,#7021,.T.);
#21332=EDGE_CURVE('',#17598,#17599,#7022,.T.);
#21333=EDGE_CURVE('',#17600,#17598,#7023,.T.);
#21334=EDGE_CURVE('',#17600,#17601,#7024,.T.);
#21335=EDGE_CURVE('',#17599,#17601,#7025,.T.);
#21336=EDGE_CURVE('',#17602,#17603,#7026,.T.);
#21337=EDGE_CURVE('',#17603,#17604,#7027,.T.);
#21338=EDGE_CURVE('',#17604,#17605,#7028,.T.);
#21339=EDGE_CURVE('',#17602,#17605,#7029,.T.);
#21340=EDGE_CURVE('',#17481,#17541,#7030,.T.);
#21341=EDGE_CURVE('',#17482,#17540,#7031,.T.);
#21342=EDGE_CURVE('',#17474,#17548,#7032,.T.);
#21343=EDGE_CURVE('',#17549,#17473,#7033,.T.);
#21344=EDGE_CURVE('',#17606,#17607,#7034,.T.);
#21345=EDGE_CURVE('',#17606,#17608,#7035,.T.);
#21346=EDGE_CURVE('',#17609,#17608,#7036,.T.);
#21347=EDGE_CURVE('',#17609,#17610,#7037,.T.);
#21348=EDGE_CURVE('',#17610,#17611,#7038,.T.);
#21349=EDGE_CURVE('',#17612,#17611,#7039,.T.);
#21350=EDGE_CURVE('',#17613,#17612,#16672,.T.);
#21351=EDGE_CURVE('',#17613,#17614,#7040,.T.);
#21352=EDGE_CURVE('',#17615,#17614,#16673,.T.);
#21353=EDGE_CURVE('',#17607,#17615,#7041,.T.);
#21354=EDGE_CURVE('',#17616,#17347,#7042,.T.);
#21355=EDGE_CURVE('',#17617,#17346,#7043,.T.);
#21356=EDGE_CURVE('',#17617,#17616,#16674,.T.);
#21357=EDGE_CURVE('',#17618,#17335,#7044,.T.);
#21358=EDGE_CURVE('',#17619,#17334,#7045,.T.);
#21359=EDGE_CURVE('',#17619,#17618,#16675,.T.);
#21360=EDGE_CURVE('',#17620,#17327,#7046,.T.);
#21361=EDGE_CURVE('',#17621,#17326,#7047,.T.);
#21362=EDGE_CURVE('',#17621,#17620,#16676,.T.);
#21363=EDGE_CURVE('',#17622,#17323,#7048,.T.);
#21364=EDGE_CURVE('',#17623,#17322,#7049,.T.);
#21365=EDGE_CURVE('',#17623,#17622,#16677,.T.);
#21366=EDGE_CURVE('',#17624,#17303,#7050,.T.);
#21367=EDGE_CURVE('',#17625,#17302,#7051,.T.);
#21368=EDGE_CURVE('',#17625,#17624,#16678,.T.);
#21369=EDGE_CURVE('',#17626,#17299,#7052,.T.);
#21370=EDGE_CURVE('',#17627,#17298,#7053,.T.);
#21371=EDGE_CURVE('',#17627,#17626,#16679,.T.);
#21372=EDGE_CURVE('',#17628,#17295,#7054,.T.);
#21373=EDGE_CURVE('',#17629,#17294,#7055,.T.);
#21374=EDGE_CURVE('',#17629,#17628,#16680,.T.);
#21375=EDGE_CURVE('',#17630,#17291,#7056,.T.);
#21376=EDGE_CURVE('',#17631,#17290,#7057,.T.);
#21377=EDGE_CURVE('',#17631,#17630,#16681,.T.);
#21378=EDGE_CURVE('',#17632,#17287,#7058,.T.);
#21379=EDGE_CURVE('',#17633,#17286,#7059,.T.);
#21380=EDGE_CURVE('',#17633,#17632,#16682,.T.);
#21381=EDGE_CURVE('',#17634,#17283,#7060,.T.);
#21382=EDGE_CURVE('',#17635,#17282,#7061,.T.);
#21383=EDGE_CURVE('',#17635,#17634,#16683,.T.);
#21384=EDGE_CURVE('',#17636,#17279,#7062,.T.);
#21385=EDGE_CURVE('',#17637,#17278,#7063,.T.);
#21386=EDGE_CURVE('',#17637,#17636,#16684,.T.);
#21387=EDGE_CURVE('',#17638,#17255,#7064,.T.);
#21388=EDGE_CURVE('',#17639,#17254,#7065,.T.);
#21389=EDGE_CURVE('',#17639,#17638,#16685,.T.);
#21390=EDGE_CURVE('',#17246,#17640,#7066,.T.);
#21391=EDGE_CURVE('',#17640,#17641,#16686,.T.);
#21392=EDGE_CURVE('',#17247,#17641,#7067,.T.);
#21393=EDGE_CURVE('',#17242,#17642,#7068,.T.);
#21394=EDGE_CURVE('',#17642,#17643,#16687,.T.);
#21395=EDGE_CURVE('',#17243,#17643,#7069,.T.);
#21396=EDGE_CURVE('',#17234,#17644,#7070,.T.);
#21397=EDGE_CURVE('',#17644,#17645,#16688,.T.);
#21398=EDGE_CURVE('',#17235,#17645,#7071,.T.);
#21399=EDGE_CURVE('',#17222,#17646,#7072,.T.);
#21400=EDGE_CURVE('',#17646,#17647,#16689,.T.);
#21401=EDGE_CURVE('',#17223,#17647,#7073,.T.);
#21402=EDGE_CURVE('',#17218,#17648,#7074,.T.);
#21403=EDGE_CURVE('',#17648,#17649,#16690,.T.);
#21404=EDGE_CURVE('',#17219,#17649,#7075,.T.);
#21405=EDGE_CURVE('',#17214,#17650,#7076,.T.);
#21406=EDGE_CURVE('',#17650,#17651,#16691,.T.);
#21407=EDGE_CURVE('',#17215,#17651,#7077,.T.);
#21408=EDGE_CURVE('',#17210,#17652,#7078,.T.);
#21409=EDGE_CURVE('',#17652,#17653,#16692,.T.);
#21410=EDGE_CURVE('',#17211,#17653,#7079,.T.);
#21411=EDGE_CURVE('',#17178,#17654,#7080,.T.);
#21412=EDGE_CURVE('',#17654,#17655,#16693,.T.);
#21413=EDGE_CURVE('',#17179,#17655,#7081,.T.);
#21414=EDGE_CURVE('',#17174,#17656,#7082,.T.);
#21415=EDGE_CURVE('',#17656,#17657,#16694,.T.);
#21416=EDGE_CURVE('',#17175,#17657,#7083,.T.);
#21417=EDGE_CURVE('',#17170,#17658,#7084,.T.);
#21418=EDGE_CURVE('',#17658,#17659,#16695,.T.);
#21419=EDGE_CURVE('',#17171,#17659,#7085,.T.);
#21420=EDGE_CURVE('',#17166,#17660,#7086,.T.);
#21421=EDGE_CURVE('',#17660,#17661,#16696,.T.);
#21422=EDGE_CURVE('',#17167,#17661,#7087,.T.);
#21423=EDGE_CURVE('',#17162,#17662,#7088,.T.);
#21424=EDGE_CURVE('',#17662,#17663,#16697,.T.);
#21425=EDGE_CURVE('',#17163,#17663,#7089,.T.);
#21426=EDGE_CURVE('',#17664,#17158,#7090,.T.);
#21427=EDGE_CURVE('',#17665,#17664,#16698,.T.);
#21428=EDGE_CURVE('',#17665,#17159,#7091,.T.);
#21429=EDGE_CURVE('',#17666,#17182,#7092,.T.);
#21430=EDGE_CURVE('',#17667,#17666,#16699,.T.);
#21431=EDGE_CURVE('',#17667,#17183,#7093,.T.);
#21432=EDGE_CURVE('',#17668,#17186,#7094,.T.);
#21433=EDGE_CURVE('',#17669,#17668,#16700,.T.);
#21434=EDGE_CURVE('',#17669,#17187,#7095,.T.);
#21435=EDGE_CURVE('',#17670,#17190,#7096,.T.);
#21436=EDGE_CURVE('',#17671,#17670,#16701,.T.);
#21437=EDGE_CURVE('',#17671,#17191,#7097,.T.);
#21438=EDGE_CURVE('',#17672,#17194,#7098,.T.);
#21439=EDGE_CURVE('',#17673,#17672,#16702,.T.);
#21440=EDGE_CURVE('',#17673,#17195,#7099,.T.);
#21441=EDGE_CURVE('',#17674,#17198,#7100,.T.);
#21442=EDGE_CURVE('',#17675,#17674,#16703,.T.);
#21443=EDGE_CURVE('',#17675,#17199,#7101,.T.);
#21444=EDGE_CURVE('',#17676,#17202,#7102,.T.);
#21445=EDGE_CURVE('',#17677,#17676,#16704,.T.);
#21446=EDGE_CURVE('',#17677,#17203,#7103,.T.);
#21447=EDGE_CURVE('',#17678,#17206,#7104,.T.);
#21448=EDGE_CURVE('',#17679,#17678,#16705,.T.);
#21449=EDGE_CURVE('',#17679,#17207,#7105,.T.);
#21450=EDGE_CURVE('',#17680,#17226,#7106,.T.);
#21451=EDGE_CURVE('',#17681,#17680,#16706,.T.);
#21452=EDGE_CURVE('',#17681,#17227,#7107,.T.);
#21453=EDGE_CURVE('',#17682,#17230,#7108,.T.);
#21454=EDGE_CURVE('',#17683,#17682,#16707,.T.);
#21455=EDGE_CURVE('',#17683,#17231,#7109,.T.);
#21456=EDGE_CURVE('',#17684,#17238,#7110,.T.);
#21457=EDGE_CURVE('',#17685,#17684,#16708,.T.);
#21458=EDGE_CURVE('',#17685,#17239,#7111,.T.);
#21459=EDGE_CURVE('',#17686,#17250,#7112,.T.);
#21460=EDGE_CURVE('',#17687,#17686,#16709,.T.);
#21461=EDGE_CURVE('',#17687,#17251,#7113,.T.);
#21462=EDGE_CURVE('',#17259,#17688,#7114,.T.);
#21463=EDGE_CURVE('',#17258,#17689,#7115,.T.);
#21464=EDGE_CURVE('',#17688,#17689,#16710,.T.);
#21465=EDGE_CURVE('',#17263,#17690,#7116,.T.);
#21466=EDGE_CURVE('',#17262,#17691,#7117,.T.);
#21467=EDGE_CURVE('',#17690,#17691,#16711,.T.);
#21468=EDGE_CURVE('',#17267,#17692,#7118,.T.);
#21469=EDGE_CURVE('',#17266,#17693,#7119,.T.);
#21470=EDGE_CURVE('',#17692,#17693,#16712,.T.);
#21471=EDGE_CURVE('',#17271,#17694,#7120,.T.);
#21472=EDGE_CURVE('',#17270,#17695,#7121,.T.);
#21473=EDGE_CURVE('',#17694,#17695,#16713,.T.);
#21474=EDGE_CURVE('',#17275,#17696,#7122,.T.);
#21475=EDGE_CURVE('',#17274,#17697,#7123,.T.);
#21476=EDGE_CURVE('',#17696,#17697,#16714,.T.);
#21477=EDGE_CURVE('',#17307,#17698,#7124,.T.);
#21478=EDGE_CURVE('',#17306,#17699,#7125,.T.);
#21479=EDGE_CURVE('',#17698,#17699,#16715,.T.);
#21480=EDGE_CURVE('',#17311,#17700,#7126,.T.);
#21481=EDGE_CURVE('',#17310,#17701,#7127,.T.);
#21482=EDGE_CURVE('',#17700,#17701,#16716,.T.);
#21483=EDGE_CURVE('',#17315,#17702,#7128,.T.);
#21484=EDGE_CURVE('',#17314,#17703,#7129,.T.);
#21485=EDGE_CURVE('',#17702,#17703,#16717,.T.);
#21486=EDGE_CURVE('',#17319,#17704,#7130,.T.);
#21487=EDGE_CURVE('',#17318,#17705,#7131,.T.);
#21488=EDGE_CURVE('',#17704,#17705,#16718,.T.);
#21489=EDGE_CURVE('',#17331,#17706,#7132,.T.);
#21490=EDGE_CURVE('',#17330,#17707,#7133,.T.);
#21491=EDGE_CURVE('',#17706,#17707,#16719,.T.);
#21492=EDGE_CURVE('',#17339,#17708,#7134,.T.);
#21493=EDGE_CURVE('',#17338,#17709,#7135,.T.);
#21494=EDGE_CURVE('',#17708,#17709,#16720,.T.);
#21495=EDGE_CURVE('',#17343,#17710,#7136,.T.);
#21496=EDGE_CURVE('',#17342,#17711,#7137,.T.);
#21497=EDGE_CURVE('',#17710,#17711,#16721,.T.);
#21498=EDGE_CURVE('',#17712,#17713,#7138,.T.);
#21499=EDGE_CURVE('',#17713,#17714,#7139,.T.);
#21500=EDGE_CURVE('',#17714,#17715,#7140,.T.);
#21501=EDGE_CURVE('',#17716,#17715,#7141,.T.);
#21502=EDGE_CURVE('',#17716,#17717,#16722,.T.);
#21503=EDGE_CURVE('',#17718,#17717,#7142,.T.);
#21504=EDGE_CURVE('',#17719,#17718,#16723,.T.);
#21505=EDGE_CURVE('',#17720,#17719,#7143,.T.);
#21506=EDGE_CURVE('',#17721,#17720,#7144,.T.);
#21507=EDGE_CURVE('',#17721,#17712,#7145,.T.);
#21508=EDGE_CURVE('',#17341,#17722,#7146,.T.);
#21509=EDGE_CURVE('',#17722,#17723,#16724,.T.);
#21510=EDGE_CURVE('',#17340,#17723,#7147,.T.);
#21511=EDGE_CURVE('',#17337,#17724,#7148,.T.);
#21512=EDGE_CURVE('',#17724,#17725,#16725,.T.);
#21513=EDGE_CURVE('',#17336,#17725,#7149,.T.);
#21514=EDGE_CURVE('',#17726,#17332,#7150,.T.);
#21515=EDGE_CURVE('',#17727,#17726,#16726,.T.);
#21516=EDGE_CURVE('',#17727,#17333,#7151,.T.);
#21517=EDGE_CURVE('',#17728,#17320,#7152,.T.);
#21518=EDGE_CURVE('',#17729,#17728,#16727,.T.);
#21519=EDGE_CURVE('',#17729,#17321,#7153,.T.);
#21520=EDGE_CURVE('',#17730,#17296,#7154,.T.);
#21521=EDGE_CURVE('',#17731,#17730,#16728,.T.);
#21522=EDGE_CURVE('',#17731,#17297,#7155,.T.);
#21523=EDGE_CURVE('',#17732,#17288,#7156,.T.);
#21524=EDGE_CURVE('',#17733,#17732,#16729,.T.);
#21525=EDGE_CURVE('',#17733,#17289,#7157,.T.);
#21526=EDGE_CURVE('',#17734,#17280,#7158,.T.);
#21527=EDGE_CURVE('',#17735,#17734,#16730,.T.);
#21528=EDGE_CURVE('',#17735,#17281,#7159,.T.);
#21529=EDGE_CURVE('',#17273,#17736,#7160,.T.);
#21530=EDGE_CURVE('',#17736,#17737,#16731,.T.);
#21531=EDGE_CURVE('',#17272,#17737,#7161,.T.);
#21532=EDGE_CURVE('',#17269,#17738,#7162,.T.);
#21533=EDGE_CURVE('',#17738,#17739,#16732,.T.);
#21534=EDGE_CURVE('',#17268,#17739,#7163,.T.);
#21535=EDGE_CURVE('',#17265,#17740,#7164,.T.);
#21536=EDGE_CURVE('',#17740,#17741,#16733,.T.);
#21537=EDGE_CURVE('',#17264,#17741,#7165,.T.);
#21538=EDGE_CURVE('',#17261,#17742,#7166,.T.);
#21539=EDGE_CURVE('',#17742,#17743,#16734,.T.);
#21540=EDGE_CURVE('',#17260,#17743,#7167,.T.);
#21541=EDGE_CURVE('',#17257,#17744,#7168,.T.);
#21542=EDGE_CURVE('',#17744,#17745,#16735,.T.);
#21543=EDGE_CURVE('',#17256,#17745,#7169,.T.);
#21544=EDGE_CURVE('',#17746,#17252,#7170,.T.);
#21545=EDGE_CURVE('',#17747,#17746,#16736,.T.);
#21546=EDGE_CURVE('',#17747,#17253,#7171,.T.);
#21547=EDGE_CURVE('',#17241,#17748,#7172,.T.);
#21548=EDGE_CURVE('',#17240,#17749,#7173,.T.);
#21549=EDGE_CURVE('',#17748,#17749,#16737,.T.);
#21550=EDGE_CURVE('',#17750,#17228,#7174,.T.);
#21551=EDGE_CURVE('',#17751,#17229,#7175,.T.);
#21552=EDGE_CURVE('',#17751,#17750,#16738,.T.);
#21553=EDGE_CURVE('',#17752,#17224,#7176,.T.);
#21554=EDGE_CURVE('',#17753,#17225,#7177,.T.);
#21555=EDGE_CURVE('',#17753,#17752,#16739,.T.);
#21556=EDGE_CURVE('',#17221,#17754,#7178,.T.);
#21557=EDGE_CURVE('',#17220,#17755,#7179,.T.);
#21558=EDGE_CURVE('',#17754,#17755,#16740,.T.);
#21559=EDGE_CURVE('',#17213,#17756,#7180,.T.);
#21560=EDGE_CURVE('',#17212,#17757,#7181,.T.);
#21561=EDGE_CURVE('',#17756,#17757,#16741,.T.);
#21562=EDGE_CURVE('',#17758,#17204,#7182,.T.);
#21563=EDGE_CURVE('',#17759,#17205,#7183,.T.);
#21564=EDGE_CURVE('',#17759,#17758,#16742,.T.);
#21565=EDGE_CURVE('',#17760,#17200,#7184,.T.);
#21566=EDGE_CURVE('',#17761,#17201,#7185,.T.);
#21567=EDGE_CURVE('',#17761,#17760,#16743,.T.);
#21568=EDGE_CURVE('',#17762,#17196,#7186,.T.);
#21569=EDGE_CURVE('',#17763,#17197,#7187,.T.);
#21570=EDGE_CURVE('',#17763,#17762,#16744,.T.);
#21571=EDGE_CURVE('',#17764,#17192,#7188,.T.);
#21572=EDGE_CURVE('',#17765,#17193,#7189,.T.);
#21573=EDGE_CURVE('',#17765,#17764,#16745,.T.);
#21574=EDGE_CURVE('',#17766,#17188,#7190,.T.);
#21575=EDGE_CURVE('',#17767,#17189,#7191,.T.);
#21576=EDGE_CURVE('',#17767,#17766,#16746,.T.);
#21577=EDGE_CURVE('',#17768,#17184,#7192,.T.);
#21578=EDGE_CURVE('',#17769,#17185,#7193,.T.);
#21579=EDGE_CURVE('',#17769,#17768,#16747,.T.);
#21580=EDGE_CURVE('',#17770,#17180,#7194,.T.);
#21581=EDGE_CURVE('',#17771,#17181,#7195,.T.);
#21582=EDGE_CURVE('',#17771,#17770,#16748,.T.);
#21583=EDGE_CURVE('',#17177,#17772,#7196,.T.);
#21584=EDGE_CURVE('',#17176,#17773,#7197,.T.);
#21585=EDGE_CURVE('',#17772,#17773,#16749,.T.);
#21586=EDGE_CURVE('',#17169,#17774,#7198,.T.);
#21587=EDGE_CURVE('',#17168,#17775,#7199,.T.);
#21588=EDGE_CURVE('',#17774,#17775,#16750,.T.);
#21589=EDGE_CURVE('',#17161,#17776,#7200,.T.);
#21590=EDGE_CURVE('',#17160,#17777,#7201,.T.);
#21591=EDGE_CURVE('',#17776,#17777,#16751,.T.);
#21592=EDGE_CURVE('',#17778,#17156,#7202,.T.);
#21593=EDGE_CURVE('',#17779,#17157,#7203,.T.);
#21594=EDGE_CURVE('',#17779,#17778,#16752,.T.);
#21595=EDGE_CURVE('',#17165,#17780,#7204,.T.);
#21596=EDGE_CURVE('',#17164,#17781,#7205,.T.);
#21597=EDGE_CURVE('',#17780,#17781,#16753,.T.);
#21598=EDGE_CURVE('',#17173,#17782,#7206,.T.);
#21599=EDGE_CURVE('',#17172,#17783,#7207,.T.);
#21600=EDGE_CURVE('',#17782,#17783,#16754,.T.);
#21601=EDGE_CURVE('',#17209,#17784,#7208,.T.);
#21602=EDGE_CURVE('',#17208,#17785,#7209,.T.);
#21603=EDGE_CURVE('',#17784,#17785,#16755,.T.);
#21604=EDGE_CURVE('',#17217,#17786,#7210,.T.);
#21605=EDGE_CURVE('',#17216,#17787,#7211,.T.);
#21606=EDGE_CURVE('',#17786,#17787,#16756,.T.);
#21607=EDGE_CURVE('',#17233,#17788,#7212,.T.);
#21608=EDGE_CURVE('',#17232,#17789,#7213,.T.);
#21609=EDGE_CURVE('',#17788,#17789,#16757,.T.);
#21610=EDGE_CURVE('',#17790,#17236,#7214,.T.);
#21611=EDGE_CURVE('',#17791,#17237,#7215,.T.);
#21612=EDGE_CURVE('',#17791,#17790,#16758,.T.);
#21613=EDGE_CURVE('',#17245,#17792,#7216,.T.);
#21614=EDGE_CURVE('',#17244,#17793,#7217,.T.);
#21615=EDGE_CURVE('',#17792,#17793,#16759,.T.);
#21616=EDGE_CURVE('',#17794,#17248,#7218,.T.);
#21617=EDGE_CURVE('',#17795,#17249,#7219,.T.);
#21618=EDGE_CURVE('',#17795,#17794,#16760,.T.);
#21619=EDGE_CURVE('',#17796,#17276,#7220,.T.);
#21620=EDGE_CURVE('',#17797,#17796,#16761,.T.);
#21621=EDGE_CURVE('',#17797,#17277,#7221,.T.);
#21622=EDGE_CURVE('',#17798,#17284,#7222,.T.);
#21623=EDGE_CURVE('',#17799,#17798,#16762,.T.);
#21624=EDGE_CURVE('',#17799,#17285,#7223,.T.);
#21625=EDGE_CURVE('',#17800,#17292,#7224,.T.);
#21626=EDGE_CURVE('',#17801,#17800,#16763,.T.);
#21627=EDGE_CURVE('',#17801,#17293,#7225,.T.);
#21628=EDGE_CURVE('',#17802,#17300,#7226,.T.);
#21629=EDGE_CURVE('',#17803,#17802,#16764,.T.);
#21630=EDGE_CURVE('',#17803,#17301,#7227,.T.);
#21631=EDGE_CURVE('',#17305,#17804,#7228,.T.);
#21632=EDGE_CURVE('',#17804,#17805,#16765,.T.);
#21633=EDGE_CURVE('',#17304,#17805,#7229,.T.);
#21634=EDGE_CURVE('',#17309,#17806,#7230,.T.);
#21635=EDGE_CURVE('',#17806,#17807,#16766,.T.);
#21636=EDGE_CURVE('',#17308,#17807,#7231,.T.);
#21637=EDGE_CURVE('',#17313,#17808,#7232,.T.);
#21638=EDGE_CURVE('',#17808,#17809,#16767,.T.);
#21639=EDGE_CURVE('',#17312,#17809,#7233,.T.);
#21640=EDGE_CURVE('',#17317,#17810,#7234,.T.);
#21641=EDGE_CURVE('',#17810,#17811,#16768,.T.);
#21642=EDGE_CURVE('',#17316,#17811,#7235,.T.);
#21643=EDGE_CURVE('',#17812,#17324,#7236,.T.);
#21644=EDGE_CURVE('',#17813,#17812,#16769,.T.);
#21645=EDGE_CURVE('',#17813,#17325,#7237,.T.);
#21646=EDGE_CURVE('',#17329,#17814,#7238,.T.);
#21647=EDGE_CURVE('',#17814,#17815,#16770,.T.);
#21648=EDGE_CURVE('',#17328,#17815,#7239,.T.);
#21649=EDGE_CURVE('',#17816,#17344,#7240,.T.);
#21650=EDGE_CURVE('',#17817,#17816,#16771,.T.);
#21651=EDGE_CURVE('',#17817,#17345,#7241,.T.);
#21652=EDGE_CURVE('',#17394,#17818,#7242,.T.);
#21653=EDGE_CURVE('',#17819,#17392,#7243,.T.);
#21654=EDGE_CURVE('',#17819,#17818,#7244,.T.);
#21655=EDGE_CURVE('',#17820,#17376,#7245,.T.);
#21656=EDGE_CURVE('',#17820,#17821,#7246,.T.);
#21657=EDGE_CURVE('',#17378,#17821,#7247,.T.);
#21658=EDGE_CURVE('',#17822,#17823,#7248,.T.);
#21659=EDGE_CURVE('',#17822,#17824,#7249,.T.);
#21660=EDGE_CURVE('',#17825,#17824,#7250,.T.);
#21661=EDGE_CURVE('',#17825,#17823,#7251,.T.);
#21662=EDGE_CURVE('',#17389,#17826,#7252,.T.);
#21663=EDGE_CURVE('',#17827,#17391,#7253,.T.);
#21664=EDGE_CURVE('',#17827,#17826,#7254,.T.);
#21665=EDGE_CURVE('',#17828,#17829,#7255,.T.);
#21666=EDGE_CURVE('',#17828,#17830,#7256,.T.);
#21667=EDGE_CURVE('',#17831,#17830,#7257,.T.);
#21668=EDGE_CURVE('',#17831,#17829,#7258,.T.);
#21669=EDGE_CURVE('',#17385,#17832,#7259,.T.);
#21670=EDGE_CURVE('',#17833,#17387,#7260,.T.);
#21671=EDGE_CURVE('',#17833,#17832,#7261,.T.);
#21672=EDGE_CURVE('',#17382,#17834,#7262,.T.);
#21673=EDGE_CURVE('',#17835,#17380,#7263,.T.);
#21674=EDGE_CURVE('',#17835,#17834,#7264,.T.);
#21675=EDGE_CURVE('',#17836,#17837,#7265,.T.);
#21676=EDGE_CURVE('',#17836,#17838,#7266,.T.);
#21677=EDGE_CURVE('',#17839,#17838,#7267,.T.);
#21678=EDGE_CURVE('',#17839,#17837,#7268,.T.);
#21679=EDGE_CURVE('',#17840,#17841,#7269,.T.);
#21680=EDGE_CURVE('',#17840,#17842,#7270,.T.);
#21681=EDGE_CURVE('',#17843,#17842,#7271,.T.);
#21682=EDGE_CURVE('',#17843,#17841,#7272,.T.);
#21683=EDGE_CURVE('',#17844,#17375,#7273,.T.);
#21684=EDGE_CURVE('',#17844,#17845,#7274,.T.);
#21685=EDGE_CURVE('',#17373,#17845,#7275,.T.);
#21686=EDGE_CURVE('',#17846,#17847,#7276,.T.);
#21687=EDGE_CURVE('',#17846,#17848,#7277,.T.);
#21688=EDGE_CURVE('',#17849,#17848,#7278,.T.);
#21689=EDGE_CURVE('',#17849,#17847,#7279,.T.);
#21690=EDGE_CURVE('',#17850,#17851,#7280,.T.);
#21691=EDGE_CURVE('',#17850,#17852,#7281,.T.);
#21692=EDGE_CURVE('',#17853,#17852,#7282,.T.);
#21693=EDGE_CURVE('',#17853,#17851,#7283,.T.);
#21694=EDGE_CURVE('',#17406,#17854,#7284,.T.);
#21695=EDGE_CURVE('',#17855,#17404,#7285,.T.);
#21696=EDGE_CURVE('',#17855,#17854,#7286,.T.);
#21697=EDGE_CURVE('',#17856,#17400,#7287,.T.);
#21698=EDGE_CURVE('',#17856,#17857,#7288,.T.);
#21699=EDGE_CURVE('',#17402,#17857,#7289,.T.);
#21700=EDGE_CURVE('',#17858,#17859,#7290,.T.);
#21701=EDGE_CURVE('',#17858,#17860,#7291,.T.);
#21702=EDGE_CURVE('',#17861,#17860,#7292,.T.);
#21703=EDGE_CURVE('',#17861,#17859,#7293,.T.);
#21704=EDGE_CURVE('',#17417,#17862,#7294,.T.);
#21705=EDGE_CURVE('',#17863,#17419,#7295,.T.);
#21706=EDGE_CURVE('',#17863,#17862,#7296,.T.);
#21707=EDGE_CURVE('',#17864,#17865,#7297,.T.);
#21708=EDGE_CURVE('',#17864,#17866,#7298,.T.);
#21709=EDGE_CURVE('',#17867,#17866,#7299,.T.);
#21710=EDGE_CURVE('',#17867,#17865,#7300,.T.);
#21711=EDGE_CURVE('',#17413,#17868,#7301,.T.);
#21712=EDGE_CURVE('',#17869,#17415,#7302,.T.);
#21713=EDGE_CURVE('',#17869,#17868,#7303,.T.);
#21714=EDGE_CURVE('',#17410,#17870,#7304,.T.);
#21715=EDGE_CURVE('',#17871,#17408,#7305,.T.);
#21716=EDGE_CURVE('',#17871,#17870,#7306,.T.);
#21717=EDGE_CURVE('',#17872,#17873,#7307,.T.);
#21718=EDGE_CURVE('',#17872,#17874,#7308,.T.);
#21719=EDGE_CURVE('',#17875,#17874,#7309,.T.);
#21720=EDGE_CURVE('',#17875,#17873,#7310,.T.);
#21721=EDGE_CURVE('',#17876,#17877,#7311,.T.);
#21722=EDGE_CURVE('',#17876,#17878,#7312,.T.);
#21723=EDGE_CURVE('',#17879,#17878,#7313,.T.);
#21724=EDGE_CURVE('',#17879,#17877,#7314,.T.);
#21725=EDGE_CURVE('',#17880,#17399,#7315,.T.);
#21726=EDGE_CURVE('',#17880,#17881,#7316,.T.);
#21727=EDGE_CURVE('',#17397,#17881,#7317,.T.);
#21728=EDGE_CURVE('',#17882,#17883,#7318,.T.);
#21729=EDGE_CURVE('',#17882,#17884,#7319,.T.);
#21730=EDGE_CURVE('',#17885,#17884,#7320,.T.);
#21731=EDGE_CURVE('',#17885,#17883,#7321,.T.);
#21732=EDGE_CURVE('',#17886,#17887,#7322,.T.);
#21733=EDGE_CURVE('',#17886,#17888,#7323,.T.);
#21734=EDGE_CURVE('',#17889,#17888,#7324,.T.);
#21735=EDGE_CURVE('',#17889,#17887,#7325,.T.);
#21736=EDGE_CURVE('',#17890,#17891,#2205,.T.);
#21737=EDGE_CURVE('',#17891,#17892,#7326,.T.);
#21738=EDGE_CURVE('',#17893,#17892,#2206,.T.);
#21739=EDGE_CURVE('',#17893,#17890,#7327,.T.);
#21740=EDGE_CURVE('',#17436,#17840,#16772,.T.);
#21741=EDGE_CURVE('',#17841,#17894,#16773,.T.);
#21742=EDGE_CURVE('',#17894,#17424,#2207,.T.);
#21743=EDGE_CURVE('',#17425,#17819,#16774,.T.);
#21744=EDGE_CURVE('',#17437,#17393,#2208,.T.);
#21745=EDGE_CURVE('',#17428,#17895,#16775,.T.);
#21746=EDGE_CURVE('',#17895,#17896,#7328,.T.);
#21747=EDGE_CURVE('',#17896,#17897,#16776,.T.);
#21748=EDGE_CURVE('',#17897,#17420,#2209,.T.);
#21749=EDGE_CURVE('',#17421,#17898,#16777,.T.);
#21750=EDGE_CURVE('',#17898,#17368,#7329,.T.);
#21751=EDGE_CURVE('',#17429,#17369,#2210,.T.);
#21752=EDGE_CURVE('',#17899,#17900,#7330,.T.);
#21753=EDGE_CURVE('',#17900,#17901,#16778,.T.);
#21754=EDGE_CURVE('',#17901,#17348,#2211,.T.);
#21755=EDGE_CURVE('',#17349,#17902,#7331,.T.);
#21756=EDGE_CURVE('',#17902,#17903,#16779,.T.);
#21757=EDGE_CURVE('',#17904,#17903,#2212,.T.);
#21758=EDGE_CURVE('',#17904,#17899,#16780,.T.);
#21759=EDGE_CURVE('',#17905,#17352,#7332,.T.);
#21760=EDGE_CURVE('',#17353,#17906,#2213,.T.);
#21761=EDGE_CURVE('',#17906,#17907,#16781,.T.);
#21762=EDGE_CURVE('',#17907,#17908,#7333,.T.);
#21763=EDGE_CURVE('',#17908,#17909,#16782,.T.);
#21764=EDGE_CURVE('',#17910,#17909,#2214,.T.);
#21765=EDGE_CURVE('',#17910,#17905,#16783,.T.);
#21766=EDGE_CURVE('',#17365,#17911,#7334,.T.);
#21767=EDGE_CURVE('',#17911,#17912,#16784,.T.);
#21768=EDGE_CURVE('',#17912,#17913,#2215,.T.);
#21769=EDGE_CURVE('',#17913,#17914,#16785,.T.);
#21770=EDGE_CURVE('',#17914,#17915,#7335,.T.);
#21771=EDGE_CURVE('',#17915,#17916,#16786,.T.);
#21772=EDGE_CURVE('',#17364,#17916,#2216,.T.);
#21773=EDGE_CURVE('',#17361,#17917,#7336,.T.);
#21774=EDGE_CURVE('',#17917,#17918,#16787,.T.);
#21775=EDGE_CURVE('',#17918,#17919,#2217,.T.);
#21776=EDGE_CURVE('',#17919,#17920,#16788,.T.);
#21777=EDGE_CURVE('',#17920,#17921,#7337,.T.);
#21778=EDGE_CURVE('',#17921,#17922,#16789,.T.);
#21779=EDGE_CURVE('',#17360,#17922,#2218,.T.);
#21780=EDGE_CURVE('',#17923,#17924,#7338,.T.);
#21781=EDGE_CURVE('',#17924,#17925,#16790,.T.);
#21782=EDGE_CURVE('',#17925,#17926,#2219,.T.);
#21783=EDGE_CURVE('',#17926,#17927,#16791,.T.);
#21784=EDGE_CURVE('',#17927,#17356,#7339,.T.);
#21785=EDGE_CURVE('',#17928,#17357,#2220,.T.);
#21786=EDGE_CURVE('',#17928,#17923,#16792,.T.);
#21787=EDGE_CURVE('',#17847,#17929,#16793,.T.);
#21788=EDGE_CURVE('',#17929,#17372,#2221,.T.);
#21789=EDGE_CURVE('',#17845,#17930,#16794,.T.);
#21790=EDGE_CURVE('',#17931,#17930,#2222,.T.);
#21791=EDGE_CURVE('',#17931,#17846,#16795,.T.);
#21792=EDGE_CURVE('',#17377,#17932,#2223,.T.);
#21793=EDGE_CURVE('',#17932,#17850,#16796,.T.);
#21794=EDGE_CURVE('',#17851,#17933,#16797,.T.);
#21795=EDGE_CURVE('',#17934,#17933,#2224,.T.);
#21796=EDGE_CURVE('',#17934,#17820,#16798,.T.);
#21797=EDGE_CURVE('',#17826,#17935,#16799,.T.);
#21798=EDGE_CURVE('',#17935,#17936,#2225,.T.);
#21799=EDGE_CURVE('',#17936,#17825,#16800,.T.);
#21800=EDGE_CURVE('',#17824,#17937,#16801,.T.);
#21801=EDGE_CURVE('',#17388,#17937,#2226,.T.);
#21802=EDGE_CURVE('',#17832,#17938,#16802,.T.);
#21803=EDGE_CURVE('',#17938,#17939,#2227,.T.);
#21804=EDGE_CURVE('',#17939,#17831,#16803,.T.);
#21805=EDGE_CURVE('',#17830,#17940,#16804,.T.);
#21806=EDGE_CURVE('',#17384,#17940,#2228,.T.);
#21807=EDGE_CURVE('',#17837,#17941,#16805,.T.);
#21808=EDGE_CURVE('',#17941,#17942,#2229,.T.);
#21809=EDGE_CURVE('',#17942,#17835,#16806,.T.);
#21810=EDGE_CURVE('',#17943,#17381,#2230,.T.);
#21811=EDGE_CURVE('',#17943,#17836,#16807,.T.);
#21812=EDGE_CURVE('',#17883,#17944,#16808,.T.);
#21813=EDGE_CURVE('',#17944,#17396,#2231,.T.);
#21814=EDGE_CURVE('',#17881,#17891,#16809,.T.);
#21815=EDGE_CURVE('',#17890,#17882,#16810,.T.);
#21816=EDGE_CURVE('',#17401,#17945,#2232,.T.);
#21817=EDGE_CURVE('',#17945,#17886,#16811,.T.);
#21818=EDGE_CURVE('',#17887,#17946,#16812,.T.);
#21819=EDGE_CURVE('',#17947,#17946,#2233,.T.);
#21820=EDGE_CURVE('',#17947,#17856,#16813,.T.);
#21821=EDGE_CURVE('',#17862,#17948,#16814,.T.);
#21822=EDGE_CURVE('',#17948,#17949,#2234,.T.);
#21823=EDGE_CURVE('',#17949,#17861,#16815,.T.);
#21824=EDGE_CURVE('',#17860,#17950,#16816,.T.);
#21825=EDGE_CURVE('',#17416,#17950,#2235,.T.);
#21826=EDGE_CURVE('',#17868,#17951,#16817,.T.);
#21827=EDGE_CURVE('',#17951,#17952,#2236,.T.);
#21828=EDGE_CURVE('',#17952,#17867,#16818,.T.);
#21829=EDGE_CURVE('',#17866,#17953,#16819,.T.);
#21830=EDGE_CURVE('',#17412,#17953,#2237,.T.);
#21831=EDGE_CURVE('',#17873,#17954,#16820,.T.);
#21832=EDGE_CURVE('',#17954,#17955,#2238,.T.);
#21833=EDGE_CURVE('',#17955,#17871,#16821,.T.);
#21834=EDGE_CURVE('',#17956,#17409,#2239,.T.);
#21835=EDGE_CURVE('',#17956,#17872,#16822,.T.);
#21836=EDGE_CURVE('',#17462,#17876,#16823,.T.);
#21837=EDGE_CURVE('',#17877,#17957,#16824,.T.);
#21838=EDGE_CURVE('',#17957,#17432,#2240,.T.);
#21839=EDGE_CURVE('',#17433,#17855,#16825,.T.);
#21840=EDGE_CURVE('',#17463,#17405,#2241,.T.);
#21841=EDGE_CURVE('',#17464,#17407,#2242,.T.);
#21842=EDGE_CURVE('',#17370,#17958,#7340,.T.);
#21843=EDGE_CURVE('',#17898,#17958,#7341,.T.);
#21844=EDGE_CURVE('',#17959,#17411,#2243,.T.);
#21845=EDGE_CURVE('',#17959,#17956,#7342,.T.);
#21846=EDGE_CURVE('',#17953,#17960,#7343,.T.);
#21847=EDGE_CURVE('',#17414,#17960,#2244,.T.);
#21848=EDGE_CURVE('',#17950,#17961,#7344,.T.);
#21849=EDGE_CURVE('',#17418,#17961,#2245,.T.);
#21850=EDGE_CURVE('',#17962,#17963,#7345,.T.);
#21851=EDGE_CURVE('',#17963,#17964,#7346,.T.);
#21852=EDGE_CURVE('',#17965,#17964,#7347,.T.);
#21853=EDGE_CURVE('',#17966,#17965,#7348,.T.);
#21854=EDGE_CURVE('',#17967,#17966,#16826,.T.);
#21855=EDGE_CURVE('',#17968,#17967,#7349,.T.);
#21856=EDGE_CURVE('',#17969,#17968,#16827,.T.);
#21857=EDGE_CURVE('',#17970,#17969,#7350,.T.);
#21858=EDGE_CURVE('',#17970,#17971,#7351,.T.);
#21859=EDGE_CURVE('',#17971,#17962,#7352,.T.);
#21860=EDGE_CURVE('',#17972,#17973,#7353,.T.);
#21861=EDGE_CURVE('',#17974,#17972,#7354,.T.);
#21862=EDGE_CURVE('',#17975,#17974,#7355,.T.);
#21863=EDGE_CURVE('',#17973,#17975,#7356,.T.);
#21864=EDGE_CURVE('',#17976,#17977,#16828,.T.);
#21865=EDGE_CURVE('',#17978,#17976,#7357,.T.);
#21866=EDGE_CURVE('',#17979,#17978,#16829,.T.);
#21867=EDGE_CURVE('',#17980,#17979,#7358,.T.);
#21868=EDGE_CURVE('',#17981,#17980,#16830,.T.);
#21869=EDGE_CURVE('',#17982,#17981,#7359,.T.);
#21870=EDGE_CURVE('',#17983,#17982,#16831,.T.);
#21871=EDGE_CURVE('',#17984,#17983,#7360,.T.);
#21872=EDGE_CURVE('',#17985,#17984,#16832,.T.);
#21873=EDGE_CURVE('',#17986,#17985,#7361,.T.);
#21874=EDGE_CURVE('',#17987,#17986,#16833,.T.);
#21875=EDGE_CURVE('',#17977,#17987,#7362,.T.);
#21876=EDGE_CURVE('',#17988,#17989,#7363,.T.);
#21877=EDGE_CURVE('',#17989,#17990,#7364,.T.);
#21878=EDGE_CURVE('',#17991,#17990,#7365,.T.);
#21879=EDGE_CURVE('',#17991,#17992,#7366,.T.);
#21880=EDGE_CURVE('',#17993,#17992,#7367,.T.);
#21881=EDGE_CURVE('',#17994,#17993,#7368,.T.);
#21882=EDGE_CURVE('',#17994,#17995,#16834,.T.);
#21883=EDGE_CURVE('',#17995,#17996,#7369,.T.);
#21884=EDGE_CURVE('',#17997,#17996,#16835,.T.);
#21885=EDGE_CURVE('',#17988,#17997,#7370,.T.);
#21886=EDGE_CURVE('',#17998,#17999,#7371,.T.);
#21887=EDGE_CURVE('',#17999,#18000,#7372,.T.);
#21888=EDGE_CURVE('',#18000,#18001,#7373,.T.);
#21889=EDGE_CURVE('',#18001,#17998,#7374,.T.);
#21890=EDGE_CURVE('',#18002,#18003,#7375,.T.);
#21891=EDGE_CURVE('',#18003,#18004,#16836,.T.);
#21892=EDGE_CURVE('',#18004,#18005,#7376,.T.);
#21893=EDGE_CURVE('',#18005,#18006,#16837,.T.);
#21894=EDGE_CURVE('',#18006,#18007,#7377,.T.);
#21895=EDGE_CURVE('',#18007,#18008,#16838,.T.);
#21896=EDGE_CURVE('',#18008,#18009,#7378,.T.);
#21897=EDGE_CURVE('',#18009,#18010,#16839,.T.);
#21898=EDGE_CURVE('',#18010,#18011,#7379,.T.);
#21899=EDGE_CURVE('',#18011,#18012,#16840,.T.);
#21900=EDGE_CURVE('',#18012,#18013,#7380,.T.);
#21901=EDGE_CURVE('',#18013,#18002,#16841,.T.);
#21902=EDGE_CURVE('',#17484,#18014,#7381,.T.);
#21903=EDGE_CURVE('',#17539,#17483,#7382,.T.);
#21904=EDGE_CURVE('',#18014,#17538,#7383,.T.);
#21905=EDGE_CURVE('',#17537,#18015,#7384,.T.);
#21906=EDGE_CURVE('',#17536,#17486,#7385,.T.);
#21907=EDGE_CURVE('',#18015,#17485,#7386,.T.);
#21908=EDGE_CURVE('',#17470,#18016,#7387,.T.);
#21909=EDGE_CURVE('',#17553,#17469,#7388,.T.);
#21910=EDGE_CURVE('',#18016,#17552,#7389,.T.);
#21911=EDGE_CURVE('',#17551,#18017,#7390,.T.);
#21912=EDGE_CURVE('',#17550,#17472,#7391,.T.);
#21913=EDGE_CURVE('',#18017,#17471,#7392,.T.);
#21914=EDGE_CURVE('',#17471,#17995,#2246,.T.);
#21915=EDGE_CURVE('',#17995,#18018,#7393,.T.);
#21916=EDGE_CURVE('',#18018,#17968,#7394,.T.);
#21917=EDGE_CURVE('',#17551,#17968,#2247,.T.);
#21918=EDGE_CURVE('',#17967,#18019,#7395,.T.);
#21919=EDGE_CURVE('',#18019,#17996,#7396,.T.);
#21920=EDGE_CURVE('',#17996,#17470,#2248,.T.);
#21921=EDGE_CURVE('',#17967,#17552,#2249,.T.);
#21922=EDGE_CURVE('',#17965,#17988,#7397,.T.);
#21923=EDGE_CURVE('',#17966,#17997,#7398,.T.);
#21924=EDGE_CURVE('',#17964,#17989,#7399,.T.);
#21925=EDGE_CURVE('',#17990,#17963,#7400,.T.);
#21926=EDGE_CURVE('',#17962,#17991,#7401,.T.);
#21927=EDGE_CURVE('',#17992,#17971,#7402,.T.);
#21928=EDGE_CURVE('',#17993,#17970,#7403,.T.);
#21929=EDGE_CURVE('',#17969,#17994,#7404,.T.);
#21930=EDGE_CURVE('',#17613,#18020,#7405,.T.);
#21931=EDGE_CURVE('',#18020,#17718,#7406,.T.);
#21932=EDGE_CURVE('',#17718,#17484,#2250,.T.);
#21933=EDGE_CURVE('',#17613,#17538,#2251,.T.);
#21934=EDGE_CURVE('',#17485,#17717,#2252,.T.);
#21935=EDGE_CURVE('',#17717,#18021,#7407,.T.);
#21936=EDGE_CURVE('',#18021,#17614,#7408,.T.);
#21937=EDGE_CURVE('',#17537,#17614,#2253,.T.);
#21938=EDGE_CURVE('',#17720,#17611,#7409,.T.);
#21939=EDGE_CURVE('',#17612,#17719,#7410,.T.);
#21940=EDGE_CURVE('',#17610,#17721,#7411,.T.);
#21941=EDGE_CURVE('',#17608,#17713,#7412,.T.);
#21942=EDGE_CURVE('',#17712,#17609,#7413,.T.);
#21943=EDGE_CURVE('',#17714,#17606,#7414,.T.);
#21944=EDGE_CURVE('',#17715,#17607,#7415,.T.);
#21945=EDGE_CURVE('',#17615,#17716,#7416,.T.);
#21946=EDGE_CURVE('',#17554,#17507,#16842,.T.);
#21947=EDGE_CURVE('',#17508,#17555,#16843,.T.);
#21948=EDGE_CURVE('',#17557,#17502,#16844,.T.);
#21949=EDGE_CURVE('',#17504,#17556,#16845,.T.);
#21950=EDGE_CURVE('',#17507,#18022,#16846,.T.);
#21951=EDGE_CURVE('',#18022,#18023,#7417,.T.);
#21952=EDGE_CURVE('',#18023,#17504,#16847,.T.);
#21953=EDGE_CURVE('',#17502,#18024,#16848,.T.);
#21954=EDGE_CURVE('',#18024,#18025,#7418,.T.);
#21955=EDGE_CURVE('',#18025,#17508,#16849,.T.);
#21956=EDGE_CURVE('',#18026,#17505,#16850,.T.);
#21957=EDGE_CURVE('',#18027,#18023,#7419,.T.);
#21958=EDGE_CURVE('',#18028,#18027,#16851,.T.);
#21959=EDGE_CURVE('',#18029,#18028,#7420,.T.);
#21960=EDGE_CURVE('',#18030,#18029,#16852,.T.);
#21961=EDGE_CURVE('',#18024,#18030,#7421,.T.);
#21962=EDGE_CURVE('',#17503,#18031,#16853,.T.);
#21963=EDGE_CURVE('',#18031,#18032,#7422,.T.);
#21964=EDGE_CURVE('',#18032,#18033,#16854,.T.);
#21965=EDGE_CURVE('',#18033,#18034,#7423,.T.);
#21966=EDGE_CURVE('',#18034,#18035,#16855,.T.);
#21967=EDGE_CURVE('',#18035,#18026,#7424,.T.);
#21968=EDGE_CURVE('',#18036,#17509,#16856,.T.);
#21969=EDGE_CURVE('',#18025,#18037,#7425,.T.);
#21970=EDGE_CURVE('',#18038,#18037,#16857,.T.);
#21971=EDGE_CURVE('',#18038,#18039,#7426,.T.);
#21972=EDGE_CURVE('',#18040,#18039,#16858,.T.);
#21973=EDGE_CURVE('',#18040,#18022,#7427,.T.);
#21974=EDGE_CURVE('',#17506,#18041,#16859,.T.);
#21975=EDGE_CURVE('',#18042,#18041,#7428,.T.);
#21976=EDGE_CURVE('',#18042,#18043,#16860,.T.);
#21977=EDGE_CURVE('',#18044,#18043,#7429,.T.);
#21978=EDGE_CURVE('',#18044,#18045,#16861,.T.);
#21979=EDGE_CURVE('',#18036,#18045,#7430,.T.);
#21980=EDGE_CURVE('',#18039,#18028,#7431,.T.);
#21981=EDGE_CURVE('',#18027,#18040,#7432,.T.);
#21982=EDGE_CURVE('',#18037,#18030,#7433,.T.);
#21983=EDGE_CURVE('',#18029,#18038,#7434,.T.);
#21984=EDGE_CURVE('',#18035,#18042,#7435,.T.);
#21985=EDGE_CURVE('',#18043,#18034,#7436,.T.);
#21986=EDGE_CURVE('',#18033,#18044,#7437,.T.);
#21987=EDGE_CURVE('',#18045,#18032,#7438,.T.);
#21988=EDGE_CURVE('',#18031,#18036,#7439,.T.);
#21989=EDGE_CURVE('',#18041,#18026,#7440,.T.);
#21990=EDGE_CURVE('',#17558,#17515,#16862,.T.);
#21991=EDGE_CURVE('',#17516,#17559,#16863,.T.);
#21992=EDGE_CURVE('',#17561,#17510,#16864,.T.);
#21993=EDGE_CURVE('',#17512,#17560,#16865,.T.);
#21994=EDGE_CURVE('',#17515,#18046,#16866,.T.);
#21995=EDGE_CURVE('',#18046,#18047,#7441,.T.);
#21996=EDGE_CURVE('',#18047,#17512,#16867,.T.);
#21997=EDGE_CURVE('',#17510,#18048,#16868,.T.);
#21998=EDGE_CURVE('',#18048,#18049,#7442,.T.);
#21999=EDGE_CURVE('',#18049,#17516,#16869,.T.);
#22000=EDGE_CURVE('',#18050,#17513,#16870,.T.);
#22001=EDGE_CURVE('',#18051,#18047,#7443,.T.);
#22002=EDGE_CURVE('',#18052,#18051,#16871,.T.);
#22003=EDGE_CURVE('',#18053,#18052,#7444,.T.);
#22004=EDGE_CURVE('',#18054,#18053,#16872,.T.);
#22005=EDGE_CURVE('',#18048,#18054,#7445,.T.);
#22006=EDGE_CURVE('',#17511,#18055,#16873,.T.);
#22007=EDGE_CURVE('',#18055,#18056,#7446,.T.);
#22008=EDGE_CURVE('',#18056,#18057,#16874,.T.);
#22009=EDGE_CURVE('',#18057,#18058,#7447,.T.);
#22010=EDGE_CURVE('',#18058,#18059,#16875,.T.);
#22011=EDGE_CURVE('',#18059,#18050,#7448,.T.);
#22012=EDGE_CURVE('',#18060,#17517,#16876,.T.);
#22013=EDGE_CURVE('',#18049,#18061,#7449,.T.);
#22014=EDGE_CURVE('',#18062,#18061,#16877,.T.);
#22015=EDGE_CURVE('',#18062,#18063,#7450,.T.);
#22016=EDGE_CURVE('',#18064,#18063,#16878,.T.);
#22017=EDGE_CURVE('',#18064,#18046,#7451,.T.);
#22018=EDGE_CURVE('',#17514,#18065,#16879,.T.);
#22019=EDGE_CURVE('',#18066,#18065,#7452,.T.);
#22020=EDGE_CURVE('',#18066,#18067,#16880,.T.);
#22021=EDGE_CURVE('',#18068,#18067,#7453,.T.);
#22022=EDGE_CURVE('',#18068,#18069,#16881,.T.);
#22023=EDGE_CURVE('',#18060,#18069,#7454,.T.);
#22024=EDGE_CURVE('',#18063,#18052,#7455,.T.);
#22025=EDGE_CURVE('',#18051,#18064,#7456,.T.);
#22026=EDGE_CURVE('',#18061,#18054,#7457,.T.);
#22027=EDGE_CURVE('',#18053,#18062,#7458,.T.);
#22028=EDGE_CURVE('',#18059,#18066,#7459,.T.);
#22029=EDGE_CURVE('',#18067,#18058,#7460,.T.);
#22030=EDGE_CURVE('',#18057,#18068,#7461,.T.);
#22031=EDGE_CURVE('',#18069,#18056,#7462,.T.);
#22032=EDGE_CURVE('',#18055,#18060,#7463,.T.);
#22033=EDGE_CURVE('',#18065,#18050,#7464,.T.);
#22034=EDGE_CURVE('',#17562,#17499,#16882,.T.);
#22035=EDGE_CURVE('',#17500,#17563,#16883,.T.);
#22036=EDGE_CURVE('',#17565,#17494,#16884,.T.);
#22037=EDGE_CURVE('',#17496,#17564,#16885,.T.);
#22038=EDGE_CURVE('',#17499,#18070,#16886,.T.);
#22039=EDGE_CURVE('',#18070,#18071,#7465,.T.);
#22040=EDGE_CURVE('',#18071,#17496,#16887,.T.);
#22041=EDGE_CURVE('',#17494,#18072,#16888,.T.);
#22042=EDGE_CURVE('',#18072,#18073,#7466,.T.);
#22043=EDGE_CURVE('',#18073,#17500,#16889,.T.);
#22044=EDGE_CURVE('',#18074,#17497,#16890,.T.);
#22045=EDGE_CURVE('',#18075,#18071,#7467,.T.);
#22046=EDGE_CURVE('',#18076,#18075,#16891,.T.);
#22047=EDGE_CURVE('',#18077,#18076,#7468,.T.);
#22048=EDGE_CURVE('',#18078,#18077,#16892,.T.);
#22049=EDGE_CURVE('',#18072,#18078,#7469,.T.);
#22050=EDGE_CURVE('',#17495,#18079,#16893,.T.);
#22051=EDGE_CURVE('',#18079,#18080,#7470,.T.);
#22052=EDGE_CURVE('',#18080,#18081,#16894,.T.);
#22053=EDGE_CURVE('',#18081,#18082,#7471,.T.);
#22054=EDGE_CURVE('',#18082,#18083,#16895,.T.);
#22055=EDGE_CURVE('',#18083,#18074,#7472,.T.);
#22056=EDGE_CURVE('',#18084,#17501,#16896,.T.);
#22057=EDGE_CURVE('',#18073,#18085,#7473,.T.);
#22058=EDGE_CURVE('',#18086,#18085,#16897,.T.);
#22059=EDGE_CURVE('',#18086,#18087,#7474,.T.);
#22060=EDGE_CURVE('',#18088,#18087,#16898,.T.);
#22061=EDGE_CURVE('',#18088,#18070,#7475,.T.);
#22062=EDGE_CURVE('',#17498,#18089,#16899,.T.);
#22063=EDGE_CURVE('',#18090,#18089,#7476,.T.);
#22064=EDGE_CURVE('',#18090,#18091,#16900,.T.);
#22065=EDGE_CURVE('',#18092,#18091,#7477,.T.);
#22066=EDGE_CURVE('',#18092,#18093,#16901,.T.);
#22067=EDGE_CURVE('',#18084,#18093,#7478,.T.);
#22068=EDGE_CURVE('',#18087,#18076,#7479,.T.);
#22069=EDGE_CURVE('',#18075,#18088,#7480,.T.);
#22070=EDGE_CURVE('',#18085,#18078,#7481,.T.);
#22071=EDGE_CURVE('',#18077,#18086,#7482,.T.);
#22072=EDGE_CURVE('',#18083,#18090,#7483,.T.);
#22073=EDGE_CURVE('',#18091,#18082,#7484,.T.);
#22074=EDGE_CURVE('',#18081,#18092,#7485,.T.);
#22075=EDGE_CURVE('',#18093,#18080,#7486,.T.);
#22076=EDGE_CURVE('',#18079,#18084,#7487,.T.);
#22077=EDGE_CURVE('',#18089,#18074,#7488,.T.);
#22078=EDGE_CURVE('',#17566,#17523,#16902,.T.);
#22079=EDGE_CURVE('',#17524,#17567,#16903,.T.);
#22080=EDGE_CURVE('',#17569,#17518,#16904,.T.);
#22081=EDGE_CURVE('',#17520,#17568,#16905,.T.);
#22082=EDGE_CURVE('',#17523,#18094,#16906,.T.);
#22083=EDGE_CURVE('',#18094,#18095,#7489,.T.);
#22084=EDGE_CURVE('',#18095,#17520,#16907,.T.);
#22085=EDGE_CURVE('',#17518,#18096,#16908,.T.);
#22086=EDGE_CURVE('',#18096,#18097,#7490,.T.);
#22087=EDGE_CURVE('',#18097,#17524,#16909,.T.);
#22088=EDGE_CURVE('',#18098,#17521,#16910,.T.);
#22089=EDGE_CURVE('',#18099,#18095,#7491,.T.);
#22090=EDGE_CURVE('',#18100,#18099,#16911,.T.);
#22091=EDGE_CURVE('',#18101,#18100,#7492,.T.);
#22092=EDGE_CURVE('',#18102,#18101,#16912,.T.);
#22093=EDGE_CURVE('',#18096,#18102,#7493,.T.);
#22094=EDGE_CURVE('',#17519,#18103,#16913,.T.);
#22095=EDGE_CURVE('',#18103,#18104,#7494,.T.);
#22096=EDGE_CURVE('',#18104,#18105,#16914,.T.);
#22097=EDGE_CURVE('',#18105,#18106,#7495,.T.);
#22098=EDGE_CURVE('',#18106,#18107,#16915,.T.);
#22099=EDGE_CURVE('',#18107,#18098,#7496,.T.);
#22100=EDGE_CURVE('',#18108,#17525,#16916,.T.);
#22101=EDGE_CURVE('',#18097,#18109,#7497,.T.);
#22102=EDGE_CURVE('',#18110,#18109,#16917,.T.);
#22103=EDGE_CURVE('',#18110,#18111,#7498,.T.);
#22104=EDGE_CURVE('',#18112,#18111,#16918,.T.);
#22105=EDGE_CURVE('',#18112,#18094,#7499,.T.);
#22106=EDGE_CURVE('',#17522,#18113,#16919,.T.);
#22107=EDGE_CURVE('',#18114,#18113,#7500,.T.);
#22108=EDGE_CURVE('',#18114,#18115,#16920,.T.);
#22109=EDGE_CURVE('',#18116,#18115,#7501,.T.);
#22110=EDGE_CURVE('',#18116,#18117,#16921,.T.);
#22111=EDGE_CURVE('',#18108,#18117,#7502,.T.);
#22112=EDGE_CURVE('',#18111,#18100,#7503,.T.);
#22113=EDGE_CURVE('',#18099,#18112,#7504,.T.);
#22114=EDGE_CURVE('',#18109,#18102,#7505,.T.);
#22115=EDGE_CURVE('',#18101,#18110,#7506,.T.);
#22116=EDGE_CURVE('',#18107,#18114,#7507,.T.);
#22117=EDGE_CURVE('',#18115,#18106,#7508,.T.);
#22118=EDGE_CURVE('',#18105,#18116,#7509,.T.);
#22119=EDGE_CURVE('',#18117,#18104,#7510,.T.);
#22120=EDGE_CURVE('',#18103,#18108,#7511,.T.);
#22121=EDGE_CURVE('',#18113,#18098,#7512,.T.);
#22122=EDGE_CURVE('',#17430,#17371,#2254,.T.);
#22123=EDGE_CURVE('',#17958,#17423,#16922,.T.);
#22124=EDGE_CURVE('',#17422,#18118,#2255,.T.);
#22125=EDGE_CURVE('',#18118,#18119,#16923,.T.);
#22126=EDGE_CURVE('',#18119,#18120,#7513,.T.);
#22127=EDGE_CURVE('',#18120,#17431,#16924,.T.);
#22128=EDGE_CURVE('',#18121,#18122,#2256,.T.);
#22129=EDGE_CURVE('',#18122,#18123,#16925,.T.);
#22130=EDGE_CURVE('',#18123,#17351,#7514,.T.);
#22131=EDGE_CURVE('',#17350,#18124,#2257,.T.);
#22132=EDGE_CURVE('',#18124,#18125,#16926,.T.);
#22133=EDGE_CURVE('',#18125,#18126,#7515,.T.);
#22134=EDGE_CURVE('',#18126,#18121,#16927,.T.);
#22135=EDGE_CURVE('',#18127,#18128,#2258,.T.);
#22136=EDGE_CURVE('',#18128,#18129,#16928,.T.);
#22137=EDGE_CURVE('',#18129,#18130,#7516,.T.);
#22138=EDGE_CURVE('',#18130,#18131,#16929,.T.);
#22139=EDGE_CURVE('',#18131,#17355,#2259,.T.);
#22140=EDGE_CURVE('',#17354,#18132,#7517,.T.);
#22141=EDGE_CURVE('',#18132,#18127,#16930,.T.);
#22142=EDGE_CURVE('',#17366,#18133,#2260,.T.);
#22143=EDGE_CURVE('',#18133,#18134,#16931,.T.);
#22144=EDGE_CURVE('',#18134,#18135,#7518,.T.);
#22145=EDGE_CURVE('',#18135,#18136,#16932,.T.);
#22146=EDGE_CURVE('',#18136,#18137,#2261,.T.);
#22147=EDGE_CURVE('',#18137,#18138,#16933,.T.);
#22148=EDGE_CURVE('',#18138,#17367,#7519,.T.);
#22149=EDGE_CURVE('',#17362,#18139,#2262,.T.);
#22150=EDGE_CURVE('',#18139,#18140,#16934,.T.);
#22151=EDGE_CURVE('',#18140,#18141,#7520,.T.);
#22152=EDGE_CURVE('',#18141,#18142,#16935,.T.);
#22153=EDGE_CURVE('',#18142,#18143,#2263,.T.);
#22154=EDGE_CURVE('',#18143,#18144,#16936,.T.);
#22155=EDGE_CURVE('',#18144,#17363,#7521,.T.);
#22156=EDGE_CURVE('',#18145,#17359,#2264,.T.);
#22157=EDGE_CURVE('',#17358,#18146,#7522,.T.);
#22158=EDGE_CURVE('',#18146,#18147,#16937,.T.);
#22159=EDGE_CURVE('',#18147,#18148,#2265,.T.);
#22160=EDGE_CURVE('',#18148,#18149,#16938,.T.);
#22161=EDGE_CURVE('',#18149,#18150,#7523,.T.);
#22162=EDGE_CURVE('',#18150,#18145,#16939,.T.);
#22163=EDGE_CURVE('',#17438,#17395,#2266,.T.);
#22164=EDGE_CURVE('',#17818,#17427,#16940,.T.);
#22165=EDGE_CURVE('',#17426,#18151,#2267,.T.);
#22166=EDGE_CURVE('',#18151,#17843,#16941,.T.);
#22167=EDGE_CURVE('',#17842,#17439,#16942,.T.);
#22168=EDGE_CURVE('',#18152,#18153,#2268,.T.);
#22169=EDGE_CURVE('',#18153,#17844,#16943,.T.);
#22170=EDGE_CURVE('',#17374,#18154,#2269,.T.);
#22171=EDGE_CURVE('',#18154,#17849,#16944,.T.);
#22172=EDGE_CURVE('',#17848,#18152,#16945,.T.);
#22173=EDGE_CURVE('',#18155,#18156,#2270,.T.);
#22174=EDGE_CURVE('',#18156,#17853,#16946,.T.);
#22175=EDGE_CURVE('',#17852,#18157,#16947,.T.);
#22176=EDGE_CURVE('',#18157,#17379,#2271,.T.);
#22177=EDGE_CURVE('',#17821,#18155,#16948,.T.);
#22178=EDGE_CURVE('',#17390,#18158,#2272,.T.);
#22179=EDGE_CURVE('',#18158,#17822,#16949,.T.);
#22180=EDGE_CURVE('',#17823,#18159,#16950,.T.);
#22181=EDGE_CURVE('',#18159,#18160,#2273,.T.);
#22182=EDGE_CURVE('',#18160,#17827,#16951,.T.);
#22183=EDGE_CURVE('',#17386,#18161,#2274,.T.);
#22184=EDGE_CURVE('',#18161,#17828,#16952,.T.);
#22185=EDGE_CURVE('',#17829,#18162,#16953,.T.);
#22186=EDGE_CURVE('',#18162,#18163,#2275,.T.);
#22187=EDGE_CURVE('',#18163,#17833,#16954,.T.);
#22188=EDGE_CURVE('',#18164,#17383,#2276,.T.);
#22189=EDGE_CURVE('',#17834,#18165,#16955,.T.);
#22190=EDGE_CURVE('',#18165,#18166,#2277,.T.);
#22191=EDGE_CURVE('',#18166,#17839,#16956,.T.);
#22192=EDGE_CURVE('',#17838,#18164,#16957,.T.);
#22193=EDGE_CURVE('',#17854,#17435,#16958,.T.);
#22194=EDGE_CURVE('',#17434,#18167,#2278,.T.);
#22195=EDGE_CURVE('',#18167,#17879,#16959,.T.);
#22196=EDGE_CURVE('',#17878,#17465,#16960,.T.);
#22197=EDGE_CURVE('',#17892,#17880,#16961,.T.);
#22198=EDGE_CURVE('',#17398,#18168,#2279,.T.);
#22199=EDGE_CURVE('',#18168,#17885,#16962,.T.);
#22200=EDGE_CURVE('',#17884,#17893,#16963,.T.);
#22201=EDGE_CURVE('',#18169,#18170,#2280,.T.);
#22202=EDGE_CURVE('',#18170,#17889,#16964,.T.);
#22203=EDGE_CURVE('',#17888,#18171,#16965,.T.);
#22204=EDGE_CURVE('',#18171,#17403,#2281,.T.);
#22205=EDGE_CURVE('',#17857,#18169,#16966,.T.);
#22206=EDGE_CURVE('',#17961,#17858,#16967,.T.);
#22207=EDGE_CURVE('',#17859,#18172,#16968,.T.);
#22208=EDGE_CURVE('',#18172,#18173,#2282,.T.);
#22209=EDGE_CURVE('',#18173,#17863,#16969,.T.);
#22210=EDGE_CURVE('',#17960,#17864,#16970,.T.);
#22211=EDGE_CURVE('',#17865,#18174,#16971,.T.);
#22212=EDGE_CURVE('',#18174,#18175,#2283,.T.);
#22213=EDGE_CURVE('',#18175,#17869,#16972,.T.);
#22214=EDGE_CURVE('',#17870,#18176,#16973,.T.);
#22215=EDGE_CURVE('',#18176,#18177,#2284,.T.);
#22216=EDGE_CURVE('',#18177,#17875,#16974,.T.);
#22217=EDGE_CURVE('',#17874,#17959,#16975,.T.);
#22218=EDGE_CURVE('',#18169,#17947,#7524,.T.);
#22219=EDGE_CURVE('',#17946,#18170,#7525,.T.);
#22220=EDGE_CURVE('',#17905,#18132,#7526,.T.);
#22221=EDGE_CURVE('',#18134,#17915,#7527,.T.);
#22222=EDGE_CURVE('',#17914,#18135,#7528,.T.);
#22223=EDGE_CURVE('',#18138,#17911,#7529,.T.);
#22224=EDGE_CURVE('',#18140,#17921,#7530,.T.);
#22225=EDGE_CURVE('',#17920,#18141,#7531,.T.);
#22226=EDGE_CURVE('',#18144,#17917,#7532,.T.);
#22227=EDGE_CURVE('',#17927,#18146,#7533,.T.);
#22228=EDGE_CURVE('',#17923,#18150,#7534,.T.);
#22229=EDGE_CURVE('',#18149,#17924,#7535,.T.);
#22230=EDGE_CURVE('',#17895,#18120,#7536,.T.);
#22231=EDGE_CURVE('',#18119,#17896,#7537,.T.);
#22232=EDGE_CURVE('',#18123,#17902,#7538,.T.);
#22233=EDGE_CURVE('',#17899,#18126,#7539,.T.);
#22234=EDGE_CURVE('',#18125,#17900,#7540,.T.);
#22235=EDGE_CURVE('',#17907,#18130,#7541,.T.);
#22236=EDGE_CURVE('',#18129,#17908,#7542,.T.);
#22237=EDGE_CURVE('',#17933,#18156,#7543,.T.);
#22238=EDGE_CURVE('',#18155,#17934,#7544,.T.);
#22239=EDGE_CURVE('',#18171,#17945,#7545,.T.);
#22240=EDGE_CURVE('',#17930,#18153,#7546,.T.);
#22241=EDGE_CURVE('',#18152,#17931,#7547,.T.);
#22242=EDGE_CURVE('',#17944,#18168,#7548,.T.);
#22243=EDGE_CURVE('',#17957,#18167,#7549,.T.);
#22244=EDGE_CURVE('',#18164,#17943,#7550,.T.);
#22245=EDGE_CURVE('',#18176,#17955,#7551,.T.);
#22246=EDGE_CURVE('',#17954,#18177,#7552,.T.);
#22247=EDGE_CURVE('',#17940,#18161,#7553,.T.);
#22248=EDGE_CURVE('',#18174,#17952,#7554,.T.);
#22249=EDGE_CURVE('',#17951,#18175,#7555,.T.);
#22250=EDGE_CURVE('',#18172,#17949,#7556,.T.);
#22251=EDGE_CURVE('',#17948,#18173,#7557,.T.);
#22252=EDGE_CURVE('',#17937,#18158,#7558,.T.);
#22253=EDGE_CURVE('',#17909,#18128,#7559,.T.);
#22254=EDGE_CURVE('',#18127,#17910,#7560,.T.);
#22255=EDGE_CURVE('',#18157,#17932,#7561,.T.);
#22256=EDGE_CURVE('',#17903,#18122,#7562,.T.);
#22257=EDGE_CURVE('',#18121,#17904,#7563,.T.);
#22258=EDGE_CURVE('',#17929,#18154,#7564,.T.);
#22259=EDGE_CURVE('',#17894,#18151,#7565,.T.);
#22260=EDGE_CURVE('',#18145,#17928,#7566,.T.);
#22261=EDGE_CURVE('',#18165,#17942,#7567,.T.);
#22262=EDGE_CURVE('',#17941,#18166,#7568,.T.);
#22263=EDGE_CURVE('',#17922,#18139,#7569,.T.);
#22264=EDGE_CURVE('',#18162,#17939,#7570,.T.);
#22265=EDGE_CURVE('',#17938,#18163,#7571,.T.);
#22266=EDGE_CURVE('',#18159,#17936,#7572,.T.);
#22267=EDGE_CURVE('',#17935,#18160,#7573,.T.);
#22268=EDGE_CURVE('',#17916,#18133,#7574,.T.);
#22269=EDGE_CURVE('',#18131,#17906,#7575,.T.);
#22270=EDGE_CURVE('',#17901,#18124,#7576,.T.);
#22271=EDGE_CURVE('',#17897,#18118,#7577,.T.);
#22272=EDGE_CURVE('',#18147,#17926,#7578,.T.);
#22273=EDGE_CURVE('',#17925,#18148,#7579,.T.);
#22274=EDGE_CURVE('',#18142,#17919,#7580,.T.);
#22275=EDGE_CURVE('',#17918,#18143,#7581,.T.);
#22276=EDGE_CURVE('',#18136,#17913,#7582,.T.);
#22277=EDGE_CURVE('',#17912,#18137,#7583,.T.);
#22278=EDGE_CURVE('',#18003,#17976,#7584,.T.);
#22279=EDGE_CURVE('',#18004,#17977,#7585,.T.);
#22280=EDGE_CURVE('',#18002,#17978,#7586,.T.);
#22281=EDGE_CURVE('',#18013,#17979,#7587,.T.);
#22282=EDGE_CURVE('',#18012,#17980,#7588,.T.);
#22283=EDGE_CURVE('',#18011,#17981,#7589,.T.);
#22284=EDGE_CURVE('',#18010,#17982,#7590,.T.);
#22285=EDGE_CURVE('',#18009,#17983,#7591,.T.);
#22286=EDGE_CURVE('',#18008,#17984,#7592,.T.);
#22287=EDGE_CURVE('',#18007,#17985,#7593,.T.);
#22288=EDGE_CURVE('',#18006,#17986,#7594,.T.);
#22289=EDGE_CURVE('',#18005,#17987,#7595,.T.);
#22290=EDGE_CURVE('',#17999,#17972,#7596,.T.);
#22291=EDGE_CURVE('',#18000,#17973,#7597,.T.);
#22292=EDGE_CURVE('',#17998,#17974,#7598,.T.);
#22293=EDGE_CURVE('',#18001,#17975,#7599,.T.);
#22294=EDGE_CURVE('',#17817,#17617,#7600,.T.);
#22295=EDGE_CURVE('',#17816,#17616,#7601,.T.);
#22296=EDGE_CURVE('',#17722,#17710,#7602,.T.);
#22297=EDGE_CURVE('',#17723,#17711,#7603,.T.);
#22298=EDGE_CURVE('',#17724,#17708,#7604,.T.);
#22299=EDGE_CURVE('',#17725,#17709,#7605,.T.);
#22300=EDGE_CURVE('',#17727,#17619,#7606,.T.);
#22301=EDGE_CURVE('',#17726,#17618,#7607,.T.);
#22302=EDGE_CURVE('',#17814,#17706,#7608,.T.);
#22303=EDGE_CURVE('',#17815,#17707,#7609,.T.);
#22304=EDGE_CURVE('',#17813,#17621,#7610,.T.);
#22305=EDGE_CURVE('',#17812,#17620,#7611,.T.);
#22306=EDGE_CURVE('',#17729,#17623,#7612,.T.);
#22307=EDGE_CURVE('',#17728,#17622,#7613,.T.);
#22308=EDGE_CURVE('',#17810,#17704,#7614,.T.);
#22309=EDGE_CURVE('',#17811,#17705,#7615,.T.);
#22310=EDGE_CURVE('',#17808,#17702,#7616,.T.);
#22311=EDGE_CURVE('',#17809,#17703,#7617,.T.);
#22312=EDGE_CURVE('',#17806,#17700,#7618,.T.);
#22313=EDGE_CURVE('',#17807,#17701,#7619,.T.);
#22314=EDGE_CURVE('',#17804,#17698,#7620,.T.);
#22315=EDGE_CURVE('',#17805,#17699,#7621,.T.);
#22316=EDGE_CURVE('',#17803,#17625,#7622,.T.);
#22317=EDGE_CURVE('',#17802,#17624,#7623,.T.);
#22318=EDGE_CURVE('',#17731,#17627,#7624,.T.);
#22319=EDGE_CURVE('',#17730,#17626,#7625,.T.);
#22320=EDGE_CURVE('',#17801,#17629,#7626,.T.);
#22321=EDGE_CURVE('',#17800,#17628,#7627,.T.);
#22322=EDGE_CURVE('',#17733,#17631,#7628,.T.);
#22323=EDGE_CURVE('',#17732,#17630,#7629,.T.);
#22324=EDGE_CURVE('',#17799,#17633,#7630,.T.);
#22325=EDGE_CURVE('',#17798,#17632,#7631,.T.);
#22326=EDGE_CURVE('',#17735,#17635,#7632,.T.);
#22327=EDGE_CURVE('',#17734,#17634,#7633,.T.);
#22328=EDGE_CURVE('',#17797,#17637,#7634,.T.);
#22329=EDGE_CURVE('',#17796,#17636,#7635,.T.);
#22330=EDGE_CURVE('',#17736,#17696,#7636,.T.);
#22331=EDGE_CURVE('',#17737,#17697,#7637,.T.);
#22332=EDGE_CURVE('',#17738,#17694,#7638,.T.);
#22333=EDGE_CURVE('',#17739,#17695,#7639,.T.);
#22334=EDGE_CURVE('',#17740,#17692,#7640,.T.);
#22335=EDGE_CURVE('',#17741,#17693,#7641,.T.);
#22336=EDGE_CURVE('',#17742,#17690,#7642,.T.);
#22337=EDGE_CURVE('',#17743,#17691,#7643,.T.);
#22338=EDGE_CURVE('',#17744,#17688,#7644,.T.);
#22339=EDGE_CURVE('',#17745,#17689,#7645,.T.);
#22340=EDGE_CURVE('',#17747,#17639,#7646,.T.);
#22341=EDGE_CURVE('',#17746,#17638,#7647,.T.);
#22342=EDGE_CURVE('',#17794,#17686,#7648,.T.);
#22343=EDGE_CURVE('',#17795,#17687,#7649,.T.);
#22344=EDGE_CURVE('',#17792,#17640,#7650,.T.);
#22345=EDGE_CURVE('',#17793,#17641,#7651,.T.);
#22346=EDGE_CURVE('',#17748,#17642,#7652,.T.);
#22347=EDGE_CURVE('',#17749,#17643,#7653,.T.);
#22348=EDGE_CURVE('',#17790,#17684,#7654,.T.);
#22349=EDGE_CURVE('',#17791,#17685,#7655,.T.);
#22350=EDGE_CURVE('',#17788,#17644,#7656,.T.);
#22351=EDGE_CURVE('',#17789,#17645,#7657,.T.);
#22352=EDGE_CURVE('',#17750,#17682,#7658,.T.);
#22353=EDGE_CURVE('',#17751,#17683,#7659,.T.);
#22354=EDGE_CURVE('',#17752,#17680,#7660,.T.);
#22355=EDGE_CURVE('',#17753,#17681,#7661,.T.);
#22356=EDGE_CURVE('',#17754,#17646,#7662,.T.);
#22357=EDGE_CURVE('',#17755,#17647,#7663,.T.);
#22358=EDGE_CURVE('',#17786,#17648,#7664,.T.);
#22359=EDGE_CURVE('',#17787,#17649,#7665,.T.);
#22360=EDGE_CURVE('',#17756,#17650,#7666,.T.);
#22361=EDGE_CURVE('',#17757,#17651,#7667,.T.);
#22362=EDGE_CURVE('',#17784,#17652,#7668,.T.);
#22363=EDGE_CURVE('',#17785,#17653,#7669,.T.);
#22364=EDGE_CURVE('',#17758,#17678,#7670,.T.);
#22365=EDGE_CURVE('',#17759,#17679,#7671,.T.);
#22366=EDGE_CURVE('',#17760,#17676,#7672,.T.);
#22367=EDGE_CURVE('',#17761,#17677,#7673,.T.);
#22368=EDGE_CURVE('',#17762,#17674,#7674,.T.);
#22369=EDGE_CURVE('',#17763,#17675,#7675,.T.);
#22370=EDGE_CURVE('',#17764,#17672,#7676,.T.);
#22371=EDGE_CURVE('',#17765,#17673,#7677,.T.);
#22372=EDGE_CURVE('',#17766,#17670,#7678,.T.);
#22373=EDGE_CURVE('',#17767,#17671,#7679,.T.);
#22374=EDGE_CURVE('',#17768,#17668,#7680,.T.);
#22375=EDGE_CURVE('',#17769,#17669,#7681,.T.);
#22376=EDGE_CURVE('',#17770,#17666,#7682,.T.);
#22377=EDGE_CURVE('',#17771,#17667,#7683,.T.);
#22378=EDGE_CURVE('',#17772,#17654,#7684,.T.);
#22379=EDGE_CURVE('',#17773,#17655,#7685,.T.);
#22380=EDGE_CURVE('',#17782,#17656,#7686,.T.);
#22381=EDGE_CURVE('',#17783,#17657,#7687,.T.);
#22382=EDGE_CURVE('',#17774,#17658,#7688,.T.);
#22383=EDGE_CURVE('',#17775,#17659,#7689,.T.);
#22384=EDGE_CURVE('',#17780,#17660,#7690,.T.);
#22385=EDGE_CURVE('',#17781,#17661,#7691,.T.);
#22386=EDGE_CURVE('',#17776,#17662,#7692,.T.);
#22387=EDGE_CURVE('',#17777,#17663,#7693,.T.);
#22388=EDGE_CURVE('',#17778,#17664,#7694,.T.);
#22389=EDGE_CURVE('',#17779,#17665,#7695,.T.);
#22390=EDGE_CURVE('',#17480,#17542,#7696,.T.);
#22391=EDGE_CURVE('',#17479,#17543,#7697,.T.);
#22392=EDGE_CURVE('',#17478,#17544,#7698,.T.);
#22393=EDGE_CURVE('',#17477,#17545,#7699,.T.);
#22394=EDGE_CURVE('',#17476,#17546,#7700,.T.);
#22395=EDGE_CURVE('',#17475,#17547,#7701,.T.);
#22396=EDGE_CURVE('',#17572,#17593,#7702,.T.);
#22397=EDGE_CURVE('',#17477,#17572,#16976,.T.);
#22398=EDGE_CURVE('',#17545,#17593,#16977,.T.);
#22399=EDGE_CURVE('',#17570,#17478,#16978,.T.);
#22400=EDGE_CURVE('',#17570,#17592,#7703,.T.);
#22401=EDGE_CURVE('',#17592,#17544,#16979,.T.);
#22402=EDGE_CURVE('',#17594,#17571,#7704,.T.);
#22403=EDGE_CURVE('',#17597,#17573,#7705,.T.);
#22404=EDGE_CURVE('',#17595,#17575,#7706,.T.);
#22405=EDGE_CURVE('',#17596,#17574,#7707,.T.);
#22406=EDGE_CURVE('',#17598,#17582,#16980,.T.);
#22407=EDGE_CURVE('',#17583,#17599,#16981,.T.);
#22408=EDGE_CURVE('',#17601,#17578,#16982,.T.);
#22409=EDGE_CURVE('',#17579,#17600,#16983,.T.);
#22410=EDGE_CURVE('',#17582,#18178,#16984,.T.);
#22411=EDGE_CURVE('',#18178,#18179,#7708,.T.);
#22412=EDGE_CURVE('',#18179,#17579,#16985,.T.);
#22413=EDGE_CURVE('',#17578,#18180,#16986,.T.);
#22414=EDGE_CURVE('',#18180,#18181,#7709,.T.);
#22415=EDGE_CURVE('',#18181,#17583,#16987,.T.);
#22416=EDGE_CURVE('',#17577,#18182,#16988,.T.);
#22417=EDGE_CURVE('',#18182,#18183,#7710,.T.);
#22418=EDGE_CURVE('',#18183,#18184,#16989,.T.);
#22419=EDGE_CURVE('',#18184,#18185,#7711,.T.);
#22420=EDGE_CURVE('',#18185,#18186,#16990,.T.);
#22421=EDGE_CURVE('',#18186,#18187,#7712,.T.);
#22422=EDGE_CURVE('',#18187,#17580,#16991,.T.);
#22423=EDGE_CURVE('',#18188,#18179,#7713,.T.);
#22424=EDGE_CURVE('',#18189,#18188,#16992,.T.);
#22425=EDGE_CURVE('',#18190,#18189,#7714,.T.);
#22426=EDGE_CURVE('',#18191,#18190,#16993,.T.);
#22427=EDGE_CURVE('',#18180,#18191,#7715,.T.);
#22428=EDGE_CURVE('',#17581,#18192,#16994,.T.);
#22429=EDGE_CURVE('',#18193,#18192,#7716,.T.);
#22430=EDGE_CURVE('',#18193,#18194,#16995,.T.);
#22431=EDGE_CURVE('',#18195,#18194,#7717,.T.);
#22432=EDGE_CURVE('',#18195,#18196,#16996,.T.);
#22433=EDGE_CURVE('',#18197,#18196,#7718,.T.);
#22434=EDGE_CURVE('',#18197,#17576,#16997,.T.);
#22435=EDGE_CURVE('',#18181,#18198,#7719,.T.);
#22436=EDGE_CURVE('',#18199,#18198,#16998,.T.);
#22437=EDGE_CURVE('',#18199,#18200,#7720,.T.);
#22438=EDGE_CURVE('',#18201,#18200,#16999,.T.);
#22439=EDGE_CURVE('',#18201,#18178,#7721,.T.);
#22440=EDGE_CURVE('',#18200,#18189,#7722,.T.);
#22441=EDGE_CURVE('',#18188,#18201,#7723,.T.);
#22442=EDGE_CURVE('',#18198,#18191,#7724,.T.);
#22443=EDGE_CURVE('',#18190,#18199,#7725,.T.);
#22444=EDGE_CURVE('',#18186,#18193,#7726,.T.);
#22445=EDGE_CURVE('',#18194,#18185,#7727,.T.);
#22446=EDGE_CURVE('',#18184,#18195,#7728,.T.);
#22447=EDGE_CURVE('',#18196,#18183,#7729,.T.);
#22448=EDGE_CURVE('',#18182,#18197,#7730,.T.);
#22449=EDGE_CURVE('',#18192,#18187,#7731,.T.);
#22450=EDGE_CURVE('',#17590,#17604,#17000,.T.);
#22451=EDGE_CURVE('',#17603,#17591,#17001,.T.);
#22452=EDGE_CURVE('',#17586,#17602,#17002,.T.);
#22453=EDGE_CURVE('',#17605,#17587,#17003,.T.);
#22454=EDGE_CURVE('',#18202,#17586,#17004,.T.);
#22455=EDGE_CURVE('',#18203,#18202,#7732,.T.);
#22456=EDGE_CURVE('',#17591,#18203,#17005,.T.);
#22457=EDGE_CURVE('',#18204,#17590,#17006,.T.);
#22458=EDGE_CURVE('',#18205,#18204,#7733,.T.);
#22459=EDGE_CURVE('',#17587,#18205,#17007,.T.);
#22460=EDGE_CURVE('',#18206,#17584,#17008,.T.);
#22461=EDGE_CURVE('',#18207,#18206,#7734,.T.);
#22462=EDGE_CURVE('',#18208,#18207,#17009,.T.);
#22463=EDGE_CURVE('',#18209,#18208,#7735,.T.);
#22464=EDGE_CURVE('',#18210,#18209,#17010,.T.);
#22465=EDGE_CURVE('',#18211,#18210,#7736,.T.);
#22466=EDGE_CURVE('',#17588,#18211,#17011,.T.);
#22467=EDGE_CURVE('',#18205,#18212,#7737,.T.);
#22468=EDGE_CURVE('',#18212,#18213,#17012,.T.);
#22469=EDGE_CURVE('',#18213,#18214,#7738,.T.);
#22470=EDGE_CURVE('',#18214,#18215,#17013,.T.);
#22471=EDGE_CURVE('',#18215,#18202,#7739,.T.);
#22472=EDGE_CURVE('',#18216,#17589,#17014,.T.);
#22473=EDGE_CURVE('',#18216,#18217,#7740,.T.);
#22474=EDGE_CURVE('',#18218,#18217,#17015,.T.);
#22475=EDGE_CURVE('',#18218,#18219,#7741,.T.);
#22476=EDGE_CURVE('',#18220,#18219,#17016,.T.);
#22477=EDGE_CURVE('',#18220,#18221,#7742,.T.);
#22478=EDGE_CURVE('',#17585,#18221,#17017,.T.);
#22479=EDGE_CURVE('',#18222,#18203,#7743,.T.);
#22480=EDGE_CURVE('',#18222,#18223,#17018,.T.);
#22481=EDGE_CURVE('',#18224,#18223,#7744,.T.);
#22482=EDGE_CURVE('',#18224,#18225,#17019,.T.);
#22483=EDGE_CURVE('',#18204,#18225,#7745,.T.);
#22484=EDGE_CURVE('',#18215,#18222,#7746,.T.);
#22485=EDGE_CURVE('',#18223,#18214,#7747,.T.);
#22486=EDGE_CURVE('',#18213,#18224,#7748,.T.);
#22487=EDGE_CURVE('',#18225,#18212,#7749,.T.);
#22488=EDGE_CURVE('',#18219,#18208,#7750,.T.);
#22489=EDGE_CURVE('',#18207,#18220,#7751,.T.);
#22490=EDGE_CURVE('',#18217,#18210,#7752,.T.);
#22491=EDGE_CURVE('',#18209,#18218,#7753,.T.);
#22492=EDGE_CURVE('',#18211,#18216,#7754,.T.);
#22493=EDGE_CURVE('',#18221,#18206,#7755,.T.);
#22494=EDGE_CURVE('',#17467,#17528,#7756,.T.);
#22495=EDGE_CURVE('',#17493,#17529,#7757,.T.);
#22496=EDGE_CURVE('',#17492,#17530,#7758,.T.);
#22497=EDGE_CURVE('',#17491,#17531,#7759,.T.);
#22498=EDGE_CURVE('',#17490,#17532,#7760,.T.);
#22499=EDGE_CURVE('',#17489,#17533,#7761,.T.);
#22500=EDGE_CURVE('',#18226,#18227,#7762,.T.);
#22501=EDGE_CURVE('',#17491,#18226,#17020,.T.);
#22502=EDGE_CURVE('',#17531,#18227,#17021,.T.);
#22503=EDGE_CURVE('',#18228,#17492,#17022,.T.);
#22504=EDGE_CURVE('',#18228,#18229,#7763,.T.);
#22505=EDGE_CURVE('',#18229,#17530,#17023,.T.);
#22506=EDGE_CURVE('',#18229,#18227,#7764,.T.);
#22507=EDGE_CURVE('',#18226,#18228,#7765,.T.);
#22508=EDGE_CURVE('',#18226,#18230,#7766,.T.);
#22509=EDGE_CURVE('',#18227,#18231,#7767,.T.);
#22510=EDGE_CURVE('',#18231,#18230,#7768,.T.);
#22511=EDGE_CURVE('',#18232,#18229,#7769,.T.);
#22512=EDGE_CURVE('',#18233,#18228,#7770,.T.);
#22513=EDGE_CURVE('',#18232,#18233,#7771,.T.);
#22514=EDGE_CURVE('',#18234,#18232,#17024,.T.);
#22515=EDGE_CURVE('',#18235,#18234,#7772,.T.);
#22516=EDGE_CURVE('',#18231,#18235,#17025,.T.);
#22517=EDGE_CURVE('',#18230,#18236,#17026,.T.);
#22518=EDGE_CURVE('',#18236,#18237,#7773,.T.);
#22519=EDGE_CURVE('',#18237,#18233,#17027,.T.);
#22520=EDGE_CURVE('',#18234,#18237,#7774,.T.);
#22521=EDGE_CURVE('',#18235,#18236,#7775,.T.);
#26477=ORIENTED_EDGE('',*,*,#20856,.F.);
#26478=ORIENTED_EDGE('',*,*,#20857,.T.);
#26479=ORIENTED_EDGE('',*,*,#20858,.T.);
#26480=ORIENTED_EDGE('',*,*,#20857,.F.);
#26481=ORIENTED_EDGE('',*,*,#20859,.F.);
#26482=ORIENTED_EDGE('',*,*,#20860,.T.);
#26483=ORIENTED_EDGE('',*,*,#20861,.T.);
#26484=ORIENTED_EDGE('',*,*,#20860,.F.);
#26485=ORIENTED_EDGE('',*,*,#20862,.F.);
#26486=ORIENTED_EDGE('',*,*,#20863,.T.);
#26487=ORIENTED_EDGE('',*,*,#20864,.T.);
#26488=ORIENTED_EDGE('',*,*,#20863,.F.);
#26489=ORIENTED_EDGE('',*,*,#20865,.F.);
#26490=ORIENTED_EDGE('',*,*,#20866,.T.);
#26491=ORIENTED_EDGE('',*,*,#20867,.T.);
#26492=ORIENTED_EDGE('',*,*,#20866,.F.);
#26493=ORIENTED_EDGE('',*,*,#20868,.F.);
#26494=ORIENTED_EDGE('',*,*,#20869,.T.);
#26495=ORIENTED_EDGE('',*,*,#20870,.T.);
#26496=ORIENTED_EDGE('',*,*,#20869,.F.);
#26497=ORIENTED_EDGE('',*,*,#20871,.T.);
#26498=ORIENTED_EDGE('',*,*,#20872,.T.);
#26499=ORIENTED_EDGE('',*,*,#20873,.F.);
#26500=ORIENTED_EDGE('',*,*,#20872,.F.);
#26501=ORIENTED_EDGE('',*,*,#20874,.F.);
#26502=ORIENTED_EDGE('',*,*,#20875,.T.);
#26503=ORIENTED_EDGE('',*,*,#20876,.T.);
#26504=ORIENTED_EDGE('',*,*,#20877,.F.);
#26505=ORIENTED_EDGE('',*,*,#20878,.T.);
#26506=ORIENTED_EDGE('',*,*,#20879,.T.);
#26507=ORIENTED_EDGE('',*,*,#20880,.F.);
#26508=ORIENTED_EDGE('',*,*,#20881,.F.);
#26509=ORIENTED_EDGE('',*,*,#20882,.T.);
#26510=ORIENTED_EDGE('',*,*,#20883,.T.);
#26511=ORIENTED_EDGE('',*,*,#20884,.F.);
#26512=ORIENTED_EDGE('',*,*,#20885,.F.);
#26513=ORIENTED_EDGE('',*,*,#20886,.T.);
#26514=ORIENTED_EDGE('',*,*,#20887,.T.);
#26515=ORIENTED_EDGE('',*,*,#20888,.F.);
#26516=ORIENTED_EDGE('',*,*,#20889,.F.);
#26517=ORIENTED_EDGE('',*,*,#20890,.T.);
#26518=ORIENTED_EDGE('',*,*,#20891,.T.);
#26519=ORIENTED_EDGE('',*,*,#20892,.F.);
#26520=ORIENTED_EDGE('',*,*,#20893,.F.);
#26521=ORIENTED_EDGE('',*,*,#20894,.T.);
#26522=ORIENTED_EDGE('',*,*,#20895,.T.);
#26523=ORIENTED_EDGE('',*,*,#20896,.F.);
#26524=ORIENTED_EDGE('',*,*,#20897,.F.);
#26525=ORIENTED_EDGE('',*,*,#20898,.F.);
#26526=ORIENTED_EDGE('',*,*,#20899,.T.);
#26527=ORIENTED_EDGE('',*,*,#20900,.T.);
#26528=ORIENTED_EDGE('',*,*,#20901,.F.);
#26529=ORIENTED_EDGE('',*,*,#20902,.F.);
#26530=ORIENTED_EDGE('',*,*,#20903,.T.);
#26531=ORIENTED_EDGE('',*,*,#20904,.T.);
#26532=ORIENTED_EDGE('',*,*,#20905,.F.);
#26533=ORIENTED_EDGE('',*,*,#20906,.F.);
#26534=ORIENTED_EDGE('',*,*,#20907,.T.);
#26535=ORIENTED_EDGE('',*,*,#20908,.T.);
#26536=ORIENTED_EDGE('',*,*,#20909,.F.);
#26537=ORIENTED_EDGE('',*,*,#20910,.F.);
#26538=ORIENTED_EDGE('',*,*,#20911,.T.);
#26539=ORIENTED_EDGE('',*,*,#20912,.T.);
#26540=ORIENTED_EDGE('',*,*,#20913,.F.);
#26541=ORIENTED_EDGE('',*,*,#20914,.F.);
#26542=ORIENTED_EDGE('',*,*,#20915,.T.);
#26543=ORIENTED_EDGE('',*,*,#20916,.T.);
#26544=ORIENTED_EDGE('',*,*,#20917,.F.);
#26545=ORIENTED_EDGE('',*,*,#20918,.F.);
#26546=ORIENTED_EDGE('',*,*,#20919,.T.);
#26547=ORIENTED_EDGE('',*,*,#20920,.T.);
#26548=ORIENTED_EDGE('',*,*,#20921,.F.);
#26549=ORIENTED_EDGE('',*,*,#20922,.F.);
#26550=ORIENTED_EDGE('',*,*,#20923,.T.);
#26551=ORIENTED_EDGE('',*,*,#20924,.T.);
#26552=ORIENTED_EDGE('',*,*,#20925,.F.);
#26553=ORIENTED_EDGE('',*,*,#20926,.T.);
#26554=ORIENTED_EDGE('',*,*,#20927,.T.);
#26555=ORIENTED_EDGE('',*,*,#20928,.F.);
#26556=ORIENTED_EDGE('',*,*,#20929,.F.);
#26557=ORIENTED_EDGE('',*,*,#20930,.T.);
#26558=ORIENTED_EDGE('',*,*,#20931,.T.);
#26559=ORIENTED_EDGE('',*,*,#20932,.F.);
#26560=ORIENTED_EDGE('',*,*,#20933,.F.);
#26561=ORIENTED_EDGE('',*,*,#20934,.T.);
#26562=ORIENTED_EDGE('',*,*,#20935,.T.);
#26563=ORIENTED_EDGE('',*,*,#20936,.F.);
#26564=ORIENTED_EDGE('',*,*,#20937,.F.);
#26565=ORIENTED_EDGE('',*,*,#20938,.T.);
#26566=ORIENTED_EDGE('',*,*,#20939,.T.);
#26567=ORIENTED_EDGE('',*,*,#20940,.F.);
#26568=ORIENTED_EDGE('',*,*,#20941,.F.);
#26569=ORIENTED_EDGE('',*,*,#20942,.F.);
#26570=ORIENTED_EDGE('',*,*,#20943,.T.);
#26571=ORIENTED_EDGE('',*,*,#20944,.T.);
#26572=ORIENTED_EDGE('',*,*,#20945,.F.);
#26573=ORIENTED_EDGE('',*,*,#20946,.F.);
#26574=ORIENTED_EDGE('',*,*,#20947,.T.);
#26575=ORIENTED_EDGE('',*,*,#20948,.T.);
#26576=ORIENTED_EDGE('',*,*,#20949,.F.);
#26577=ORIENTED_EDGE('',*,*,#20950,.T.);
#26578=ORIENTED_EDGE('',*,*,#20951,.T.);
#26579=ORIENTED_EDGE('',*,*,#20952,.F.);
#26580=ORIENTED_EDGE('',*,*,#20953,.F.);
#26581=ORIENTED_EDGE('',*,*,#20954,.F.);
#26582=ORIENTED_EDGE('',*,*,#20955,.T.);
#26583=ORIENTED_EDGE('',*,*,#20956,.T.);
#26584=ORIENTED_EDGE('',*,*,#20957,.F.);
#26585=ORIENTED_EDGE('',*,*,#20958,.T.);
#26586=ORIENTED_EDGE('',*,*,#20959,.T.);
#26587=ORIENTED_EDGE('',*,*,#20960,.F.);
#26588=ORIENTED_EDGE('',*,*,#20961,.F.);
#26589=ORIENTED_EDGE('',*,*,#20962,.T.);
#26590=ORIENTED_EDGE('',*,*,#20963,.T.);
#26591=ORIENTED_EDGE('',*,*,#20964,.F.);
#26592=ORIENTED_EDGE('',*,*,#20965,.F.);
#26593=ORIENTED_EDGE('',*,*,#20966,.F.);
#26594=ORIENTED_EDGE('',*,*,#20967,.T.);
#26595=ORIENTED_EDGE('',*,*,#20968,.T.);
#26596=ORIENTED_EDGE('',*,*,#20969,.F.);
#26597=ORIENTED_EDGE('',*,*,#20970,.T.);
#26598=ORIENTED_EDGE('',*,*,#20971,.T.);
#26599=ORIENTED_EDGE('',*,*,#20972,.F.);
#26600=ORIENTED_EDGE('',*,*,#20973,.F.);
#26601=ORIENTED_EDGE('',*,*,#20974,.F.);
#26602=ORIENTED_EDGE('',*,*,#20975,.T.);
#26603=ORIENTED_EDGE('',*,*,#20976,.T.);
#26604=ORIENTED_EDGE('',*,*,#20977,.F.);
#26605=ORIENTED_EDGE('',*,*,#20978,.F.);
#26606=ORIENTED_EDGE('',*,*,#20979,.T.);
#26607=ORIENTED_EDGE('',*,*,#20980,.T.);
#26608=ORIENTED_EDGE('',*,*,#20981,.F.);
#26609=ORIENTED_EDGE('',*,*,#20982,.F.);
#26610=ORIENTED_EDGE('',*,*,#20983,.T.);
#26611=ORIENTED_EDGE('',*,*,#20984,.T.);
#26612=ORIENTED_EDGE('',*,*,#20985,.F.);
#26613=ORIENTED_EDGE('',*,*,#20986,.F.);
#26614=ORIENTED_EDGE('',*,*,#20987,.T.);
#26615=ORIENTED_EDGE('',*,*,#20988,.T.);
#26616=ORIENTED_EDGE('',*,*,#20989,.F.);
#26617=ORIENTED_EDGE('',*,*,#20990,.F.);
#26618=ORIENTED_EDGE('',*,*,#20991,.T.);
#26619=ORIENTED_EDGE('',*,*,#20992,.T.);
#26620=ORIENTED_EDGE('',*,*,#20993,.F.);
#26621=ORIENTED_EDGE('',*,*,#20994,.T.);
#26622=ORIENTED_EDGE('',*,*,#20995,.T.);
#26623=ORIENTED_EDGE('',*,*,#20996,.F.);
#26624=ORIENTED_EDGE('',*,*,#20997,.F.);
#26625=ORIENTED_EDGE('',*,*,#20998,.T.);
#26626=ORIENTED_EDGE('',*,*,#20999,.T.);
#26627=ORIENTED_EDGE('',*,*,#21000,.F.);
#26628=ORIENTED_EDGE('',*,*,#21001,.F.);
#26629=ORIENTED_EDGE('',*,*,#21002,.T.);
#26630=ORIENTED_EDGE('',*,*,#21003,.T.);
#26631=ORIENTED_EDGE('',*,*,#21004,.F.);
#26632=ORIENTED_EDGE('',*,*,#21005,.F.);
#26633=ORIENTED_EDGE('',*,*,#21006,.T.);
#26634=ORIENTED_EDGE('',*,*,#21007,.T.);
#26635=ORIENTED_EDGE('',*,*,#21008,.F.);
#26636=ORIENTED_EDGE('',*,*,#21009,.F.);
#26637=ORIENTED_EDGE('',*,*,#21010,.T.);
#26638=ORIENTED_EDGE('',*,*,#21011,.T.);
#26639=ORIENTED_EDGE('',*,*,#21012,.F.);
#26640=ORIENTED_EDGE('',*,*,#21013,.F.);
#26641=ORIENTED_EDGE('',*,*,#21014,.T.);
#26642=ORIENTED_EDGE('',*,*,#21015,.T.);
#26643=ORIENTED_EDGE('',*,*,#21016,.F.);
#26644=ORIENTED_EDGE('',*,*,#21017,.F.);
#26645=ORIENTED_EDGE('',*,*,#21018,.T.);
#26646=ORIENTED_EDGE('',*,*,#21019,.T.);
#26647=ORIENTED_EDGE('',*,*,#21020,.F.);
#26648=ORIENTED_EDGE('',*,*,#21021,.F.);
#26649=ORIENTED_EDGE('',*,*,#21022,.F.);
#26650=ORIENTED_EDGE('',*,*,#21023,.T.);
#26651=ORIENTED_EDGE('',*,*,#21024,.T.);
#26652=ORIENTED_EDGE('',*,*,#21025,.F.);
#26653=ORIENTED_EDGE('',*,*,#21026,.F.);
#26654=ORIENTED_EDGE('',*,*,#21027,.T.);
#26655=ORIENTED_EDGE('',*,*,#21028,.T.);
#26656=ORIENTED_EDGE('',*,*,#21029,.F.);
#26657=ORIENTED_EDGE('',*,*,#21030,.F.);
#26658=ORIENTED_EDGE('',*,*,#21031,.T.);
#26659=ORIENTED_EDGE('',*,*,#21032,.T.);
#26660=ORIENTED_EDGE('',*,*,#21033,.F.);
#26661=ORIENTED_EDGE('',*,*,#21034,.F.);
#26662=ORIENTED_EDGE('',*,*,#21035,.T.);
#26663=ORIENTED_EDGE('',*,*,#21036,.T.);
#26664=ORIENTED_EDGE('',*,*,#21037,.F.);
#26665=ORIENTED_EDGE('',*,*,#21038,.T.);
#26666=ORIENTED_EDGE('',*,*,#21039,.T.);
#26667=ORIENTED_EDGE('',*,*,#21040,.F.);
#26668=ORIENTED_EDGE('',*,*,#21041,.F.);
#26669=ORIENTED_EDGE('',*,*,#21042,.T.);
#26670=ORIENTED_EDGE('',*,*,#21043,.T.);
#26671=ORIENTED_EDGE('',*,*,#21044,.F.);
#26672=ORIENTED_EDGE('',*,*,#21045,.F.);
#26673=ORIENTED_EDGE('',*,*,#21046,.F.);
#26674=ORIENTED_EDGE('',*,*,#21047,.T.);
#26675=ORIENTED_EDGE('',*,*,#21048,.T.);
#26676=ORIENTED_EDGE('',*,*,#21049,.F.);
#26677=ORIENTED_EDGE('',*,*,#21050,.T.);
#26678=ORIENTED_EDGE('',*,*,#21051,.T.);
#26679=ORIENTED_EDGE('',*,*,#21052,.F.);
#26680=ORIENTED_EDGE('',*,*,#21053,.F.);
#26681=ORIENTED_EDGE('',*,*,#21054,.F.);
#26682=ORIENTED_EDGE('',*,*,#21055,.T.);
#26683=ORIENTED_EDGE('',*,*,#21056,.T.);
#26684=ORIENTED_EDGE('',*,*,#21057,.F.);
#26685=ORIENTED_EDGE('',*,*,#21058,.F.);
#26686=ORIENTED_EDGE('',*,*,#21059,.T.);
#26687=ORIENTED_EDGE('',*,*,#21060,.T.);
#26688=ORIENTED_EDGE('',*,*,#21061,.F.);
#26689=ORIENTED_EDGE('',*,*,#21062,.T.);
#26690=ORIENTED_EDGE('',*,*,#21063,.T.);
#26691=ORIENTED_EDGE('',*,*,#21064,.F.);
#26692=ORIENTED_EDGE('',*,*,#21065,.F.);
#26693=ORIENTED_EDGE('',*,*,#21066,.F.);
#26694=ORIENTED_EDGE('',*,*,#21067,.F.);
#26695=ORIENTED_EDGE('',*,*,#21068,.F.);
#26696=ORIENTED_EDGE('',*,*,#21069,.F.);
#26697=ORIENTED_EDGE('',*,*,#21070,.F.);
#26698=ORIENTED_EDGE('',*,*,#21071,.F.);
#26699=ORIENTED_EDGE('',*,*,#21072,.F.);
#26700=ORIENTED_EDGE('',*,*,#21073,.F.);
#26701=ORIENTED_EDGE('',*,*,#21074,.F.);
#26702=ORIENTED_EDGE('',*,*,#21075,.F.);
#26703=ORIENTED_EDGE('',*,*,#21076,.F.);
#26704=ORIENTED_EDGE('',*,*,#21077,.F.);
#26705=ORIENTED_EDGE('',*,*,#21078,.F.);
#26706=ORIENTED_EDGE('',*,*,#21079,.F.);
#26707=ORIENTED_EDGE('',*,*,#21080,.F.);
#26708=ORIENTED_EDGE('',*,*,#21081,.F.);
#26709=ORIENTED_EDGE('',*,*,#21082,.F.);
#26710=ORIENTED_EDGE('',*,*,#21083,.F.);
#26711=ORIENTED_EDGE('',*,*,#21084,.F.);
#26712=ORIENTED_EDGE('',*,*,#21085,.F.);
#26713=ORIENTED_EDGE('',*,*,#21086,.F.);
#26714=ORIENTED_EDGE('',*,*,#21087,.F.);
#26715=ORIENTED_EDGE('',*,*,#21088,.F.);
#26716=ORIENTED_EDGE('',*,*,#21089,.F.);
#26717=ORIENTED_EDGE('',*,*,#21090,.F.);
#26718=ORIENTED_EDGE('',*,*,#21091,.F.);
#26719=ORIENTED_EDGE('',*,*,#21092,.F.);
#26720=ORIENTED_EDGE('',*,*,#21093,.F.);
#26721=ORIENTED_EDGE('',*,*,#21094,.F.);
#26722=ORIENTED_EDGE('',*,*,#21095,.F.);
#26723=ORIENTED_EDGE('',*,*,#21096,.F.);
#26724=ORIENTED_EDGE('',*,*,#21097,.F.);
#26725=ORIENTED_EDGE('',*,*,#21098,.F.);
#26726=ORIENTED_EDGE('',*,*,#21099,.F.);
#26727=ORIENTED_EDGE('',*,*,#21100,.F.);
#26728=ORIENTED_EDGE('',*,*,#21101,.F.);
#26729=ORIENTED_EDGE('',*,*,#21102,.F.);
#26730=ORIENTED_EDGE('',*,*,#21103,.F.);
#26731=ORIENTED_EDGE('',*,*,#21104,.F.);
#26732=ORIENTED_EDGE('',*,*,#21105,.F.);
#26733=ORIENTED_EDGE('',*,*,#21106,.F.);
#26734=ORIENTED_EDGE('',*,*,#21107,.F.);
#26735=ORIENTED_EDGE('',*,*,#21108,.F.);
#26736=ORIENTED_EDGE('',*,*,#21109,.F.);
#26737=ORIENTED_EDGE('',*,*,#21110,.F.);
#26738=ORIENTED_EDGE('',*,*,#21111,.F.);
#26739=ORIENTED_EDGE('',*,*,#21112,.F.);
#26740=ORIENTED_EDGE('',*,*,#21113,.F.);
#26741=ORIENTED_EDGE('',*,*,#21114,.F.);
#26742=ORIENTED_EDGE('',*,*,#21115,.F.);
#26743=ORIENTED_EDGE('',*,*,#21116,.F.);
#26744=ORIENTED_EDGE('',*,*,#21117,.F.);
#26745=ORIENTED_EDGE('',*,*,#21118,.F.);
#26746=ORIENTED_EDGE('',*,*,#21119,.F.);
#26747=ORIENTED_EDGE('',*,*,#21120,.F.);
#26748=ORIENTED_EDGE('',*,*,#21121,.F.);
#26749=ORIENTED_EDGE('',*,*,#21122,.F.);
#26750=ORIENTED_EDGE('',*,*,#21123,.F.);
#26751=ORIENTED_EDGE('',*,*,#21124,.F.);
#26752=ORIENTED_EDGE('',*,*,#21125,.F.);
#26753=ORIENTED_EDGE('',*,*,#21126,.F.);
#26754=ORIENTED_EDGE('',*,*,#21127,.F.);
#26755=ORIENTED_EDGE('',*,*,#21128,.F.);
#26756=ORIENTED_EDGE('',*,*,#21129,.F.);
#26757=ORIENTED_EDGE('',*,*,#21130,.F.);
#26758=ORIENTED_EDGE('',*,*,#21131,.F.);
#26759=ORIENTED_EDGE('',*,*,#21132,.F.);
#26760=ORIENTED_EDGE('',*,*,#21133,.F.);
#26761=ORIENTED_EDGE('',*,*,#21134,.F.);
#26762=ORIENTED_EDGE('',*,*,#21135,.F.);
#26763=ORIENTED_EDGE('',*,*,#21136,.F.);
#26764=ORIENTED_EDGE('',*,*,#21137,.F.);
#26765=ORIENTED_EDGE('',*,*,#21138,.F.);
#26766=ORIENTED_EDGE('',*,*,#21139,.T.);
#26767=ORIENTED_EDGE('',*,*,#21140,.F.);
#26768=ORIENTED_EDGE('',*,*,#21141,.T.);
#26769=ORIENTED_EDGE('',*,*,#21142,.F.);
#26770=ORIENTED_EDGE('',*,*,#21143,.T.);
#26771=ORIENTED_EDGE('',*,*,#21144,.F.);
#26772=ORIENTED_EDGE('',*,*,#21145,.T.);
#26773=ORIENTED_EDGE('',*,*,#21146,.T.);
#26774=ORIENTED_EDGE('',*,*,#21147,.T.);
#26775=ORIENTED_EDGE('',*,*,#21148,.F.);
#26776=ORIENTED_EDGE('',*,*,#21149,.T.);
#26777=ORIENTED_EDGE('',*,*,#21150,.F.);
#26778=ORIENTED_EDGE('',*,*,#21151,.T.);
#26779=ORIENTED_EDGE('',*,*,#21152,.F.);
#26780=ORIENTED_EDGE('',*,*,#21153,.T.);
#26781=ORIENTED_EDGE('',*,*,#21154,.T.);
#26782=ORIENTED_EDGE('',*,*,#21155,.T.);
#26783=ORIENTED_EDGE('',*,*,#21156,.F.);
#26784=ORIENTED_EDGE('',*,*,#21157,.T.);
#26785=ORIENTED_EDGE('',*,*,#21158,.T.);
#26786=ORIENTED_EDGE('',*,*,#21159,.T.);
#26787=ORIENTED_EDGE('',*,*,#21160,.F.);
#26788=ORIENTED_EDGE('',*,*,#21159,.F.);
#26789=ORIENTED_EDGE('',*,*,#21161,.F.);
#26790=ORIENTED_EDGE('',*,*,#21162,.T.);
#26791=ORIENTED_EDGE('',*,*,#21163,.T.);
#26792=ORIENTED_EDGE('',*,*,#21162,.F.);
#26793=ORIENTED_EDGE('',*,*,#21164,.T.);
#26794=ORIENTED_EDGE('',*,*,#21165,.T.);
#26795=ORIENTED_EDGE('',*,*,#21166,.F.);
#26796=ORIENTED_EDGE('',*,*,#21165,.F.);
#26797=ORIENTED_EDGE('',*,*,#21167,.F.);
#26798=ORIENTED_EDGE('',*,*,#21168,.T.);
#26799=ORIENTED_EDGE('',*,*,#21169,.T.);
#26800=ORIENTED_EDGE('',*,*,#21168,.F.);
#26801=ORIENTED_EDGE('',*,*,#21170,.F.);
#26802=ORIENTED_EDGE('',*,*,#21171,.T.);
#26803=ORIENTED_EDGE('',*,*,#21172,.T.);
#26804=ORIENTED_EDGE('',*,*,#21171,.F.);
#26805=ORIENTED_EDGE('',*,*,#21173,.F.);
#26806=ORIENTED_EDGE('',*,*,#21174,.T.);
#26807=ORIENTED_EDGE('',*,*,#21175,.T.);
#26808=ORIENTED_EDGE('',*,*,#21174,.F.);
#26809=ORIENTED_EDGE('',*,*,#21176,.F.);
#26810=ORIENTED_EDGE('',*,*,#21177,.T.);
#26811=ORIENTED_EDGE('',*,*,#21173,.T.);
#26812=ORIENTED_EDGE('',*,*,#21177,.F.);
#26813=ORIENTED_EDGE('',*,*,#21178,.T.);
#26814=ORIENTED_EDGE('',*,*,#21179,.T.);
#26815=ORIENTED_EDGE('',*,*,#21170,.T.);
#26816=ORIENTED_EDGE('',*,*,#21179,.F.);
#26817=ORIENTED_EDGE('',*,*,#21180,.T.);
#26818=ORIENTED_EDGE('',*,*,#21181,.T.);
#26819=ORIENTED_EDGE('',*,*,#21182,.F.);
#26820=ORIENTED_EDGE('',*,*,#21181,.F.);
#26821=ORIENTED_EDGE('',*,*,#21183,.T.);
#26822=ORIENTED_EDGE('',*,*,#21184,.T.);
#26823=ORIENTED_EDGE('',*,*,#21185,.F.);
#26824=ORIENTED_EDGE('',*,*,#21184,.F.);
#26825=ORIENTED_EDGE('',*,*,#21186,.T.);
#26826=ORIENTED_EDGE('',*,*,#21187,.T.);
#26827=ORIENTED_EDGE('',*,*,#21188,.F.);
#26828=ORIENTED_EDGE('',*,*,#21187,.F.);
#26829=ORIENTED_EDGE('',*,*,#21189,.T.);
#26830=ORIENTED_EDGE('',*,*,#21190,.T.);
#26831=ORIENTED_EDGE('',*,*,#21191,.F.);
#26832=ORIENTED_EDGE('',*,*,#21190,.F.);
#26833=ORIENTED_EDGE('',*,*,#21192,.T.);
#26834=ORIENTED_EDGE('',*,*,#21193,.T.);
#26835=ORIENTED_EDGE('',*,*,#21194,.F.);
#26836=ORIENTED_EDGE('',*,*,#21195,.T.);
#26837=ORIENTED_EDGE('',*,*,#21196,.F.);
#26838=ORIENTED_EDGE('',*,*,#21197,.T.);
#26839=ORIENTED_EDGE('',*,*,#21198,.F.);
#26840=ORIENTED_EDGE('',*,*,#21199,.F.);
#26841=ORIENTED_EDGE('',*,*,#21200,.F.);
#26842=ORIENTED_EDGE('',*,*,#21201,.F.);
#26843=ORIENTED_EDGE('',*,*,#21202,.F.);
#26844=ORIENTED_EDGE('',*,*,#21203,.F.);
#26845=ORIENTED_EDGE('',*,*,#21204,.F.);
#26846=ORIENTED_EDGE('',*,*,#21205,.F.);
#26847=ORIENTED_EDGE('',*,*,#21206,.F.);
#26848=ORIENTED_EDGE('',*,*,#21207,.F.);
#26849=ORIENTED_EDGE('',*,*,#21208,.F.);
#26850=ORIENTED_EDGE('',*,*,#21209,.F.);
#26851=ORIENTED_EDGE('',*,*,#21210,.F.);
#26852=ORIENTED_EDGE('',*,*,#21211,.F.);
#26853=ORIENTED_EDGE('',*,*,#21212,.F.);
#26854=ORIENTED_EDGE('',*,*,#21213,.F.);
#26855=ORIENTED_EDGE('',*,*,#21214,.T.);
#26856=ORIENTED_EDGE('',*,*,#21215,.F.);
#26857=ORIENTED_EDGE('',*,*,#21216,.F.);
#26858=ORIENTED_EDGE('',*,*,#21217,.T.);
#26859=ORIENTED_EDGE('',*,*,#21218,.F.);
#26860=ORIENTED_EDGE('',*,*,#21219,.F.);
#26861=ORIENTED_EDGE('',*,*,#21220,.F.);
#26862=ORIENTED_EDGE('',*,*,#21221,.F.);
#26863=ORIENTED_EDGE('',*,*,#21222,.F.);
#26864=ORIENTED_EDGE('',*,*,#21223,.F.);
#26865=ORIENTED_EDGE('',*,*,#21224,.F.);
#26866=ORIENTED_EDGE('',*,*,#21225,.T.);
#26867=ORIENTED_EDGE('',*,*,#21226,.F.);
#26868=ORIENTED_EDGE('',*,*,#21227,.T.);
#26869=ORIENTED_EDGE('',*,*,#21228,.F.);
#26870=ORIENTED_EDGE('',*,*,#21229,.F.);
#26871=ORIENTED_EDGE('',*,*,#21230,.F.);
#26872=ORIENTED_EDGE('',*,*,#21231,.T.);
#26873=ORIENTED_EDGE('',*,*,#21232,.F.);
#26874=ORIENTED_EDGE('',*,*,#21233,.T.);
#26875=ORIENTED_EDGE('',*,*,#21234,.F.);
#26876=ORIENTED_EDGE('',*,*,#21235,.T.);
#26877=ORIENTED_EDGE('',*,*,#21236,.F.);
#26878=ORIENTED_EDGE('',*,*,#21237,.F.);
#26879=ORIENTED_EDGE('',*,*,#21238,.F.);
#26880=ORIENTED_EDGE('',*,*,#21239,.T.);
#26881=ORIENTED_EDGE('',*,*,#21240,.F.);
#26882=ORIENTED_EDGE('',*,*,#21241,.T.);
#26883=ORIENTED_EDGE('',*,*,#21242,.F.);
#26884=ORIENTED_EDGE('',*,*,#21243,.T.);
#26885=ORIENTED_EDGE('',*,*,#21244,.F.);
#26886=ORIENTED_EDGE('',*,*,#21245,.F.);
#26887=ORIENTED_EDGE('',*,*,#21246,.F.);
#26888=ORIENTED_EDGE('',*,*,#21247,.T.);
#26889=ORIENTED_EDGE('',*,*,#21248,.F.);
#26890=ORIENTED_EDGE('',*,*,#21249,.T.);
#26891=ORIENTED_EDGE('',*,*,#21250,.F.);
#26892=ORIENTED_EDGE('',*,*,#21251,.T.);
#26893=ORIENTED_EDGE('',*,*,#21252,.F.);
#26894=ORIENTED_EDGE('',*,*,#21253,.F.);
#26895=ORIENTED_EDGE('',*,*,#21254,.F.);
#26896=ORIENTED_EDGE('',*,*,#21255,.T.);
#26897=ORIENTED_EDGE('',*,*,#21256,.F.);
#26898=ORIENTED_EDGE('',*,*,#21257,.T.);
#26899=ORIENTED_EDGE('',*,*,#21258,.T.);
#26900=ORIENTED_EDGE('',*,*,#21259,.T.);
#26901=ORIENTED_EDGE('',*,*,#21260,.T.);
#26902=ORIENTED_EDGE('',*,*,#21261,.T.);
#26903=ORIENTED_EDGE('',*,*,#21262,.T.);
#26904=ORIENTED_EDGE('',*,*,#21263,.T.);
#26905=ORIENTED_EDGE('',*,*,#21264,.F.);
#26906=ORIENTED_EDGE('',*,*,#21265,.F.);
#26907=ORIENTED_EDGE('',*,*,#21266,.F.);
#26908=ORIENTED_EDGE('',*,*,#21267,.F.);
#26909=ORIENTED_EDGE('',*,*,#21268,.F.);
#26910=ORIENTED_EDGE('',*,*,#21269,.F.);
#26911=ORIENTED_EDGE('',*,*,#21270,.T.);
#26912=ORIENTED_EDGE('',*,*,#21271,.T.);
#26913=ORIENTED_EDGE('',*,*,#21272,.T.);
#26914=ORIENTED_EDGE('',*,*,#21273,.T.);
#26915=ORIENTED_EDGE('',*,*,#21274,.T.);
#26916=ORIENTED_EDGE('',*,*,#21275,.T.);
#26917=ORIENTED_EDGE('',*,*,#21276,.T.);
#26918=ORIENTED_EDGE('',*,*,#21277,.T.);
#26919=ORIENTED_EDGE('',*,*,#21278,.T.);
#26920=ORIENTED_EDGE('',*,*,#21279,.F.);
#26921=ORIENTED_EDGE('',*,*,#21280,.F.);
#26922=ORIENTED_EDGE('',*,*,#21281,.T.);
#26923=ORIENTED_EDGE('',*,*,#21282,.F.);
#26924=ORIENTED_EDGE('',*,*,#21283,.F.);
#26925=ORIENTED_EDGE('',*,*,#21284,.F.);
#26926=ORIENTED_EDGE('',*,*,#21285,.F.);
#26927=ORIENTED_EDGE('',*,*,#21286,.T.);
#26928=ORIENTED_EDGE('',*,*,#21287,.F.);
#26929=ORIENTED_EDGE('',*,*,#21288,.F.);
#26930=ORIENTED_EDGE('',*,*,#21289,.F.);
#26931=ORIENTED_EDGE('',*,*,#21290,.T.);
#26932=ORIENTED_EDGE('',*,*,#21291,.F.);
#26933=ORIENTED_EDGE('',*,*,#21292,.F.);
#26934=ORIENTED_EDGE('',*,*,#21293,.F.);
#26935=ORIENTED_EDGE('',*,*,#21294,.T.);
#26936=ORIENTED_EDGE('',*,*,#21295,.F.);
#26937=ORIENTED_EDGE('',*,*,#21296,.F.);
#26938=ORIENTED_EDGE('',*,*,#21297,.F.);
#26939=ORIENTED_EDGE('',*,*,#21298,.T.);
#26940=ORIENTED_EDGE('',*,*,#21299,.F.);
#26941=ORIENTED_EDGE('',*,*,#21197,.F.);
#26942=ORIENTED_EDGE('',*,*,#21300,.T.);
#26943=ORIENTED_EDGE('',*,*,#21256,.T.);
#26944=ORIENTED_EDGE('',*,*,#21301,.F.);
#26945=ORIENTED_EDGE('',*,*,#21264,.T.);
#26946=ORIENTED_EDGE('',*,*,#21302,.F.);
#26947=ORIENTED_EDGE('',*,*,#21217,.F.);
#26948=ORIENTED_EDGE('',*,*,#21303,.F.);
#26949=ORIENTED_EDGE('',*,*,#21304,.F.);
#26950=ORIENTED_EDGE('',*,*,#21305,.F.);
#26951=ORIENTED_EDGE('',*,*,#21306,.F.);
#26952=ORIENTED_EDGE('',*,*,#21307,.F.);
#26953=ORIENTED_EDGE('',*,*,#21308,.F.);
#26954=ORIENTED_EDGE('',*,*,#21309,.F.);
#26955=ORIENTED_EDGE('',*,*,#21310,.T.);
#26956=ORIENTED_EDGE('',*,*,#21311,.T.);
#26957=ORIENTED_EDGE('',*,*,#21312,.F.);
#26958=ORIENTED_EDGE('',*,*,#21313,.T.);
#26959=ORIENTED_EDGE('',*,*,#21314,.T.);
#26960=ORIENTED_EDGE('',*,*,#21315,.T.);
#26961=ORIENTED_EDGE('',*,*,#21316,.T.);
#26962=ORIENTED_EDGE('',*,*,#21317,.T.);
#26963=ORIENTED_EDGE('',*,*,#21318,.F.);
#26964=ORIENTED_EDGE('',*,*,#21319,.T.);
#26965=ORIENTED_EDGE('',*,*,#21320,.F.);
#26966=ORIENTED_EDGE('',*,*,#21321,.T.);
#26967=ORIENTED_EDGE('',*,*,#21322,.F.);
#26968=ORIENTED_EDGE('',*,*,#21323,.T.);
#26969=ORIENTED_EDGE('',*,*,#21324,.T.);
#26970=ORIENTED_EDGE('',*,*,#21325,.T.);
#26971=ORIENTED_EDGE('',*,*,#21326,.F.);
#26972=ORIENTED_EDGE('',*,*,#21327,.T.);
#26973=ORIENTED_EDGE('',*,*,#21328,.T.);
#26974=ORIENTED_EDGE('',*,*,#21329,.T.);
#26975=ORIENTED_EDGE('',*,*,#21330,.T.);
#26976=ORIENTED_EDGE('',*,*,#21331,.T.);
#26977=ORIENTED_EDGE('',*,*,#21332,.F.);
#26978=ORIENTED_EDGE('',*,*,#21333,.F.);
#26979=ORIENTED_EDGE('',*,*,#21334,.T.);
#26980=ORIENTED_EDGE('',*,*,#21335,.F.);
#26981=ORIENTED_EDGE('',*,*,#21336,.T.);
#26982=ORIENTED_EDGE('',*,*,#21337,.T.);
#26983=ORIENTED_EDGE('',*,*,#21338,.T.);
#26984=ORIENTED_EDGE('',*,*,#21339,.F.);
#26985=ORIENTED_EDGE('',*,*,#21211,.T.);
#26986=ORIENTED_EDGE('',*,*,#21340,.T.);
#26987=ORIENTED_EDGE('',*,*,#21270,.F.);
#26988=ORIENTED_EDGE('',*,*,#21341,.F.);
#26989=ORIENTED_EDGE('',*,*,#21278,.F.);
#26990=ORIENTED_EDGE('',*,*,#21342,.F.);
#26991=ORIENTED_EDGE('',*,*,#21203,.T.);
#26992=ORIENTED_EDGE('',*,*,#21343,.F.);
#26993=ORIENTED_EDGE('',*,*,#21344,.F.);
#26994=ORIENTED_EDGE('',*,*,#21345,.T.);
#26995=ORIENTED_EDGE('',*,*,#21346,.F.);
#26996=ORIENTED_EDGE('',*,*,#21347,.T.);
#26997=ORIENTED_EDGE('',*,*,#21348,.T.);
#26998=ORIENTED_EDGE('',*,*,#21349,.F.);
#26999=ORIENTED_EDGE('',*,*,#21350,.F.);
#27000=ORIENTED_EDGE('',*,*,#21351,.T.);
#27001=ORIENTED_EDGE('',*,*,#21352,.F.);
#27002=ORIENTED_EDGE('',*,*,#21353,.F.);
#27003=ORIENTED_EDGE('',*,*,#21354,.T.);
#27004=ORIENTED_EDGE('',*,*,#21064,.T.);
#27005=ORIENTED_EDGE('',*,*,#21355,.F.);
#27006=ORIENTED_EDGE('',*,*,#21356,.T.);
#27007=ORIENTED_EDGE('',*,*,#21357,.T.);
#27008=ORIENTED_EDGE('',*,*,#21052,.T.);
#27009=ORIENTED_EDGE('',*,*,#21358,.F.);
#27010=ORIENTED_EDGE('',*,*,#21359,.T.);
#27011=ORIENTED_EDGE('',*,*,#21360,.T.);
#27012=ORIENTED_EDGE('',*,*,#21044,.T.);
#27013=ORIENTED_EDGE('',*,*,#21361,.F.);
#27014=ORIENTED_EDGE('',*,*,#21362,.T.);
#27015=ORIENTED_EDGE('',*,*,#21363,.T.);
#27016=ORIENTED_EDGE('',*,*,#21040,.T.);
#27017=ORIENTED_EDGE('',*,*,#21364,.F.);
#27018=ORIENTED_EDGE('',*,*,#21365,.T.);
#27019=ORIENTED_EDGE('',*,*,#21366,.T.);
#27020=ORIENTED_EDGE('',*,*,#21020,.T.);
#27021=ORIENTED_EDGE('',*,*,#21367,.F.);
#27022=ORIENTED_EDGE('',*,*,#21368,.T.);
#27023=ORIENTED_EDGE('',*,*,#21369,.T.);
#27024=ORIENTED_EDGE('',*,*,#21016,.T.);
#27025=ORIENTED_EDGE('',*,*,#21370,.F.);
#27026=ORIENTED_EDGE('',*,*,#21371,.T.);
#27027=ORIENTED_EDGE('',*,*,#21372,.T.);
#27028=ORIENTED_EDGE('',*,*,#21012,.T.);
#27029=ORIENTED_EDGE('',*,*,#21373,.F.);
#27030=ORIENTED_EDGE('',*,*,#21374,.T.);
#27031=ORIENTED_EDGE('',*,*,#21375,.T.);
#27032=ORIENTED_EDGE('',*,*,#21008,.T.);
#27033=ORIENTED_EDGE('',*,*,#21376,.F.);
#27034=ORIENTED_EDGE('',*,*,#21377,.T.);
#27035=ORIENTED_EDGE('',*,*,#21378,.T.);
#27036=ORIENTED_EDGE('',*,*,#21004,.T.);
#27037=ORIENTED_EDGE('',*,*,#21379,.F.);
#27038=ORIENTED_EDGE('',*,*,#21380,.T.);
#27039=ORIENTED_EDGE('',*,*,#21381,.T.);
#27040=ORIENTED_EDGE('',*,*,#21000,.T.);
#27041=ORIENTED_EDGE('',*,*,#21382,.F.);
#27042=ORIENTED_EDGE('',*,*,#21383,.T.);
#27043=ORIENTED_EDGE('',*,*,#21384,.T.);
#27044=ORIENTED_EDGE('',*,*,#20996,.T.);
#27045=ORIENTED_EDGE('',*,*,#21385,.F.);
#27046=ORIENTED_EDGE('',*,*,#21386,.T.);
#27047=ORIENTED_EDGE('',*,*,#21387,.T.);
#27048=ORIENTED_EDGE('',*,*,#20972,.T.);
#27049=ORIENTED_EDGE('',*,*,#21388,.F.);
#27050=ORIENTED_EDGE('',*,*,#21389,.T.);
#27051=ORIENTED_EDGE('',*,*,#20964,.T.);
#27052=ORIENTED_EDGE('',*,*,#21390,.T.);
#27053=ORIENTED_EDGE('',*,*,#21391,.T.);
#27054=ORIENTED_EDGE('',*,*,#21392,.F.);
#27055=ORIENTED_EDGE('',*,*,#20960,.T.);
#27056=ORIENTED_EDGE('',*,*,#21393,.T.);
#27057=ORIENTED_EDGE('',*,*,#21394,.T.);
#27058=ORIENTED_EDGE('',*,*,#21395,.F.);
#27059=ORIENTED_EDGE('',*,*,#20952,.T.);
#27060=ORIENTED_EDGE('',*,*,#21396,.T.);
#27061=ORIENTED_EDGE('',*,*,#21397,.T.);
#27062=ORIENTED_EDGE('',*,*,#21398,.F.);
#27063=ORIENTED_EDGE('',*,*,#20940,.T.);
#27064=ORIENTED_EDGE('',*,*,#21399,.T.);
#27065=ORIENTED_EDGE('',*,*,#21400,.T.);
#27066=ORIENTED_EDGE('',*,*,#21401,.F.);
#27067=ORIENTED_EDGE('',*,*,#20936,.T.);
#27068=ORIENTED_EDGE('',*,*,#21402,.T.);
#27069=ORIENTED_EDGE('',*,*,#21403,.T.);
#27070=ORIENTED_EDGE('',*,*,#21404,.F.);
#27071=ORIENTED_EDGE('',*,*,#20932,.T.);
#27072=ORIENTED_EDGE('',*,*,#21405,.T.);
#27073=ORIENTED_EDGE('',*,*,#21406,.T.);
#27074=ORIENTED_EDGE('',*,*,#21407,.F.);
#27075=ORIENTED_EDGE('',*,*,#20928,.T.);
#27076=ORIENTED_EDGE('',*,*,#21408,.T.);
#27077=ORIENTED_EDGE('',*,*,#21409,.T.);
#27078=ORIENTED_EDGE('',*,*,#21410,.F.);
#27079=ORIENTED_EDGE('',*,*,#20896,.T.);
#27080=ORIENTED_EDGE('',*,*,#21411,.T.);
#27081=ORIENTED_EDGE('',*,*,#21412,.T.);
#27082=ORIENTED_EDGE('',*,*,#21413,.F.);
#27083=ORIENTED_EDGE('',*,*,#20892,.T.);
#27084=ORIENTED_EDGE('',*,*,#21414,.T.);
#27085=ORIENTED_EDGE('',*,*,#21415,.T.);
#27086=ORIENTED_EDGE('',*,*,#21416,.F.);
#27087=ORIENTED_EDGE('',*,*,#20888,.T.);
#27088=ORIENTED_EDGE('',*,*,#21417,.T.);
#27089=ORIENTED_EDGE('',*,*,#21418,.T.);
#27090=ORIENTED_EDGE('',*,*,#21419,.F.);
#27091=ORIENTED_EDGE('',*,*,#20884,.T.);
#27092=ORIENTED_EDGE('',*,*,#21420,.T.);
#27093=ORIENTED_EDGE('',*,*,#21421,.T.);
#27094=ORIENTED_EDGE('',*,*,#21422,.F.);
#27095=ORIENTED_EDGE('',*,*,#20880,.T.);
#27096=ORIENTED_EDGE('',*,*,#21423,.T.);
#27097=ORIENTED_EDGE('',*,*,#21424,.T.);
#27098=ORIENTED_EDGE('',*,*,#21425,.F.);
#27099=ORIENTED_EDGE('',*,*,#20876,.F.);
#27100=ORIENTED_EDGE('',*,*,#21426,.F.);
#27101=ORIENTED_EDGE('',*,*,#21427,.F.);
#27102=ORIENTED_EDGE('',*,*,#21428,.T.);
#27103=ORIENTED_EDGE('',*,*,#20900,.F.);
#27104=ORIENTED_EDGE('',*,*,#21429,.F.);
#27105=ORIENTED_EDGE('',*,*,#21430,.F.);
#27106=ORIENTED_EDGE('',*,*,#21431,.T.);
#27107=ORIENTED_EDGE('',*,*,#20904,.F.);
#27108=ORIENTED_EDGE('',*,*,#21432,.F.);
#27109=ORIENTED_EDGE('',*,*,#21433,.F.);
#27110=ORIENTED_EDGE('',*,*,#21434,.T.);
#27111=ORIENTED_EDGE('',*,*,#20908,.F.);
#27112=ORIENTED_EDGE('',*,*,#21435,.F.);
#27113=ORIENTED_EDGE('',*,*,#21436,.F.);
#27114=ORIENTED_EDGE('',*,*,#21437,.T.);
#27115=ORIENTED_EDGE('',*,*,#20912,.F.);
#27116=ORIENTED_EDGE('',*,*,#21438,.F.);
#27117=ORIENTED_EDGE('',*,*,#21439,.F.);
#27118=ORIENTED_EDGE('',*,*,#21440,.T.);
#27119=ORIENTED_EDGE('',*,*,#20916,.F.);
#27120=ORIENTED_EDGE('',*,*,#21441,.F.);
#27121=ORIENTED_EDGE('',*,*,#21442,.F.);
#27122=ORIENTED_EDGE('',*,*,#21443,.T.);
#27123=ORIENTED_EDGE('',*,*,#20920,.F.);
#27124=ORIENTED_EDGE('',*,*,#21444,.F.);
#27125=ORIENTED_EDGE('',*,*,#21445,.F.);
#27126=ORIENTED_EDGE('',*,*,#21446,.T.);
#27127=ORIENTED_EDGE('',*,*,#20924,.F.);
#27128=ORIENTED_EDGE('',*,*,#21447,.F.);
#27129=ORIENTED_EDGE('',*,*,#21448,.F.);
#27130=ORIENTED_EDGE('',*,*,#21449,.T.);
#27131=ORIENTED_EDGE('',*,*,#20944,.F.);
#27132=ORIENTED_EDGE('',*,*,#21450,.F.);
#27133=ORIENTED_EDGE('',*,*,#21451,.F.);
#27134=ORIENTED_EDGE('',*,*,#21452,.T.);
#27135=ORIENTED_EDGE('',*,*,#20948,.F.);
#27136=ORIENTED_EDGE('',*,*,#21453,.F.);
#27137=ORIENTED_EDGE('',*,*,#21454,.F.);
#27138=ORIENTED_EDGE('',*,*,#21455,.T.);
#27139=ORIENTED_EDGE('',*,*,#20956,.F.);
#27140=ORIENTED_EDGE('',*,*,#21456,.F.);
#27141=ORIENTED_EDGE('',*,*,#21457,.F.);
#27142=ORIENTED_EDGE('',*,*,#21458,.T.);
#27143=ORIENTED_EDGE('',*,*,#20968,.F.);
#27144=ORIENTED_EDGE('',*,*,#21459,.F.);
#27145=ORIENTED_EDGE('',*,*,#21460,.F.);
#27146=ORIENTED_EDGE('',*,*,#21461,.T.);
#27147=ORIENTED_EDGE('',*,*,#21462,.F.);
#27148=ORIENTED_EDGE('',*,*,#20976,.F.);
#27149=ORIENTED_EDGE('',*,*,#21463,.T.);
#27150=ORIENTED_EDGE('',*,*,#21464,.F.);
#27151=ORIENTED_EDGE('',*,*,#21465,.F.);
#27152=ORIENTED_EDGE('',*,*,#20980,.F.);
#27153=ORIENTED_EDGE('',*,*,#21466,.T.);
#27154=ORIENTED_EDGE('',*,*,#21467,.F.);
#27155=ORIENTED_EDGE('',*,*,#21468,.F.);
#27156=ORIENTED_EDGE('',*,*,#20984,.F.);
#27157=ORIENTED_EDGE('',*,*,#21469,.T.);
#27158=ORIENTED_EDGE('',*,*,#21470,.F.);
#27159=ORIENTED_EDGE('',*,*,#21471,.F.);
#27160=ORIENTED_EDGE('',*,*,#20988,.F.);
#27161=ORIENTED_EDGE('',*,*,#21472,.T.);
#27162=ORIENTED_EDGE('',*,*,#21473,.F.);
#27163=ORIENTED_EDGE('',*,*,#21474,.F.);
#27164=ORIENTED_EDGE('',*,*,#20992,.F.);
#27165=ORIENTED_EDGE('',*,*,#21475,.T.);
#27166=ORIENTED_EDGE('',*,*,#21476,.F.);
#27167=ORIENTED_EDGE('',*,*,#21477,.F.);
#27168=ORIENTED_EDGE('',*,*,#21024,.F.);
#27169=ORIENTED_EDGE('',*,*,#21478,.T.);
#27170=ORIENTED_EDGE('',*,*,#21479,.F.);
#27171=ORIENTED_EDGE('',*,*,#21480,.F.);
#27172=ORIENTED_EDGE('',*,*,#21028,.F.);
#27173=ORIENTED_EDGE('',*,*,#21481,.T.);
#27174=ORIENTED_EDGE('',*,*,#21482,.F.);
#27175=ORIENTED_EDGE('',*,*,#21483,.F.);
#27176=ORIENTED_EDGE('',*,*,#21032,.F.);
#27177=ORIENTED_EDGE('',*,*,#21484,.T.);
#27178=ORIENTED_EDGE('',*,*,#21485,.F.);
#27179=ORIENTED_EDGE('',*,*,#21486,.F.);
#27180=ORIENTED_EDGE('',*,*,#21036,.F.);
#27181=ORIENTED_EDGE('',*,*,#21487,.T.);
#27182=ORIENTED_EDGE('',*,*,#21488,.F.);
#27183=ORIENTED_EDGE('',*,*,#21489,.F.);
#27184=ORIENTED_EDGE('',*,*,#21048,.F.);
#27185=ORIENTED_EDGE('',*,*,#21490,.T.);
#27186=ORIENTED_EDGE('',*,*,#21491,.F.);
#27187=ORIENTED_EDGE('',*,*,#21492,.F.);
#27188=ORIENTED_EDGE('',*,*,#21056,.F.);
#27189=ORIENTED_EDGE('',*,*,#21493,.T.);
#27190=ORIENTED_EDGE('',*,*,#21494,.F.);
#27191=ORIENTED_EDGE('',*,*,#21495,.F.);
#27192=ORIENTED_EDGE('',*,*,#21060,.F.);
#27193=ORIENTED_EDGE('',*,*,#21496,.T.);
#27194=ORIENTED_EDGE('',*,*,#21497,.F.);
#27195=ORIENTED_EDGE('',*,*,#21498,.T.);
#27196=ORIENTED_EDGE('',*,*,#21499,.T.);
#27197=ORIENTED_EDGE('',*,*,#21500,.T.);
#27198=ORIENTED_EDGE('',*,*,#21501,.F.);
#27199=ORIENTED_EDGE('',*,*,#21502,.T.);
#27200=ORIENTED_EDGE('',*,*,#21503,.F.);
#27201=ORIENTED_EDGE('',*,*,#21504,.F.);
#27202=ORIENTED_EDGE('',*,*,#21505,.F.);
#27203=ORIENTED_EDGE('',*,*,#21506,.F.);
#27204=ORIENTED_EDGE('',*,*,#21507,.T.);
#27205=ORIENTED_EDGE('',*,*,#21058,.T.);
#27206=ORIENTED_EDGE('',*,*,#21508,.T.);
#27207=ORIENTED_EDGE('',*,*,#21509,.T.);
#27208=ORIENTED_EDGE('',*,*,#21510,.F.);
#27209=ORIENTED_EDGE('',*,*,#21054,.T.);
#27210=ORIENTED_EDGE('',*,*,#21511,.T.);
#27211=ORIENTED_EDGE('',*,*,#21512,.T.);
#27212=ORIENTED_EDGE('',*,*,#21513,.F.);
#27213=ORIENTED_EDGE('',*,*,#21050,.F.);
#27214=ORIENTED_EDGE('',*,*,#21514,.F.);
#27215=ORIENTED_EDGE('',*,*,#21515,.F.);
#27216=ORIENTED_EDGE('',*,*,#21516,.T.);
#27217=ORIENTED_EDGE('',*,*,#21038,.F.);
#27218=ORIENTED_EDGE('',*,*,#21517,.F.);
#27219=ORIENTED_EDGE('',*,*,#21518,.F.);
#27220=ORIENTED_EDGE('',*,*,#21519,.T.);
#27221=ORIENTED_EDGE('',*,*,#21014,.F.);
#27222=ORIENTED_EDGE('',*,*,#21520,.F.);
#27223=ORIENTED_EDGE('',*,*,#21521,.F.);
#27224=ORIENTED_EDGE('',*,*,#21522,.T.);
#27225=ORIENTED_EDGE('',*,*,#21006,.F.);
#27226=ORIENTED_EDGE('',*,*,#21523,.F.);
#27227=ORIENTED_EDGE('',*,*,#21524,.F.);
#27228=ORIENTED_EDGE('',*,*,#21525,.T.);
#27229=ORIENTED_EDGE('',*,*,#20998,.F.);
#27230=ORIENTED_EDGE('',*,*,#21526,.F.);
#27231=ORIENTED_EDGE('',*,*,#21527,.F.);
#27232=ORIENTED_EDGE('',*,*,#21528,.T.);
#27233=ORIENTED_EDGE('',*,*,#20990,.T.);
#27234=ORIENTED_EDGE('',*,*,#21529,.T.);
#27235=ORIENTED_EDGE('',*,*,#21530,.T.);
#27236=ORIENTED_EDGE('',*,*,#21531,.F.);
#27237=ORIENTED_EDGE('',*,*,#20986,.T.);
#27238=ORIENTED_EDGE('',*,*,#21532,.T.);
#27239=ORIENTED_EDGE('',*,*,#21533,.T.);
#27240=ORIENTED_EDGE('',*,*,#21534,.F.);
#27241=ORIENTED_EDGE('',*,*,#20982,.T.);
#27242=ORIENTED_EDGE('',*,*,#21535,.T.);
#27243=ORIENTED_EDGE('',*,*,#21536,.T.);
#27244=ORIENTED_EDGE('',*,*,#21537,.F.);
#27245=ORIENTED_EDGE('',*,*,#20978,.T.);
#27246=ORIENTED_EDGE('',*,*,#21538,.T.);
#27247=ORIENTED_EDGE('',*,*,#21539,.T.);
#27248=ORIENTED_EDGE('',*,*,#21540,.F.);
#27249=ORIENTED_EDGE('',*,*,#20974,.T.);
#27250=ORIENTED_EDGE('',*,*,#21541,.T.);
#27251=ORIENTED_EDGE('',*,*,#21542,.T.);
#27252=ORIENTED_EDGE('',*,*,#21543,.F.);
#27253=ORIENTED_EDGE('',*,*,#20970,.F.);
#27254=ORIENTED_EDGE('',*,*,#21544,.F.);
#27255=ORIENTED_EDGE('',*,*,#21545,.F.);
#27256=ORIENTED_EDGE('',*,*,#21546,.T.);
#27257=ORIENTED_EDGE('',*,*,#21547,.F.);
#27258=ORIENTED_EDGE('',*,*,#20958,.F.);
#27259=ORIENTED_EDGE('',*,*,#21548,.T.);
#27260=ORIENTED_EDGE('',*,*,#21549,.F.);
#27261=ORIENTED_EDGE('',*,*,#21550,.T.);
#27262=ORIENTED_EDGE('',*,*,#20946,.T.);
#27263=ORIENTED_EDGE('',*,*,#21551,.F.);
#27264=ORIENTED_EDGE('',*,*,#21552,.T.);
#27265=ORIENTED_EDGE('',*,*,#21553,.T.);
#27266=ORIENTED_EDGE('',*,*,#20942,.T.);
#27267=ORIENTED_EDGE('',*,*,#21554,.F.);
#27268=ORIENTED_EDGE('',*,*,#21555,.T.);
#27269=ORIENTED_EDGE('',*,*,#21556,.F.);
#27270=ORIENTED_EDGE('',*,*,#20938,.F.);
#27271=ORIENTED_EDGE('',*,*,#21557,.T.);
#27272=ORIENTED_EDGE('',*,*,#21558,.F.);
#27273=ORIENTED_EDGE('',*,*,#21559,.F.);
#27274=ORIENTED_EDGE('',*,*,#20930,.F.);
#27275=ORIENTED_EDGE('',*,*,#21560,.T.);
#27276=ORIENTED_EDGE('',*,*,#21561,.F.);
#27277=ORIENTED_EDGE('',*,*,#21562,.T.);
#27278=ORIENTED_EDGE('',*,*,#20922,.T.);
#27279=ORIENTED_EDGE('',*,*,#21563,.F.);
#27280=ORIENTED_EDGE('',*,*,#21564,.T.);
#27281=ORIENTED_EDGE('',*,*,#21565,.T.);
#27282=ORIENTED_EDGE('',*,*,#20918,.T.);
#27283=ORIENTED_EDGE('',*,*,#21566,.F.);
#27284=ORIENTED_EDGE('',*,*,#21567,.T.);
#27285=ORIENTED_EDGE('',*,*,#21568,.T.);
#27286=ORIENTED_EDGE('',*,*,#20914,.T.);
#27287=ORIENTED_EDGE('',*,*,#21569,.F.);
#27288=ORIENTED_EDGE('',*,*,#21570,.T.);
#27289=ORIENTED_EDGE('',*,*,#21571,.T.);
#27290=ORIENTED_EDGE('',*,*,#20910,.T.);
#27291=ORIENTED_EDGE('',*,*,#21572,.F.);
#27292=ORIENTED_EDGE('',*,*,#21573,.T.);
#27293=ORIENTED_EDGE('',*,*,#21574,.T.);
#27294=ORIENTED_EDGE('',*,*,#20906,.T.);
#27295=ORIENTED_EDGE('',*,*,#21575,.F.);
#27296=ORIENTED_EDGE('',*,*,#21576,.T.);
#27297=ORIENTED_EDGE('',*,*,#21577,.T.);
#27298=ORIENTED_EDGE('',*,*,#20902,.T.);
#27299=ORIENTED_EDGE('',*,*,#21578,.F.);
#27300=ORIENTED_EDGE('',*,*,#21579,.T.);
#27301=ORIENTED_EDGE('',*,*,#21580,.T.);
#27302=ORIENTED_EDGE('',*,*,#20898,.T.);
#27303=ORIENTED_EDGE('',*,*,#21581,.F.);
#27304=ORIENTED_EDGE('',*,*,#21582,.T.);
#27305=ORIENTED_EDGE('',*,*,#21583,.F.);
#27306=ORIENTED_EDGE('',*,*,#20894,.F.);
#27307=ORIENTED_EDGE('',*,*,#21584,.T.);
#27308=ORIENTED_EDGE('',*,*,#21585,.F.);
#27309=ORIENTED_EDGE('',*,*,#21586,.F.);
#27310=ORIENTED_EDGE('',*,*,#20886,.F.);
#27311=ORIENTED_EDGE('',*,*,#21587,.T.);
#27312=ORIENTED_EDGE('',*,*,#21588,.F.);
#27313=ORIENTED_EDGE('',*,*,#21589,.F.);
#27314=ORIENTED_EDGE('',*,*,#20878,.F.);
#27315=ORIENTED_EDGE('',*,*,#21590,.T.);
#27316=ORIENTED_EDGE('',*,*,#21591,.F.);
#27317=ORIENTED_EDGE('',*,*,#21592,.T.);
#27318=ORIENTED_EDGE('',*,*,#20874,.T.);
#27319=ORIENTED_EDGE('',*,*,#21593,.F.);
#27320=ORIENTED_EDGE('',*,*,#21594,.T.);
#27321=ORIENTED_EDGE('',*,*,#21595,.F.);
#27322=ORIENTED_EDGE('',*,*,#20882,.F.);
#27323=ORIENTED_EDGE('',*,*,#21596,.T.);
#27324=ORIENTED_EDGE('',*,*,#21597,.F.);
#27325=ORIENTED_EDGE('',*,*,#21598,.F.);
#27326=ORIENTED_EDGE('',*,*,#20890,.F.);
#27327=ORIENTED_EDGE('',*,*,#21599,.T.);
#27328=ORIENTED_EDGE('',*,*,#21600,.F.);
#27329=ORIENTED_EDGE('',*,*,#21601,.F.);
#27330=ORIENTED_EDGE('',*,*,#20926,.F.);
#27331=ORIENTED_EDGE('',*,*,#21602,.T.);
#27332=ORIENTED_EDGE('',*,*,#21603,.F.);
#27333=ORIENTED_EDGE('',*,*,#21604,.F.);
#27334=ORIENTED_EDGE('',*,*,#20934,.F.);
#27335=ORIENTED_EDGE('',*,*,#21605,.T.);
#27336=ORIENTED_EDGE('',*,*,#21606,.F.);
#27337=ORIENTED_EDGE('',*,*,#21607,.F.);
#27338=ORIENTED_EDGE('',*,*,#20950,.F.);
#27339=ORIENTED_EDGE('',*,*,#21608,.T.);
#27340=ORIENTED_EDGE('',*,*,#21609,.F.);
#27341=ORIENTED_EDGE('',*,*,#21610,.T.);
#27342=ORIENTED_EDGE('',*,*,#20954,.T.);
#27343=ORIENTED_EDGE('',*,*,#21611,.F.);
#27344=ORIENTED_EDGE('',*,*,#21612,.T.);
#27345=ORIENTED_EDGE('',*,*,#21613,.F.);
#27346=ORIENTED_EDGE('',*,*,#20962,.F.);
#27347=ORIENTED_EDGE('',*,*,#21614,.T.);
#27348=ORIENTED_EDGE('',*,*,#21615,.F.);
#27349=ORIENTED_EDGE('',*,*,#21616,.T.);
#27350=ORIENTED_EDGE('',*,*,#20966,.T.);
#27351=ORIENTED_EDGE('',*,*,#21617,.F.);
#27352=ORIENTED_EDGE('',*,*,#21618,.T.);
#27353=ORIENTED_EDGE('',*,*,#20994,.F.);
#27354=ORIENTED_EDGE('',*,*,#21619,.F.);
#27355=ORIENTED_EDGE('',*,*,#21620,.F.);
#27356=ORIENTED_EDGE('',*,*,#21621,.T.);
#27357=ORIENTED_EDGE('',*,*,#21002,.F.);
#27358=ORIENTED_EDGE('',*,*,#21622,.F.);
#27359=ORIENTED_EDGE('',*,*,#21623,.F.);
#27360=ORIENTED_EDGE('',*,*,#21624,.T.);
#27361=ORIENTED_EDGE('',*,*,#21010,.F.);
#27362=ORIENTED_EDGE('',*,*,#21625,.F.);
#27363=ORIENTED_EDGE('',*,*,#21626,.F.);
#27364=ORIENTED_EDGE('',*,*,#21627,.T.);
#27365=ORIENTED_EDGE('',*,*,#21018,.F.);
#27366=ORIENTED_EDGE('',*,*,#21628,.F.);
#27367=ORIENTED_EDGE('',*,*,#21629,.F.);
#27368=ORIENTED_EDGE('',*,*,#21630,.T.);
#27369=ORIENTED_EDGE('',*,*,#21022,.T.);
#27370=ORIENTED_EDGE('',*,*,#21631,.T.);
#27371=ORIENTED_EDGE('',*,*,#21632,.T.);
#27372=ORIENTED_EDGE('',*,*,#21633,.F.);
#27373=ORIENTED_EDGE('',*,*,#21026,.T.);
#27374=ORIENTED_EDGE('',*,*,#21634,.T.);
#27375=ORIENTED_EDGE('',*,*,#21635,.T.);
#27376=ORIENTED_EDGE('',*,*,#21636,.F.);
#27377=ORIENTED_EDGE('',*,*,#21030,.T.);
#27378=ORIENTED_EDGE('',*,*,#21637,.T.);
#27379=ORIENTED_EDGE('',*,*,#21638,.T.);
#27380=ORIENTED_EDGE('',*,*,#21639,.F.);
#27381=ORIENTED_EDGE('',*,*,#21034,.T.);
#27382=ORIENTED_EDGE('',*,*,#21640,.T.);
#27383=ORIENTED_EDGE('',*,*,#21641,.T.);
#27384=ORIENTED_EDGE('',*,*,#21642,.F.);
#27385=ORIENTED_EDGE('',*,*,#21042,.F.);
#27386=ORIENTED_EDGE('',*,*,#21643,.F.);
#27387=ORIENTED_EDGE('',*,*,#21644,.F.);
#27388=ORIENTED_EDGE('',*,*,#21645,.T.);
#27389=ORIENTED_EDGE('',*,*,#21046,.T.);
#27390=ORIENTED_EDGE('',*,*,#21646,.T.);
#27391=ORIENTED_EDGE('',*,*,#21647,.T.);
#27392=ORIENTED_EDGE('',*,*,#21648,.F.);
#27393=ORIENTED_EDGE('',*,*,#21062,.F.);
#27394=ORIENTED_EDGE('',*,*,#21649,.F.);
#27395=ORIENTED_EDGE('',*,*,#21650,.F.);
#27396=ORIENTED_EDGE('',*,*,#21651,.T.);
#27397=ORIENTED_EDGE('',*,*,#21652,.F.);
#27398=ORIENTED_EDGE('',*,*,#21111,.T.);
#27399=ORIENTED_EDGE('',*,*,#21653,.F.);
#27400=ORIENTED_EDGE('',*,*,#21654,.T.);
#27401=ORIENTED_EDGE('',*,*,#21655,.F.);
#27402=ORIENTED_EDGE('',*,*,#21656,.T.);
#27403=ORIENTED_EDGE('',*,*,#21657,.F.);
#27404=ORIENTED_EDGE('',*,*,#21095,.T.);
#27405=ORIENTED_EDGE('',*,*,#21658,.F.);
#27406=ORIENTED_EDGE('',*,*,#21659,.T.);
#27407=ORIENTED_EDGE('',*,*,#21660,.F.);
#27408=ORIENTED_EDGE('',*,*,#21661,.T.);
#27409=ORIENTED_EDGE('',*,*,#21662,.F.);
#27410=ORIENTED_EDGE('',*,*,#21109,.T.);
#27411=ORIENTED_EDGE('',*,*,#21663,.F.);
#27412=ORIENTED_EDGE('',*,*,#21664,.T.);
#27413=ORIENTED_EDGE('',*,*,#21665,.F.);
#27414=ORIENTED_EDGE('',*,*,#21666,.T.);
#27415=ORIENTED_EDGE('',*,*,#21667,.F.);
#27416=ORIENTED_EDGE('',*,*,#21668,.T.);
#27417=ORIENTED_EDGE('',*,*,#21669,.F.);
#27418=ORIENTED_EDGE('',*,*,#21105,.T.);
#27419=ORIENTED_EDGE('',*,*,#21670,.F.);
#27420=ORIENTED_EDGE('',*,*,#21671,.T.);
#27421=ORIENTED_EDGE('',*,*,#21672,.F.);
#27422=ORIENTED_EDGE('',*,*,#21099,.T.);
#27423=ORIENTED_EDGE('',*,*,#21673,.F.);
#27424=ORIENTED_EDGE('',*,*,#21674,.T.);
#27425=ORIENTED_EDGE('',*,*,#21675,.F.);
#27426=ORIENTED_EDGE('',*,*,#21676,.T.);
#27427=ORIENTED_EDGE('',*,*,#21677,.F.);
#27428=ORIENTED_EDGE('',*,*,#21678,.T.);
#27429=ORIENTED_EDGE('',*,*,#21679,.F.);
#27430=ORIENTED_EDGE('',*,*,#21680,.T.);
#27431=ORIENTED_EDGE('',*,*,#21681,.F.);
#27432=ORIENTED_EDGE('',*,*,#21682,.T.);
#27433=ORIENTED_EDGE('',*,*,#21683,.F.);
#27434=ORIENTED_EDGE('',*,*,#21684,.T.);
#27435=ORIENTED_EDGE('',*,*,#21685,.F.);
#27436=ORIENTED_EDGE('',*,*,#21093,.T.);
#27437=ORIENTED_EDGE('',*,*,#21686,.F.);
#27438=ORIENTED_EDGE('',*,*,#21687,.T.);
#27439=ORIENTED_EDGE('',*,*,#21688,.F.);
#27440=ORIENTED_EDGE('',*,*,#21689,.T.);
#27441=ORIENTED_EDGE('',*,*,#21690,.F.);
#27442=ORIENTED_EDGE('',*,*,#21691,.T.);
#27443=ORIENTED_EDGE('',*,*,#21692,.F.);
#27444=ORIENTED_EDGE('',*,*,#21693,.T.);
#27445=ORIENTED_EDGE('',*,*,#21694,.F.);
#27446=ORIENTED_EDGE('',*,*,#21123,.T.);
#27447=ORIENTED_EDGE('',*,*,#21695,.F.);
#27448=ORIENTED_EDGE('',*,*,#21696,.T.);
#27449=ORIENTED_EDGE('',*,*,#21697,.F.);
#27450=ORIENTED_EDGE('',*,*,#21698,.T.);
#27451=ORIENTED_EDGE('',*,*,#21699,.F.);
#27452=ORIENTED_EDGE('',*,*,#21119,.T.);
#27453=ORIENTED_EDGE('',*,*,#21700,.F.);
#27454=ORIENTED_EDGE('',*,*,#21701,.T.);
#27455=ORIENTED_EDGE('',*,*,#21702,.F.);
#27456=ORIENTED_EDGE('',*,*,#21703,.T.);
#27457=ORIENTED_EDGE('',*,*,#21704,.F.);
#27458=ORIENTED_EDGE('',*,*,#21137,.T.);
#27459=ORIENTED_EDGE('',*,*,#21705,.F.);
#27460=ORIENTED_EDGE('',*,*,#21706,.T.);
#27461=ORIENTED_EDGE('',*,*,#21707,.F.);
#27462=ORIENTED_EDGE('',*,*,#21708,.T.);
#27463=ORIENTED_EDGE('',*,*,#21709,.F.);
#27464=ORIENTED_EDGE('',*,*,#21710,.T.);
#27465=ORIENTED_EDGE('',*,*,#21711,.F.);
#27466=ORIENTED_EDGE('',*,*,#21133,.T.);
#27467=ORIENTED_EDGE('',*,*,#21712,.F.);
#27468=ORIENTED_EDGE('',*,*,#21713,.T.);
#27469=ORIENTED_EDGE('',*,*,#21714,.F.);
#27470=ORIENTED_EDGE('',*,*,#21127,.T.);
#27471=ORIENTED_EDGE('',*,*,#21715,.F.);
#27472=ORIENTED_EDGE('',*,*,#21716,.T.);
#27473=ORIENTED_EDGE('',*,*,#21717,.F.);
#27474=ORIENTED_EDGE('',*,*,#21718,.T.);
#27475=ORIENTED_EDGE('',*,*,#21719,.F.);
#27476=ORIENTED_EDGE('',*,*,#21720,.T.);
#27477=ORIENTED_EDGE('',*,*,#21721,.F.);
#27478=ORIENTED_EDGE('',*,*,#21722,.T.);
#27479=ORIENTED_EDGE('',*,*,#21723,.F.);
#27480=ORIENTED_EDGE('',*,*,#21724,.T.);
#27481=ORIENTED_EDGE('',*,*,#21725,.F.);
#27482=ORIENTED_EDGE('',*,*,#21726,.T.);
#27483=ORIENTED_EDGE('',*,*,#21727,.F.);
#27484=ORIENTED_EDGE('',*,*,#21117,.T.);
#27485=ORIENTED_EDGE('',*,*,#21728,.F.);
#27486=ORIENTED_EDGE('',*,*,#21729,.T.);
#27487=ORIENTED_EDGE('',*,*,#21730,.F.);
#27488=ORIENTED_EDGE('',*,*,#21731,.T.);
#27489=ORIENTED_EDGE('',*,*,#21732,.F.);
#27490=ORIENTED_EDGE('',*,*,#21733,.T.);
#27491=ORIENTED_EDGE('',*,*,#21734,.F.);
#27492=ORIENTED_EDGE('',*,*,#21735,.T.);
#27493=ORIENTED_EDGE('',*,*,#21736,.T.);
#27494=ORIENTED_EDGE('',*,*,#21737,.T.);
#27495=ORIENTED_EDGE('',*,*,#21738,.F.);
#27496=ORIENTED_EDGE('',*,*,#21739,.T.);
#27497=ORIENTED_EDGE('',*,*,#21172,.F.);
#27498=ORIENTED_EDGE('',*,*,#21154,.F.);
#27499=ORIENTED_EDGE('',*,*,#21740,.T.);
#27500=ORIENTED_EDGE('',*,*,#21679,.T.);
#27501=ORIENTED_EDGE('',*,*,#21741,.T.);
#27502=ORIENTED_EDGE('',*,*,#21742,.T.);
#27503=ORIENTED_EDGE('',*,*,#21142,.T.);
#27504=ORIENTED_EDGE('',*,*,#21743,.T.);
#27505=ORIENTED_EDGE('',*,*,#21653,.T.);
#27506=ORIENTED_EDGE('',*,*,#21110,.T.);
#27507=ORIENTED_EDGE('',*,*,#21744,.F.);
#27508=ORIENTED_EDGE('',*,*,#21146,.F.);
#27509=ORIENTED_EDGE('',*,*,#21745,.T.);
#27510=ORIENTED_EDGE('',*,*,#21746,.T.);
#27511=ORIENTED_EDGE('',*,*,#21747,.T.);
#27512=ORIENTED_EDGE('',*,*,#21748,.T.);
#27513=ORIENTED_EDGE('',*,*,#21138,.T.);
#27514=ORIENTED_EDGE('',*,*,#21749,.T.);
#27515=ORIENTED_EDGE('',*,*,#21750,.T.);
#27516=ORIENTED_EDGE('',*,*,#21086,.T.);
#27517=ORIENTED_EDGE('',*,*,#21751,.F.);
#27518=ORIENTED_EDGE('',*,*,#21752,.T.);
#27519=ORIENTED_EDGE('',*,*,#21753,.T.);
#27520=ORIENTED_EDGE('',*,*,#21754,.T.);
#27521=ORIENTED_EDGE('',*,*,#21066,.T.);
#27522=ORIENTED_EDGE('',*,*,#21755,.T.);
#27523=ORIENTED_EDGE('',*,*,#21756,.T.);
#27524=ORIENTED_EDGE('',*,*,#21757,.F.);
#27525=ORIENTED_EDGE('',*,*,#21758,.T.);
#27526=ORIENTED_EDGE('',*,*,#21759,.T.);
#27527=ORIENTED_EDGE('',*,*,#21070,.T.);
#27528=ORIENTED_EDGE('',*,*,#21760,.T.);
#27529=ORIENTED_EDGE('',*,*,#21761,.T.);
#27530=ORIENTED_EDGE('',*,*,#21762,.T.);
#27531=ORIENTED_EDGE('',*,*,#21763,.T.);
#27532=ORIENTED_EDGE('',*,*,#21764,.F.);
#27533=ORIENTED_EDGE('',*,*,#21765,.T.);
#27534=ORIENTED_EDGE('',*,*,#21766,.T.);
#27535=ORIENTED_EDGE('',*,*,#21767,.T.);
#27536=ORIENTED_EDGE('',*,*,#21768,.T.);
#27537=ORIENTED_EDGE('',*,*,#21769,.T.);
#27538=ORIENTED_EDGE('',*,*,#21770,.T.);
#27539=ORIENTED_EDGE('',*,*,#21771,.T.);
#27540=ORIENTED_EDGE('',*,*,#21772,.F.);
#27541=ORIENTED_EDGE('',*,*,#21082,.T.);
#27542=ORIENTED_EDGE('',*,*,#21773,.T.);
#27543=ORIENTED_EDGE('',*,*,#21774,.T.);
#27544=ORIENTED_EDGE('',*,*,#21775,.T.);
#27545=ORIENTED_EDGE('',*,*,#21776,.T.);
#27546=ORIENTED_EDGE('',*,*,#21777,.T.);
#27547=ORIENTED_EDGE('',*,*,#21778,.T.);
#27548=ORIENTED_EDGE('',*,*,#21779,.F.);
#27549=ORIENTED_EDGE('',*,*,#21078,.T.);
#27550=ORIENTED_EDGE('',*,*,#21780,.T.);
#27551=ORIENTED_EDGE('',*,*,#21781,.T.);
#27552=ORIENTED_EDGE('',*,*,#21782,.T.);
#27553=ORIENTED_EDGE('',*,*,#21783,.T.);
#27554=ORIENTED_EDGE('',*,*,#21784,.T.);
#27555=ORIENTED_EDGE('',*,*,#21074,.T.);
#27556=ORIENTED_EDGE('',*,*,#21785,.F.);
#27557=ORIENTED_EDGE('',*,*,#21786,.T.);
#27558=ORIENTED_EDGE('',*,*,#21686,.T.);
#27559=ORIENTED_EDGE('',*,*,#21787,.T.);
#27560=ORIENTED_EDGE('',*,*,#21788,.T.);
#27561=ORIENTED_EDGE('',*,*,#21090,.T.);
#27562=ORIENTED_EDGE('',*,*,#21685,.T.);
#27563=ORIENTED_EDGE('',*,*,#21789,.T.);
#27564=ORIENTED_EDGE('',*,*,#21790,.F.);
#27565=ORIENTED_EDGE('',*,*,#21791,.T.);
#27566=ORIENTED_EDGE('',*,*,#21655,.T.);
#27567=ORIENTED_EDGE('',*,*,#21094,.T.);
#27568=ORIENTED_EDGE('',*,*,#21792,.T.);
#27569=ORIENTED_EDGE('',*,*,#21793,.T.);
#27570=ORIENTED_EDGE('',*,*,#21690,.T.);
#27571=ORIENTED_EDGE('',*,*,#21794,.T.);
#27572=ORIENTED_EDGE('',*,*,#21795,.F.);
#27573=ORIENTED_EDGE('',*,*,#21796,.T.);
#27574=ORIENTED_EDGE('',*,*,#21662,.T.);
#27575=ORIENTED_EDGE('',*,*,#21797,.T.);
#27576=ORIENTED_EDGE('',*,*,#21798,.T.);
#27577=ORIENTED_EDGE('',*,*,#21799,.T.);
#27578=ORIENTED_EDGE('',*,*,#21660,.T.);
#27579=ORIENTED_EDGE('',*,*,#21800,.T.);
#27580=ORIENTED_EDGE('',*,*,#21801,.F.);
#27581=ORIENTED_EDGE('',*,*,#21106,.T.);
#27582=ORIENTED_EDGE('',*,*,#21669,.T.);
#27583=ORIENTED_EDGE('',*,*,#21802,.T.);
#27584=ORIENTED_EDGE('',*,*,#21803,.T.);
#27585=ORIENTED_EDGE('',*,*,#21804,.T.);
#27586=ORIENTED_EDGE('',*,*,#21667,.T.);
#27587=ORIENTED_EDGE('',*,*,#21805,.T.);
#27588=ORIENTED_EDGE('',*,*,#21806,.F.);
#27589=ORIENTED_EDGE('',*,*,#21102,.T.);
#27590=ORIENTED_EDGE('',*,*,#21675,.T.);
#27591=ORIENTED_EDGE('',*,*,#21807,.T.);
#27592=ORIENTED_EDGE('',*,*,#21808,.T.);
#27593=ORIENTED_EDGE('',*,*,#21809,.T.);
#27594=ORIENTED_EDGE('',*,*,#21673,.T.);
#27595=ORIENTED_EDGE('',*,*,#21098,.T.);
#27596=ORIENTED_EDGE('',*,*,#21810,.F.);
#27597=ORIENTED_EDGE('',*,*,#21811,.T.);
#27598=ORIENTED_EDGE('',*,*,#21728,.T.);
#27599=ORIENTED_EDGE('',*,*,#21812,.T.);
#27600=ORIENTED_EDGE('',*,*,#21813,.T.);
#27601=ORIENTED_EDGE('',*,*,#21114,.T.);
#27602=ORIENTED_EDGE('',*,*,#21727,.T.);
#27603=ORIENTED_EDGE('',*,*,#21814,.T.);
#27604=ORIENTED_EDGE('',*,*,#21736,.F.);
#27605=ORIENTED_EDGE('',*,*,#21815,.T.);
#27606=ORIENTED_EDGE('',*,*,#21697,.T.);
#27607=ORIENTED_EDGE('',*,*,#21118,.T.);
#27608=ORIENTED_EDGE('',*,*,#21816,.T.);
#27609=ORIENTED_EDGE('',*,*,#21817,.T.);
#27610=ORIENTED_EDGE('',*,*,#21732,.T.);
#27611=ORIENTED_EDGE('',*,*,#21818,.T.);
#27612=ORIENTED_EDGE('',*,*,#21819,.F.);
#27613=ORIENTED_EDGE('',*,*,#21820,.T.);
#27614=ORIENTED_EDGE('',*,*,#21704,.T.);
#27615=ORIENTED_EDGE('',*,*,#21821,.T.);
#27616=ORIENTED_EDGE('',*,*,#21822,.T.);
#27617=ORIENTED_EDGE('',*,*,#21823,.T.);
#27618=ORIENTED_EDGE('',*,*,#21702,.T.);
#27619=ORIENTED_EDGE('',*,*,#21824,.T.);
#27620=ORIENTED_EDGE('',*,*,#21825,.F.);
#27621=ORIENTED_EDGE('',*,*,#21134,.T.);
#27622=ORIENTED_EDGE('',*,*,#21711,.T.);
#27623=ORIENTED_EDGE('',*,*,#21826,.T.);
#27624=ORIENTED_EDGE('',*,*,#21827,.T.);
#27625=ORIENTED_EDGE('',*,*,#21828,.T.);
#27626=ORIENTED_EDGE('',*,*,#21709,.T.);
#27627=ORIENTED_EDGE('',*,*,#21829,.T.);
#27628=ORIENTED_EDGE('',*,*,#21830,.F.);
#27629=ORIENTED_EDGE('',*,*,#21130,.T.);
#27630=ORIENTED_EDGE('',*,*,#21717,.T.);
#27631=ORIENTED_EDGE('',*,*,#21831,.T.);
#27632=ORIENTED_EDGE('',*,*,#21832,.T.);
#27633=ORIENTED_EDGE('',*,*,#21833,.T.);
#27634=ORIENTED_EDGE('',*,*,#21715,.T.);
#27635=ORIENTED_EDGE('',*,*,#21126,.T.);
#27636=ORIENTED_EDGE('',*,*,#21834,.F.);
#27637=ORIENTED_EDGE('',*,*,#21835,.T.);
#27638=ORIENTED_EDGE('',*,*,#21192,.F.);
#27639=ORIENTED_EDGE('',*,*,#21836,.T.);
#27640=ORIENTED_EDGE('',*,*,#21721,.T.);
#27641=ORIENTED_EDGE('',*,*,#21837,.T.);
#27642=ORIENTED_EDGE('',*,*,#21838,.T.);
#27643=ORIENTED_EDGE('',*,*,#21150,.T.);
#27644=ORIENTED_EDGE('',*,*,#21839,.T.);
#27645=ORIENTED_EDGE('',*,*,#21695,.T.);
#27646=ORIENTED_EDGE('',*,*,#21122,.T.);
#27647=ORIENTED_EDGE('',*,*,#21840,.F.);
#27648=ORIENTED_EDGE('',*,*,#21193,.F.);
#27649=ORIENTED_EDGE('',*,*,#21840,.T.);
#27650=ORIENTED_EDGE('',*,*,#21125,.T.);
#27651=ORIENTED_EDGE('',*,*,#21841,.F.);
#27652=ORIENTED_EDGE('',*,*,#21842,.F.);
#27653=ORIENTED_EDGE('',*,*,#21087,.T.);
#27654=ORIENTED_EDGE('',*,*,#21750,.F.);
#27655=ORIENTED_EDGE('',*,*,#21843,.T.);
#27656=ORIENTED_EDGE('',*,*,#21834,.T.);
#27657=ORIENTED_EDGE('',*,*,#21129,.T.);
#27658=ORIENTED_EDGE('',*,*,#21844,.F.);
#27659=ORIENTED_EDGE('',*,*,#21845,.T.);
#27660=ORIENTED_EDGE('',*,*,#21830,.T.);
#27661=ORIENTED_EDGE('',*,*,#21846,.T.);
#27662=ORIENTED_EDGE('',*,*,#21847,.F.);
#27663=ORIENTED_EDGE('',*,*,#21131,.T.);
#27664=ORIENTED_EDGE('',*,*,#21825,.T.);
#27665=ORIENTED_EDGE('',*,*,#21848,.T.);
#27666=ORIENTED_EDGE('',*,*,#21849,.F.);
#27667=ORIENTED_EDGE('',*,*,#21135,.T.);
#27668=ORIENTED_EDGE('',*,*,#21850,.T.);
#27669=ORIENTED_EDGE('',*,*,#21851,.T.);
#27670=ORIENTED_EDGE('',*,*,#21852,.F.);
#27671=ORIENTED_EDGE('',*,*,#21853,.F.);
#27672=ORIENTED_EDGE('',*,*,#21854,.F.);
#27673=ORIENTED_EDGE('',*,*,#21855,.F.);
#27674=ORIENTED_EDGE('',*,*,#21856,.F.);
#27675=ORIENTED_EDGE('',*,*,#21857,.F.);
#27676=ORIENTED_EDGE('',*,*,#21858,.T.);
#27677=ORIENTED_EDGE('',*,*,#21859,.T.);
#27678=ORIENTED_EDGE('',*,*,#21163,.F.);
#27679=ORIENTED_EDGE('',*,*,#21160,.T.);
#27680=ORIENTED_EDGE('',*,*,#20858,.F.);
#27681=ORIENTED_EDGE('',*,*,#20861,.F.);
#27682=ORIENTED_EDGE('',*,*,#20864,.F.);
#27683=ORIENTED_EDGE('',*,*,#20867,.F.);
#27684=ORIENTED_EDGE('',*,*,#21860,.F.);
#27685=ORIENTED_EDGE('',*,*,#21861,.F.);
#27686=ORIENTED_EDGE('',*,*,#21862,.F.);
#27687=ORIENTED_EDGE('',*,*,#21863,.F.);
#27688=ORIENTED_EDGE('',*,*,#21864,.F.);
#27689=ORIENTED_EDGE('',*,*,#21865,.F.);
#27690=ORIENTED_EDGE('',*,*,#21866,.F.);
#27691=ORIENTED_EDGE('',*,*,#21867,.F.);
#27692=ORIENTED_EDGE('',*,*,#21868,.F.);
#27693=ORIENTED_EDGE('',*,*,#21869,.F.);
#27694=ORIENTED_EDGE('',*,*,#21870,.F.);
#27695=ORIENTED_EDGE('',*,*,#21871,.F.);
#27696=ORIENTED_EDGE('',*,*,#21872,.F.);
#27697=ORIENTED_EDGE('',*,*,#21873,.F.);
#27698=ORIENTED_EDGE('',*,*,#21874,.F.);
#27699=ORIENTED_EDGE('',*,*,#21875,.F.);
#27700=ORIENTED_EDGE('',*,*,#21166,.T.);
#27701=ORIENTED_EDGE('',*,*,#21169,.F.);
#27702=ORIENTED_EDGE('',*,*,#21175,.F.);
#27703=ORIENTED_EDGE('',*,*,#21876,.T.);
#27704=ORIENTED_EDGE('',*,*,#21877,.T.);
#27705=ORIENTED_EDGE('',*,*,#21878,.F.);
#27706=ORIENTED_EDGE('',*,*,#21879,.T.);
#27707=ORIENTED_EDGE('',*,*,#21880,.F.);
#27708=ORIENTED_EDGE('',*,*,#21881,.F.);
#27709=ORIENTED_EDGE('',*,*,#21882,.T.);
#27710=ORIENTED_EDGE('',*,*,#21883,.T.);
#27711=ORIENTED_EDGE('',*,*,#21884,.F.);
#27712=ORIENTED_EDGE('',*,*,#21885,.F.);
#27713=ORIENTED_EDGE('',*,*,#21164,.F.);
#27714=ORIENTED_EDGE('',*,*,#21158,.F.);
#27715=ORIENTED_EDGE('',*,*,#20856,.T.);
#27716=ORIENTED_EDGE('',*,*,#20859,.T.);
#27717=ORIENTED_EDGE('',*,*,#20862,.T.);
#27718=ORIENTED_EDGE('',*,*,#20865,.T.);
#27719=ORIENTED_EDGE('',*,*,#21886,.T.);
#27720=ORIENTED_EDGE('',*,*,#21887,.T.);
#27721=ORIENTED_EDGE('',*,*,#21888,.T.);
#27722=ORIENTED_EDGE('',*,*,#21889,.T.);
#27723=ORIENTED_EDGE('',*,*,#21890,.T.);
#27724=ORIENTED_EDGE('',*,*,#21891,.T.);
#27725=ORIENTED_EDGE('',*,*,#21892,.T.);
#27726=ORIENTED_EDGE('',*,*,#21893,.T.);
#27727=ORIENTED_EDGE('',*,*,#21894,.T.);
#27728=ORIENTED_EDGE('',*,*,#21895,.T.);
#27729=ORIENTED_EDGE('',*,*,#21896,.T.);
#27730=ORIENTED_EDGE('',*,*,#21897,.T.);
#27731=ORIENTED_EDGE('',*,*,#21898,.T.);
#27732=ORIENTED_EDGE('',*,*,#21899,.T.);
#27733=ORIENTED_EDGE('',*,*,#21900,.T.);
#27734=ORIENTED_EDGE('',*,*,#21901,.T.);
#27735=ORIENTED_EDGE('',*,*,#21161,.T.);
#27736=ORIENTED_EDGE('',*,*,#21167,.T.);
#27737=ORIENTED_EDGE('',*,*,#21178,.F.);
#27738=ORIENTED_EDGE('',*,*,#21902,.F.);
#27739=ORIENTED_EDGE('',*,*,#21213,.T.);
#27740=ORIENTED_EDGE('',*,*,#21903,.F.);
#27741=ORIENTED_EDGE('',*,*,#21268,.T.);
#27742=ORIENTED_EDGE('',*,*,#21904,.F.);
#27743=ORIENTED_EDGE('',*,*,#21341,.T.);
#27744=ORIENTED_EDGE('',*,*,#21269,.T.);
#27745=ORIENTED_EDGE('',*,*,#21903,.T.);
#27746=ORIENTED_EDGE('',*,*,#21212,.T.);
#27747=ORIENTED_EDGE('',*,*,#21905,.F.);
#27748=ORIENTED_EDGE('',*,*,#21266,.T.);
#27749=ORIENTED_EDGE('',*,*,#21906,.T.);
#27750=ORIENTED_EDGE('',*,*,#21215,.T.);
#27751=ORIENTED_EDGE('',*,*,#21907,.F.);
#27752=ORIENTED_EDGE('',*,*,#21303,.T.);
#27753=ORIENTED_EDGE('',*,*,#21216,.T.);
#27754=ORIENTED_EDGE('',*,*,#21906,.F.);
#27755=ORIENTED_EDGE('',*,*,#21265,.T.);
#27756=ORIENTED_EDGE('',*,*,#21908,.F.);
#27757=ORIENTED_EDGE('',*,*,#21199,.T.);
#27758=ORIENTED_EDGE('',*,*,#21909,.F.);
#27759=ORIENTED_EDGE('',*,*,#21282,.T.);
#27760=ORIENTED_EDGE('',*,*,#21910,.F.);
#27761=ORIENTED_EDGE('',*,*,#21301,.T.);
#27762=ORIENTED_EDGE('',*,*,#21283,.T.);
#27763=ORIENTED_EDGE('',*,*,#21909,.T.);
#27764=ORIENTED_EDGE('',*,*,#21198,.T.);
#27765=ORIENTED_EDGE('',*,*,#21911,.F.);
#27766=ORIENTED_EDGE('',*,*,#21280,.T.);
#27767=ORIENTED_EDGE('',*,*,#21912,.T.);
#27768=ORIENTED_EDGE('',*,*,#21201,.T.);
#27769=ORIENTED_EDGE('',*,*,#21913,.F.);
#27770=ORIENTED_EDGE('',*,*,#21343,.T.);
#27771=ORIENTED_EDGE('',*,*,#21202,.T.);
#27772=ORIENTED_EDGE('',*,*,#21912,.F.);
#27773=ORIENTED_EDGE('',*,*,#21279,.T.);
#27774=ORIENTED_EDGE('',*,*,#21911,.T.);
#27775=ORIENTED_EDGE('',*,*,#21913,.T.);
#27776=ORIENTED_EDGE('',*,*,#21914,.T.);
#27777=ORIENTED_EDGE('',*,*,#21915,.T.);
#27778=ORIENTED_EDGE('',*,*,#21916,.T.);
#27779=ORIENTED_EDGE('',*,*,#21917,.F.);
#27780=ORIENTED_EDGE('',*,*,#21918,.T.);
#27781=ORIENTED_EDGE('',*,*,#21919,.T.);
#27782=ORIENTED_EDGE('',*,*,#21920,.T.);
#27783=ORIENTED_EDGE('',*,*,#21908,.T.);
#27784=ORIENTED_EDGE('',*,*,#21910,.T.);
#27785=ORIENTED_EDGE('',*,*,#21921,.F.);
#27786=ORIENTED_EDGE('',*,*,#21921,.T.);
#27787=ORIENTED_EDGE('',*,*,#21281,.F.);
#27788=ORIENTED_EDGE('',*,*,#21917,.T.);
#27789=ORIENTED_EDGE('',*,*,#21855,.T.);
#27790=ORIENTED_EDGE('',*,*,#21920,.F.);
#27791=ORIENTED_EDGE('',*,*,#21883,.F.);
#27792=ORIENTED_EDGE('',*,*,#21914,.F.);
#27793=ORIENTED_EDGE('',*,*,#21200,.T.);
#27794=ORIENTED_EDGE('',*,*,#21853,.T.);
#27795=ORIENTED_EDGE('',*,*,#21922,.T.);
#27796=ORIENTED_EDGE('',*,*,#21885,.T.);
#27797=ORIENTED_EDGE('',*,*,#21923,.F.);
#27798=ORIENTED_EDGE('',*,*,#21852,.T.);
#27799=ORIENTED_EDGE('',*,*,#21924,.T.);
#27800=ORIENTED_EDGE('',*,*,#21876,.F.);
#27801=ORIENTED_EDGE('',*,*,#21922,.F.);
#27802=ORIENTED_EDGE('',*,*,#21878,.T.);
#27803=ORIENTED_EDGE('',*,*,#21925,.T.);
#27804=ORIENTED_EDGE('',*,*,#21850,.F.);
#27805=ORIENTED_EDGE('',*,*,#21926,.T.);
#27806=ORIENTED_EDGE('',*,*,#21880,.T.);
#27807=ORIENTED_EDGE('',*,*,#21927,.T.);
#27808=ORIENTED_EDGE('',*,*,#21858,.F.);
#27809=ORIENTED_EDGE('',*,*,#21928,.F.);
#27810=ORIENTED_EDGE('',*,*,#21857,.T.);
#27811=ORIENTED_EDGE('',*,*,#21929,.T.);
#27812=ORIENTED_EDGE('',*,*,#21881,.T.);
#27813=ORIENTED_EDGE('',*,*,#21928,.T.);
#27814=ORIENTED_EDGE('',*,*,#21915,.F.);
#27815=ORIENTED_EDGE('',*,*,#21882,.F.);
#27816=ORIENTED_EDGE('',*,*,#21929,.F.);
#27817=ORIENTED_EDGE('',*,*,#21856,.T.);
#27818=ORIENTED_EDGE('',*,*,#21916,.F.);
#27819=ORIENTED_EDGE('',*,*,#21918,.F.);
#27820=ORIENTED_EDGE('',*,*,#21854,.T.);
#27821=ORIENTED_EDGE('',*,*,#21923,.T.);
#27822=ORIENTED_EDGE('',*,*,#21884,.T.);
#27823=ORIENTED_EDGE('',*,*,#21919,.F.);
#27824=ORIENTED_EDGE('',*,*,#21930,.T.);
#27825=ORIENTED_EDGE('',*,*,#21931,.T.);
#27826=ORIENTED_EDGE('',*,*,#21932,.T.);
#27827=ORIENTED_EDGE('',*,*,#21902,.T.);
#27828=ORIENTED_EDGE('',*,*,#21904,.T.);
#27829=ORIENTED_EDGE('',*,*,#21933,.F.);
#27830=ORIENTED_EDGE('',*,*,#21905,.T.);
#27831=ORIENTED_EDGE('',*,*,#21907,.T.);
#27832=ORIENTED_EDGE('',*,*,#21934,.T.);
#27833=ORIENTED_EDGE('',*,*,#21935,.T.);
#27834=ORIENTED_EDGE('',*,*,#21936,.T.);
#27835=ORIENTED_EDGE('',*,*,#21937,.F.);
#27836=ORIENTED_EDGE('',*,*,#21937,.T.);
#27837=ORIENTED_EDGE('',*,*,#21351,.F.);
#27838=ORIENTED_EDGE('',*,*,#21933,.T.);
#27839=ORIENTED_EDGE('',*,*,#21267,.T.);
#27840=ORIENTED_EDGE('',*,*,#21934,.F.);
#27841=ORIENTED_EDGE('',*,*,#21214,.F.);
#27842=ORIENTED_EDGE('',*,*,#21932,.F.);
#27843=ORIENTED_EDGE('',*,*,#21503,.T.);
#27844=ORIENTED_EDGE('',*,*,#21349,.T.);
#27845=ORIENTED_EDGE('',*,*,#21938,.F.);
#27846=ORIENTED_EDGE('',*,*,#21505,.T.);
#27847=ORIENTED_EDGE('',*,*,#21939,.F.);
#27848=ORIENTED_EDGE('',*,*,#21348,.F.);
#27849=ORIENTED_EDGE('',*,*,#21940,.T.);
#27850=ORIENTED_EDGE('',*,*,#21506,.T.);
#27851=ORIENTED_EDGE('',*,*,#21938,.T.);
#27852=ORIENTED_EDGE('',*,*,#21346,.T.);
#27853=ORIENTED_EDGE('',*,*,#21941,.T.);
#27854=ORIENTED_EDGE('',*,*,#21498,.F.);
#27855=ORIENTED_EDGE('',*,*,#21942,.T.);
#27856=ORIENTED_EDGE('',*,*,#21500,.F.);
#27857=ORIENTED_EDGE('',*,*,#21943,.T.);
#27858=ORIENTED_EDGE('',*,*,#21344,.T.);
#27859=ORIENTED_EDGE('',*,*,#21944,.F.);
#27860=ORIENTED_EDGE('',*,*,#21353,.T.);
#27861=ORIENTED_EDGE('',*,*,#21945,.T.);
#27862=ORIENTED_EDGE('',*,*,#21501,.T.);
#27863=ORIENTED_EDGE('',*,*,#21944,.T.);
#27864=ORIENTED_EDGE('',*,*,#21935,.F.);
#27865=ORIENTED_EDGE('',*,*,#21502,.F.);
#27866=ORIENTED_EDGE('',*,*,#21945,.F.);
#27867=ORIENTED_EDGE('',*,*,#21352,.T.);
#27868=ORIENTED_EDGE('',*,*,#21936,.F.);
#27869=ORIENTED_EDGE('',*,*,#21930,.F.);
#27870=ORIENTED_EDGE('',*,*,#21350,.T.);
#27871=ORIENTED_EDGE('',*,*,#21939,.T.);
#27872=ORIENTED_EDGE('',*,*,#21504,.T.);
#27873=ORIENTED_EDGE('',*,*,#21931,.F.);
#27874=ORIENTED_EDGE('',*,*,#21237,.T.);
#27875=ORIENTED_EDGE('',*,*,#21946,.F.);
#27876=ORIENTED_EDGE('',*,*,#21284,.T.);
#27877=ORIENTED_EDGE('',*,*,#21947,.F.);
#27878=ORIENTED_EDGE('',*,*,#21948,.F.);
#27879=ORIENTED_EDGE('',*,*,#21286,.F.);
#27880=ORIENTED_EDGE('',*,*,#21949,.F.);
#27881=ORIENTED_EDGE('',*,*,#21233,.F.);
#27882=ORIENTED_EDGE('',*,*,#21946,.T.);
#27883=ORIENTED_EDGE('',*,*,#21950,.T.);
#27884=ORIENTED_EDGE('',*,*,#21951,.T.);
#27885=ORIENTED_EDGE('',*,*,#21952,.T.);
#27886=ORIENTED_EDGE('',*,*,#21949,.T.);
#27887=ORIENTED_EDGE('',*,*,#21285,.T.);
#27888=ORIENTED_EDGE('',*,*,#21948,.T.);
#27889=ORIENTED_EDGE('',*,*,#21953,.T.);
#27890=ORIENTED_EDGE('',*,*,#21954,.T.);
#27891=ORIENTED_EDGE('',*,*,#21955,.T.);
#27892=ORIENTED_EDGE('',*,*,#21947,.T.);
#27893=ORIENTED_EDGE('',*,*,#21287,.T.);
#27894=ORIENTED_EDGE('',*,*,#21956,.T.);
#27895=ORIENTED_EDGE('',*,*,#21234,.T.);
#27896=ORIENTED_EDGE('',*,*,#21952,.F.);
#27897=ORIENTED_EDGE('',*,*,#21957,.F.);
#27898=ORIENTED_EDGE('',*,*,#21958,.F.);
#27899=ORIENTED_EDGE('',*,*,#21959,.F.);
#27900=ORIENTED_EDGE('',*,*,#21960,.F.);
#27901=ORIENTED_EDGE('',*,*,#21961,.F.);
#27902=ORIENTED_EDGE('',*,*,#21953,.F.);
#27903=ORIENTED_EDGE('',*,*,#21232,.T.);
#27904=ORIENTED_EDGE('',*,*,#21962,.T.);
#27905=ORIENTED_EDGE('',*,*,#21963,.T.);
#27906=ORIENTED_EDGE('',*,*,#21964,.T.);
#27907=ORIENTED_EDGE('',*,*,#21965,.T.);
#27908=ORIENTED_EDGE('',*,*,#21966,.T.);
#27909=ORIENTED_EDGE('',*,*,#21967,.T.);
#27910=ORIENTED_EDGE('',*,*,#21968,.T.);
#27911=ORIENTED_EDGE('',*,*,#21238,.T.);
#27912=ORIENTED_EDGE('',*,*,#21955,.F.);
#27913=ORIENTED_EDGE('',*,*,#21969,.T.);
#27914=ORIENTED_EDGE('',*,*,#21970,.F.);
#27915=ORIENTED_EDGE('',*,*,#21971,.T.);
#27916=ORIENTED_EDGE('',*,*,#21972,.F.);
#27917=ORIENTED_EDGE('',*,*,#21973,.T.);
#27918=ORIENTED_EDGE('',*,*,#21950,.F.);
#27919=ORIENTED_EDGE('',*,*,#21236,.T.);
#27920=ORIENTED_EDGE('',*,*,#21974,.T.);
#27921=ORIENTED_EDGE('',*,*,#21975,.F.);
#27922=ORIENTED_EDGE('',*,*,#21976,.T.);
#27923=ORIENTED_EDGE('',*,*,#21977,.F.);
#27924=ORIENTED_EDGE('',*,*,#21978,.T.);
#27925=ORIENTED_EDGE('',*,*,#21979,.F.);
#27926=ORIENTED_EDGE('',*,*,#21972,.T.);
#27927=ORIENTED_EDGE('',*,*,#21980,.T.);
#27928=ORIENTED_EDGE('',*,*,#21958,.T.);
#27929=ORIENTED_EDGE('',*,*,#21981,.T.);
#27930=ORIENTED_EDGE('',*,*,#21970,.T.);
#27931=ORIENTED_EDGE('',*,*,#21982,.T.);
#27932=ORIENTED_EDGE('',*,*,#21960,.T.);
#27933=ORIENTED_EDGE('',*,*,#21983,.T.);
#27934=ORIENTED_EDGE('',*,*,#21957,.T.);
#27935=ORIENTED_EDGE('',*,*,#21951,.F.);
#27936=ORIENTED_EDGE('',*,*,#21973,.F.);
#27937=ORIENTED_EDGE('',*,*,#21981,.F.);
#27938=ORIENTED_EDGE('',*,*,#21969,.F.);
#27939=ORIENTED_EDGE('',*,*,#21954,.F.);
#27940=ORIENTED_EDGE('',*,*,#21961,.T.);
#27941=ORIENTED_EDGE('',*,*,#21982,.F.);
#27942=ORIENTED_EDGE('',*,*,#21959,.T.);
#27943=ORIENTED_EDGE('',*,*,#21980,.F.);
#27944=ORIENTED_EDGE('',*,*,#21971,.F.);
#27945=ORIENTED_EDGE('',*,*,#21983,.F.);
#27946=ORIENTED_EDGE('',*,*,#21189,.F.);
#27947=ORIENTED_EDGE('',*,*,#21976,.F.);
#27948=ORIENTED_EDGE('',*,*,#21984,.F.);
#27949=ORIENTED_EDGE('',*,*,#21966,.F.);
#27950=ORIENTED_EDGE('',*,*,#21985,.F.);
#27951=ORIENTED_EDGE('',*,*,#21978,.F.);
#27952=ORIENTED_EDGE('',*,*,#21986,.F.);
#27953=ORIENTED_EDGE('',*,*,#21964,.F.);
#27954=ORIENTED_EDGE('',*,*,#21987,.F.);
#27955=ORIENTED_EDGE('',*,*,#21968,.F.);
#27956=ORIENTED_EDGE('',*,*,#21988,.F.);
#27957=ORIENTED_EDGE('',*,*,#21962,.F.);
#27958=ORIENTED_EDGE('',*,*,#21239,.F.);
#27959=ORIENTED_EDGE('',*,*,#21974,.F.);
#27960=ORIENTED_EDGE('',*,*,#21235,.F.);
#27961=ORIENTED_EDGE('',*,*,#21956,.F.);
#27962=ORIENTED_EDGE('',*,*,#21989,.F.);
#27963=ORIENTED_EDGE('',*,*,#21967,.F.);
#27964=ORIENTED_EDGE('',*,*,#21984,.T.);
#27965=ORIENTED_EDGE('',*,*,#21975,.T.);
#27966=ORIENTED_EDGE('',*,*,#21989,.T.);
#27967=ORIENTED_EDGE('',*,*,#21979,.T.);
#27968=ORIENTED_EDGE('',*,*,#21987,.T.);
#27969=ORIENTED_EDGE('',*,*,#21963,.F.);
#27970=ORIENTED_EDGE('',*,*,#21988,.T.);
#27971=ORIENTED_EDGE('',*,*,#21965,.F.);
#27972=ORIENTED_EDGE('',*,*,#21986,.T.);
#27973=ORIENTED_EDGE('',*,*,#21977,.T.);
#27974=ORIENTED_EDGE('',*,*,#21985,.T.);
#27975=ORIENTED_EDGE('',*,*,#21191,.T.);
#27976=ORIENTED_EDGE('',*,*,#21245,.T.);
#27977=ORIENTED_EDGE('',*,*,#21990,.F.);
#27978=ORIENTED_EDGE('',*,*,#21288,.T.);
#27979=ORIENTED_EDGE('',*,*,#21991,.F.);
#27980=ORIENTED_EDGE('',*,*,#21992,.F.);
#27981=ORIENTED_EDGE('',*,*,#21290,.F.);
#27982=ORIENTED_EDGE('',*,*,#21993,.F.);
#27983=ORIENTED_EDGE('',*,*,#21241,.F.);
#27984=ORIENTED_EDGE('',*,*,#21990,.T.);
#27985=ORIENTED_EDGE('',*,*,#21994,.T.);
#27986=ORIENTED_EDGE('',*,*,#21995,.T.);
#27987=ORIENTED_EDGE('',*,*,#21996,.T.);
#27988=ORIENTED_EDGE('',*,*,#21993,.T.);
#27989=ORIENTED_EDGE('',*,*,#21289,.T.);
#27990=ORIENTED_EDGE('',*,*,#21992,.T.);
#27991=ORIENTED_EDGE('',*,*,#21997,.T.);
#27992=ORIENTED_EDGE('',*,*,#21998,.T.);
#27993=ORIENTED_EDGE('',*,*,#21999,.T.);
#27994=ORIENTED_EDGE('',*,*,#21991,.T.);
#27995=ORIENTED_EDGE('',*,*,#21291,.T.);
#27996=ORIENTED_EDGE('',*,*,#22000,.T.);
#27997=ORIENTED_EDGE('',*,*,#21242,.T.);
#27998=ORIENTED_EDGE('',*,*,#21996,.F.);
#27999=ORIENTED_EDGE('',*,*,#22001,.F.);
#28000=ORIENTED_EDGE('',*,*,#22002,.F.);
#28001=ORIENTED_EDGE('',*,*,#22003,.F.);
#28002=ORIENTED_EDGE('',*,*,#22004,.F.);
#28003=ORIENTED_EDGE('',*,*,#22005,.F.);
#28004=ORIENTED_EDGE('',*,*,#21997,.F.);
#28005=ORIENTED_EDGE('',*,*,#21240,.T.);
#28006=ORIENTED_EDGE('',*,*,#22006,.T.);
#28007=ORIENTED_EDGE('',*,*,#22007,.T.);
#28008=ORIENTED_EDGE('',*,*,#22008,.T.);
#28009=ORIENTED_EDGE('',*,*,#22009,.T.);
#28010=ORIENTED_EDGE('',*,*,#22010,.T.);
#28011=ORIENTED_EDGE('',*,*,#22011,.T.);
#28012=ORIENTED_EDGE('',*,*,#22012,.T.);
#28013=ORIENTED_EDGE('',*,*,#21246,.T.);
#28014=ORIENTED_EDGE('',*,*,#21999,.F.);
#28015=ORIENTED_EDGE('',*,*,#22013,.T.);
#28016=ORIENTED_EDGE('',*,*,#22014,.F.);
#28017=ORIENTED_EDGE('',*,*,#22015,.T.);
#28018=ORIENTED_EDGE('',*,*,#22016,.F.);
#28019=ORIENTED_EDGE('',*,*,#22017,.T.);
#28020=ORIENTED_EDGE('',*,*,#21994,.F.);
#28021=ORIENTED_EDGE('',*,*,#21244,.T.);
#28022=ORIENTED_EDGE('',*,*,#22018,.T.);
#28023=ORIENTED_EDGE('',*,*,#22019,.F.);
#28024=ORIENTED_EDGE('',*,*,#22020,.T.);
#28025=ORIENTED_EDGE('',*,*,#22021,.F.);
#28026=ORIENTED_EDGE('',*,*,#22022,.T.);
#28027=ORIENTED_EDGE('',*,*,#22023,.F.);
#28028=ORIENTED_EDGE('',*,*,#22016,.T.);
#28029=ORIENTED_EDGE('',*,*,#22024,.T.);
#28030=ORIENTED_EDGE('',*,*,#22002,.T.);
#28031=ORIENTED_EDGE('',*,*,#22025,.T.);
#28032=ORIENTED_EDGE('',*,*,#22014,.T.);
#28033=ORIENTED_EDGE('',*,*,#22026,.T.);
#28034=ORIENTED_EDGE('',*,*,#22004,.T.);
#28035=ORIENTED_EDGE('',*,*,#22027,.T.);
#28036=ORIENTED_EDGE('',*,*,#22001,.T.);
#28037=ORIENTED_EDGE('',*,*,#21995,.F.);
#28038=ORIENTED_EDGE('',*,*,#22017,.F.);
#28039=ORIENTED_EDGE('',*,*,#22025,.F.);
#28040=ORIENTED_EDGE('',*,*,#22013,.F.);
#28041=ORIENTED_EDGE('',*,*,#21998,.F.);
#28042=ORIENTED_EDGE('',*,*,#22005,.T.);
#28043=ORIENTED_EDGE('',*,*,#22026,.F.);
#28044=ORIENTED_EDGE('',*,*,#22003,.T.);
#28045=ORIENTED_EDGE('',*,*,#22024,.F.);
#28046=ORIENTED_EDGE('',*,*,#22015,.F.);
#28047=ORIENTED_EDGE('',*,*,#22027,.F.);
#28048=ORIENTED_EDGE('',*,*,#21186,.F.);
#28049=ORIENTED_EDGE('',*,*,#22020,.F.);
#28050=ORIENTED_EDGE('',*,*,#22028,.F.);
#28051=ORIENTED_EDGE('',*,*,#22010,.F.);
#28052=ORIENTED_EDGE('',*,*,#22029,.F.);
#28053=ORIENTED_EDGE('',*,*,#22022,.F.);
#28054=ORIENTED_EDGE('',*,*,#22030,.F.);
#28055=ORIENTED_EDGE('',*,*,#22008,.F.);
#28056=ORIENTED_EDGE('',*,*,#22031,.F.);
#28057=ORIENTED_EDGE('',*,*,#22012,.F.);
#28058=ORIENTED_EDGE('',*,*,#22032,.F.);
#28059=ORIENTED_EDGE('',*,*,#22006,.F.);
#28060=ORIENTED_EDGE('',*,*,#21247,.F.);
#28061=ORIENTED_EDGE('',*,*,#22018,.F.);
#28062=ORIENTED_EDGE('',*,*,#21243,.F.);
#28063=ORIENTED_EDGE('',*,*,#22000,.F.);
#28064=ORIENTED_EDGE('',*,*,#22033,.F.);
#28065=ORIENTED_EDGE('',*,*,#22011,.F.);
#28066=ORIENTED_EDGE('',*,*,#22028,.T.);
#28067=ORIENTED_EDGE('',*,*,#22019,.T.);
#28068=ORIENTED_EDGE('',*,*,#22033,.T.);
#28069=ORIENTED_EDGE('',*,*,#22023,.T.);
#28070=ORIENTED_EDGE('',*,*,#22031,.T.);
#28071=ORIENTED_EDGE('',*,*,#22007,.F.);
#28072=ORIENTED_EDGE('',*,*,#22032,.T.);
#28073=ORIENTED_EDGE('',*,*,#22009,.F.);
#28074=ORIENTED_EDGE('',*,*,#22030,.T.);
#28075=ORIENTED_EDGE('',*,*,#22021,.T.);
#28076=ORIENTED_EDGE('',*,*,#22029,.T.);
#28077=ORIENTED_EDGE('',*,*,#21188,.T.);
#28078=ORIENTED_EDGE('',*,*,#21229,.T.);
#28079=ORIENTED_EDGE('',*,*,#22034,.F.);
#28080=ORIENTED_EDGE('',*,*,#21292,.T.);
#28081=ORIENTED_EDGE('',*,*,#22035,.F.);
#28082=ORIENTED_EDGE('',*,*,#22036,.F.);
#28083=ORIENTED_EDGE('',*,*,#21294,.F.);
#28084=ORIENTED_EDGE('',*,*,#22037,.F.);
#28085=ORIENTED_EDGE('',*,*,#21225,.F.);
#28086=ORIENTED_EDGE('',*,*,#22034,.T.);
#28087=ORIENTED_EDGE('',*,*,#22038,.T.);
#28088=ORIENTED_EDGE('',*,*,#22039,.T.);
#28089=ORIENTED_EDGE('',*,*,#22040,.T.);
#28090=ORIENTED_EDGE('',*,*,#22037,.T.);
#28091=ORIENTED_EDGE('',*,*,#21293,.T.);
#28092=ORIENTED_EDGE('',*,*,#22036,.T.);
#28093=ORIENTED_EDGE('',*,*,#22041,.T.);
#28094=ORIENTED_EDGE('',*,*,#22042,.T.);
#28095=ORIENTED_EDGE('',*,*,#22043,.T.);
#28096=ORIENTED_EDGE('',*,*,#22035,.T.);
#28097=ORIENTED_EDGE('',*,*,#21295,.T.);
#28098=ORIENTED_EDGE('',*,*,#22044,.T.);
#28099=ORIENTED_EDGE('',*,*,#21226,.T.);
#28100=ORIENTED_EDGE('',*,*,#22040,.F.);
#28101=ORIENTED_EDGE('',*,*,#22045,.F.);
#28102=ORIENTED_EDGE('',*,*,#22046,.F.);
#28103=ORIENTED_EDGE('',*,*,#22047,.F.);
#28104=ORIENTED_EDGE('',*,*,#22048,.F.);
#28105=ORIENTED_EDGE('',*,*,#22049,.F.);
#28106=ORIENTED_EDGE('',*,*,#22041,.F.);
#28107=ORIENTED_EDGE('',*,*,#21224,.T.);
#28108=ORIENTED_EDGE('',*,*,#22050,.T.);
#28109=ORIENTED_EDGE('',*,*,#22051,.T.);
#28110=ORIENTED_EDGE('',*,*,#22052,.T.);
#28111=ORIENTED_EDGE('',*,*,#22053,.T.);
#28112=ORIENTED_EDGE('',*,*,#22054,.T.);
#28113=ORIENTED_EDGE('',*,*,#22055,.T.);
#28114=ORIENTED_EDGE('',*,*,#22056,.T.);
#28115=ORIENTED_EDGE('',*,*,#21230,.T.);
#28116=ORIENTED_EDGE('',*,*,#22043,.F.);
#28117=ORIENTED_EDGE('',*,*,#22057,.T.);
#28118=ORIENTED_EDGE('',*,*,#22058,.F.);
#28119=ORIENTED_EDGE('',*,*,#22059,.T.);
#28120=ORIENTED_EDGE('',*,*,#22060,.F.);
#28121=ORIENTED_EDGE('',*,*,#22061,.T.);
#28122=ORIENTED_EDGE('',*,*,#22038,.F.);
#28123=ORIENTED_EDGE('',*,*,#21228,.T.);
#28124=ORIENTED_EDGE('',*,*,#22062,.T.);
#28125=ORIENTED_EDGE('',*,*,#22063,.F.);
#28126=ORIENTED_EDGE('',*,*,#22064,.T.);
#28127=ORIENTED_EDGE('',*,*,#22065,.F.);
#28128=ORIENTED_EDGE('',*,*,#22066,.T.);
#28129=ORIENTED_EDGE('',*,*,#22067,.F.);
#28130=ORIENTED_EDGE('',*,*,#22060,.T.);
#28131=ORIENTED_EDGE('',*,*,#22068,.T.);
#28132=ORIENTED_EDGE('',*,*,#22046,.T.);
#28133=ORIENTED_EDGE('',*,*,#22069,.T.);
#28134=ORIENTED_EDGE('',*,*,#22058,.T.);
#28135=ORIENTED_EDGE('',*,*,#22070,.T.);
#28136=ORIENTED_EDGE('',*,*,#22048,.T.);
#28137=ORIENTED_EDGE('',*,*,#22071,.T.);
#28138=ORIENTED_EDGE('',*,*,#22045,.T.);
#28139=ORIENTED_EDGE('',*,*,#22039,.F.);
#28140=ORIENTED_EDGE('',*,*,#22061,.F.);
#28141=ORIENTED_EDGE('',*,*,#22069,.F.);
#28142=ORIENTED_EDGE('',*,*,#22057,.F.);
#28143=ORIENTED_EDGE('',*,*,#22042,.F.);
#28144=ORIENTED_EDGE('',*,*,#22049,.T.);
#28145=ORIENTED_EDGE('',*,*,#22070,.F.);
#28146=ORIENTED_EDGE('',*,*,#22047,.T.);
#28147=ORIENTED_EDGE('',*,*,#22068,.F.);
#28148=ORIENTED_EDGE('',*,*,#22059,.F.);
#28149=ORIENTED_EDGE('',*,*,#22071,.F.);
#28150=ORIENTED_EDGE('',*,*,#21183,.F.);
#28151=ORIENTED_EDGE('',*,*,#22064,.F.);
#28152=ORIENTED_EDGE('',*,*,#22072,.F.);
#28153=ORIENTED_EDGE('',*,*,#22054,.F.);
#28154=ORIENTED_EDGE('',*,*,#22073,.F.);
#28155=ORIENTED_EDGE('',*,*,#22066,.F.);
#28156=ORIENTED_EDGE('',*,*,#22074,.F.);
#28157=ORIENTED_EDGE('',*,*,#22052,.F.);
#28158=ORIENTED_EDGE('',*,*,#22075,.F.);
#28159=ORIENTED_EDGE('',*,*,#22056,.F.);
#28160=ORIENTED_EDGE('',*,*,#22076,.F.);
#28161=ORIENTED_EDGE('',*,*,#22050,.F.);
#28162=ORIENTED_EDGE('',*,*,#21231,.F.);
#28163=ORIENTED_EDGE('',*,*,#22062,.F.);
#28164=ORIENTED_EDGE('',*,*,#21227,.F.);
#28165=ORIENTED_EDGE('',*,*,#22044,.F.);
#28166=ORIENTED_EDGE('',*,*,#22077,.F.);
#28167=ORIENTED_EDGE('',*,*,#22055,.F.);
#28168=ORIENTED_EDGE('',*,*,#22072,.T.);
#28169=ORIENTED_EDGE('',*,*,#22063,.T.);
#28170=ORIENTED_EDGE('',*,*,#22077,.T.);
#28171=ORIENTED_EDGE('',*,*,#22067,.T.);
#28172=ORIENTED_EDGE('',*,*,#22075,.T.);
#28173=ORIENTED_EDGE('',*,*,#22051,.F.);
#28174=ORIENTED_EDGE('',*,*,#22076,.T.);
#28175=ORIENTED_EDGE('',*,*,#22053,.F.);
#28176=ORIENTED_EDGE('',*,*,#22074,.T.);
#28177=ORIENTED_EDGE('',*,*,#22065,.T.);
#28178=ORIENTED_EDGE('',*,*,#22073,.T.);
#28179=ORIENTED_EDGE('',*,*,#21185,.T.);
#28180=ORIENTED_EDGE('',*,*,#21253,.T.);
#28181=ORIENTED_EDGE('',*,*,#22078,.F.);
#28182=ORIENTED_EDGE('',*,*,#21296,.T.);
#28183=ORIENTED_EDGE('',*,*,#22079,.F.);
#28184=ORIENTED_EDGE('',*,*,#22080,.F.);
#28185=ORIENTED_EDGE('',*,*,#21298,.F.);
#28186=ORIENTED_EDGE('',*,*,#22081,.F.);
#28187=ORIENTED_EDGE('',*,*,#21249,.F.);
#28188=ORIENTED_EDGE('',*,*,#22078,.T.);
#28189=ORIENTED_EDGE('',*,*,#22082,.T.);
#28190=ORIENTED_EDGE('',*,*,#22083,.T.);
#28191=ORIENTED_EDGE('',*,*,#22084,.T.);
#28192=ORIENTED_EDGE('',*,*,#22081,.T.);
#28193=ORIENTED_EDGE('',*,*,#21297,.T.);
#28194=ORIENTED_EDGE('',*,*,#22080,.T.);
#28195=ORIENTED_EDGE('',*,*,#22085,.T.);
#28196=ORIENTED_EDGE('',*,*,#22086,.T.);
#28197=ORIENTED_EDGE('',*,*,#22087,.T.);
#28198=ORIENTED_EDGE('',*,*,#22079,.T.);
#28199=ORIENTED_EDGE('',*,*,#21299,.T.);
#28200=ORIENTED_EDGE('',*,*,#22088,.T.);
#28201=ORIENTED_EDGE('',*,*,#21250,.T.);
#28202=ORIENTED_EDGE('',*,*,#22084,.F.);
#28203=ORIENTED_EDGE('',*,*,#22089,.F.);
#28204=ORIENTED_EDGE('',*,*,#22090,.F.);
#28205=ORIENTED_EDGE('',*,*,#22091,.F.);
#28206=ORIENTED_EDGE('',*,*,#22092,.F.);
#28207=ORIENTED_EDGE('',*,*,#22093,.F.);
#28208=ORIENTED_EDGE('',*,*,#22085,.F.);
#28209=ORIENTED_EDGE('',*,*,#21248,.T.);
#28210=ORIENTED_EDGE('',*,*,#22094,.T.);
#28211=ORIENTED_EDGE('',*,*,#22095,.T.);
#28212=ORIENTED_EDGE('',*,*,#22096,.T.);
#28213=ORIENTED_EDGE('',*,*,#22097,.T.);
#28214=ORIENTED_EDGE('',*,*,#22098,.T.);
#28215=ORIENTED_EDGE('',*,*,#22099,.T.);
#28216=ORIENTED_EDGE('',*,*,#22100,.T.);
#28217=ORIENTED_EDGE('',*,*,#21254,.T.);
#28218=ORIENTED_EDGE('',*,*,#22087,.F.);
#28219=ORIENTED_EDGE('',*,*,#22101,.T.);
#28220=ORIENTED_EDGE('',*,*,#22102,.F.);
#28221=ORIENTED_EDGE('',*,*,#22103,.T.);
#28222=ORIENTED_EDGE('',*,*,#22104,.F.);
#28223=ORIENTED_EDGE('',*,*,#22105,.T.);
#28224=ORIENTED_EDGE('',*,*,#22082,.F.);
#28225=ORIENTED_EDGE('',*,*,#21252,.T.);
#28226=ORIENTED_EDGE('',*,*,#22106,.T.);
#28227=ORIENTED_EDGE('',*,*,#22107,.F.);
#28228=ORIENTED_EDGE('',*,*,#22108,.T.);
#28229=ORIENTED_EDGE('',*,*,#22109,.F.);
#28230=ORIENTED_EDGE('',*,*,#22110,.T.);
#28231=ORIENTED_EDGE('',*,*,#22111,.F.);
#28232=ORIENTED_EDGE('',*,*,#22104,.T.);
#28233=ORIENTED_EDGE('',*,*,#22112,.T.);
#28234=ORIENTED_EDGE('',*,*,#22090,.T.);
#28235=ORIENTED_EDGE('',*,*,#22113,.T.);
#28236=ORIENTED_EDGE('',*,*,#22102,.T.);
#28237=ORIENTED_EDGE('',*,*,#22114,.T.);
#28238=ORIENTED_EDGE('',*,*,#22092,.T.);
#28239=ORIENTED_EDGE('',*,*,#22115,.T.);
#28240=ORIENTED_EDGE('',*,*,#22089,.T.);
#28241=ORIENTED_EDGE('',*,*,#22083,.F.);
#28242=ORIENTED_EDGE('',*,*,#22105,.F.);
#28243=ORIENTED_EDGE('',*,*,#22113,.F.);
#28244=ORIENTED_EDGE('',*,*,#22101,.F.);
#28245=ORIENTED_EDGE('',*,*,#22086,.F.);
#28246=ORIENTED_EDGE('',*,*,#22093,.T.);
#28247=ORIENTED_EDGE('',*,*,#22114,.F.);
#28248=ORIENTED_EDGE('',*,*,#22091,.T.);
#28249=ORIENTED_EDGE('',*,*,#22112,.F.);
#28250=ORIENTED_EDGE('',*,*,#22103,.F.);
#28251=ORIENTED_EDGE('',*,*,#22115,.F.);
#28252=ORIENTED_EDGE('',*,*,#21180,.F.);
#28253=ORIENTED_EDGE('',*,*,#22108,.F.);
#28254=ORIENTED_EDGE('',*,*,#22116,.F.);
#28255=ORIENTED_EDGE('',*,*,#22098,.F.);
#28256=ORIENTED_EDGE('',*,*,#22117,.F.);
#28257=ORIENTED_EDGE('',*,*,#22110,.F.);
#28258=ORIENTED_EDGE('',*,*,#22118,.F.);
#28259=ORIENTED_EDGE('',*,*,#22096,.F.);
#28260=ORIENTED_EDGE('',*,*,#22119,.F.);
#28261=ORIENTED_EDGE('',*,*,#22100,.F.);
#28262=ORIENTED_EDGE('',*,*,#22120,.F.);
#28263=ORIENTED_EDGE('',*,*,#22094,.F.);
#28264=ORIENTED_EDGE('',*,*,#21255,.F.);
#28265=ORIENTED_EDGE('',*,*,#22106,.F.);
#28266=ORIENTED_EDGE('',*,*,#21251,.F.);
#28267=ORIENTED_EDGE('',*,*,#22088,.F.);
#28268=ORIENTED_EDGE('',*,*,#22121,.F.);
#28269=ORIENTED_EDGE('',*,*,#22099,.F.);
#28270=ORIENTED_EDGE('',*,*,#22116,.T.);
#28271=ORIENTED_EDGE('',*,*,#22107,.T.);
#28272=ORIENTED_EDGE('',*,*,#22121,.T.);
#28273=ORIENTED_EDGE('',*,*,#22111,.T.);
#28274=ORIENTED_EDGE('',*,*,#22119,.T.);
#28275=ORIENTED_EDGE('',*,*,#22095,.F.);
#28276=ORIENTED_EDGE('',*,*,#22120,.T.);
#28277=ORIENTED_EDGE('',*,*,#22097,.F.);
#28278=ORIENTED_EDGE('',*,*,#22118,.T.);
#28279=ORIENTED_EDGE('',*,*,#22109,.T.);
#28280=ORIENTED_EDGE('',*,*,#22117,.T.);
#28281=ORIENTED_EDGE('',*,*,#21182,.T.);
#28282=ORIENTED_EDGE('',*,*,#21176,.T.);
#28283=ORIENTED_EDGE('',*,*,#21148,.T.);
#28284=ORIENTED_EDGE('',*,*,#22122,.T.);
#28285=ORIENTED_EDGE('',*,*,#21088,.T.);
#28286=ORIENTED_EDGE('',*,*,#21842,.T.);
#28287=ORIENTED_EDGE('',*,*,#22123,.T.);
#28288=ORIENTED_EDGE('',*,*,#21140,.T.);
#28289=ORIENTED_EDGE('',*,*,#22124,.T.);
#28290=ORIENTED_EDGE('',*,*,#22125,.T.);
#28291=ORIENTED_EDGE('',*,*,#22126,.T.);
#28292=ORIENTED_EDGE('',*,*,#22127,.T.);
#28293=ORIENTED_EDGE('',*,*,#22128,.T.);
#28294=ORIENTED_EDGE('',*,*,#22129,.T.);
#28295=ORIENTED_EDGE('',*,*,#22130,.T.);
#28296=ORIENTED_EDGE('',*,*,#21068,.T.);
#28297=ORIENTED_EDGE('',*,*,#22131,.T.);
#28298=ORIENTED_EDGE('',*,*,#22132,.T.);
#28299=ORIENTED_EDGE('',*,*,#22133,.T.);
#28300=ORIENTED_EDGE('',*,*,#22134,.T.);
#28301=ORIENTED_EDGE('',*,*,#22135,.T.);
#28302=ORIENTED_EDGE('',*,*,#22136,.T.);
#28303=ORIENTED_EDGE('',*,*,#22137,.T.);
#28304=ORIENTED_EDGE('',*,*,#22138,.T.);
#28305=ORIENTED_EDGE('',*,*,#22139,.T.);
#28306=ORIENTED_EDGE('',*,*,#21072,.T.);
#28307=ORIENTED_EDGE('',*,*,#22140,.T.);
#28308=ORIENTED_EDGE('',*,*,#22141,.T.);
#28309=ORIENTED_EDGE('',*,*,#22142,.T.);
#28310=ORIENTED_EDGE('',*,*,#22143,.T.);
#28311=ORIENTED_EDGE('',*,*,#22144,.T.);
#28312=ORIENTED_EDGE('',*,*,#22145,.T.);
#28313=ORIENTED_EDGE('',*,*,#22146,.T.);
#28314=ORIENTED_EDGE('',*,*,#22147,.T.);
#28315=ORIENTED_EDGE('',*,*,#22148,.T.);
#28316=ORIENTED_EDGE('',*,*,#21084,.T.);
#28317=ORIENTED_EDGE('',*,*,#22149,.T.);
#28318=ORIENTED_EDGE('',*,*,#22150,.T.);
#28319=ORIENTED_EDGE('',*,*,#22151,.T.);
#28320=ORIENTED_EDGE('',*,*,#22152,.T.);
#28321=ORIENTED_EDGE('',*,*,#22153,.T.);
#28322=ORIENTED_EDGE('',*,*,#22154,.T.);
#28323=ORIENTED_EDGE('',*,*,#22155,.T.);
#28324=ORIENTED_EDGE('',*,*,#21080,.T.);
#28325=ORIENTED_EDGE('',*,*,#22156,.T.);
#28326=ORIENTED_EDGE('',*,*,#21076,.T.);
#28327=ORIENTED_EDGE('',*,*,#22157,.T.);
#28328=ORIENTED_EDGE('',*,*,#22158,.T.);
#28329=ORIENTED_EDGE('',*,*,#22159,.T.);
#28330=ORIENTED_EDGE('',*,*,#22160,.T.);
#28331=ORIENTED_EDGE('',*,*,#22161,.T.);
#28332=ORIENTED_EDGE('',*,*,#22162,.T.);
#28333=ORIENTED_EDGE('',*,*,#21156,.T.);
#28334=ORIENTED_EDGE('',*,*,#22163,.T.);
#28335=ORIENTED_EDGE('',*,*,#21112,.T.);
#28336=ORIENTED_EDGE('',*,*,#21652,.T.);
#28337=ORIENTED_EDGE('',*,*,#22164,.T.);
#28338=ORIENTED_EDGE('',*,*,#21144,.T.);
#28339=ORIENTED_EDGE('',*,*,#22165,.T.);
#28340=ORIENTED_EDGE('',*,*,#22166,.T.);
#28341=ORIENTED_EDGE('',*,*,#21681,.T.);
#28342=ORIENTED_EDGE('',*,*,#22167,.T.);
#28343=ORIENTED_EDGE('',*,*,#22168,.T.);
#28344=ORIENTED_EDGE('',*,*,#22169,.T.);
#28345=ORIENTED_EDGE('',*,*,#21683,.T.);
#28346=ORIENTED_EDGE('',*,*,#21092,.T.);
#28347=ORIENTED_EDGE('',*,*,#22170,.T.);
#28348=ORIENTED_EDGE('',*,*,#22171,.T.);
#28349=ORIENTED_EDGE('',*,*,#21688,.T.);
#28350=ORIENTED_EDGE('',*,*,#22172,.T.);
#28351=ORIENTED_EDGE('',*,*,#22173,.T.);
#28352=ORIENTED_EDGE('',*,*,#22174,.T.);
#28353=ORIENTED_EDGE('',*,*,#21692,.T.);
#28354=ORIENTED_EDGE('',*,*,#22175,.T.);
#28355=ORIENTED_EDGE('',*,*,#22176,.T.);
#28356=ORIENTED_EDGE('',*,*,#21096,.T.);
#28357=ORIENTED_EDGE('',*,*,#21657,.T.);
#28358=ORIENTED_EDGE('',*,*,#22177,.T.);
#28359=ORIENTED_EDGE('',*,*,#22178,.T.);
#28360=ORIENTED_EDGE('',*,*,#22179,.T.);
#28361=ORIENTED_EDGE('',*,*,#21658,.T.);
#28362=ORIENTED_EDGE('',*,*,#22180,.T.);
#28363=ORIENTED_EDGE('',*,*,#22181,.T.);
#28364=ORIENTED_EDGE('',*,*,#22182,.T.);
#28365=ORIENTED_EDGE('',*,*,#21663,.T.);
#28366=ORIENTED_EDGE('',*,*,#21108,.T.);
#28367=ORIENTED_EDGE('',*,*,#22183,.T.);
#28368=ORIENTED_EDGE('',*,*,#22184,.T.);
#28369=ORIENTED_EDGE('',*,*,#21665,.T.);
#28370=ORIENTED_EDGE('',*,*,#22185,.T.);
#28371=ORIENTED_EDGE('',*,*,#22186,.T.);
#28372=ORIENTED_EDGE('',*,*,#22187,.T.);
#28373=ORIENTED_EDGE('',*,*,#21670,.T.);
#28374=ORIENTED_EDGE('',*,*,#21104,.T.);
#28375=ORIENTED_EDGE('',*,*,#22188,.T.);
#28376=ORIENTED_EDGE('',*,*,#21100,.T.);
#28377=ORIENTED_EDGE('',*,*,#21672,.T.);
#28378=ORIENTED_EDGE('',*,*,#22189,.T.);
#28379=ORIENTED_EDGE('',*,*,#22190,.T.);
#28380=ORIENTED_EDGE('',*,*,#22191,.T.);
#28381=ORIENTED_EDGE('',*,*,#21677,.T.);
#28382=ORIENTED_EDGE('',*,*,#22192,.T.);
#28383=ORIENTED_EDGE('',*,*,#21194,.T.);
#28384=ORIENTED_EDGE('',*,*,#21841,.T.);
#28385=ORIENTED_EDGE('',*,*,#21124,.T.);
#28386=ORIENTED_EDGE('',*,*,#21694,.T.);
#28387=ORIENTED_EDGE('',*,*,#22193,.T.);
#28388=ORIENTED_EDGE('',*,*,#21152,.T.);
#28389=ORIENTED_EDGE('',*,*,#22194,.T.);
#28390=ORIENTED_EDGE('',*,*,#22195,.T.);
#28391=ORIENTED_EDGE('',*,*,#21723,.T.);
#28392=ORIENTED_EDGE('',*,*,#22196,.T.);
#28393=ORIENTED_EDGE('',*,*,#21738,.T.);
#28394=ORIENTED_EDGE('',*,*,#22197,.T.);
#28395=ORIENTED_EDGE('',*,*,#21725,.T.);
#28396=ORIENTED_EDGE('',*,*,#21116,.T.);
#28397=ORIENTED_EDGE('',*,*,#22198,.T.);
#28398=ORIENTED_EDGE('',*,*,#22199,.T.);
#28399=ORIENTED_EDGE('',*,*,#21730,.T.);
#28400=ORIENTED_EDGE('',*,*,#22200,.T.);
#28401=ORIENTED_EDGE('',*,*,#22201,.T.);
#28402=ORIENTED_EDGE('',*,*,#22202,.T.);
#28403=ORIENTED_EDGE('',*,*,#21734,.T.);
#28404=ORIENTED_EDGE('',*,*,#22203,.T.);
#28405=ORIENTED_EDGE('',*,*,#22204,.T.);
#28406=ORIENTED_EDGE('',*,*,#21120,.T.);
#28407=ORIENTED_EDGE('',*,*,#21699,.T.);
#28408=ORIENTED_EDGE('',*,*,#22205,.T.);
#28409=ORIENTED_EDGE('',*,*,#21849,.T.);
#28410=ORIENTED_EDGE('',*,*,#22206,.T.);
#28411=ORIENTED_EDGE('',*,*,#21700,.T.);
#28412=ORIENTED_EDGE('',*,*,#22207,.T.);
#28413=ORIENTED_EDGE('',*,*,#22208,.T.);
#28414=ORIENTED_EDGE('',*,*,#22209,.T.);
#28415=ORIENTED_EDGE('',*,*,#21705,.T.);
#28416=ORIENTED_EDGE('',*,*,#21136,.T.);
#28417=ORIENTED_EDGE('',*,*,#21847,.T.);
#28418=ORIENTED_EDGE('',*,*,#22210,.T.);
#28419=ORIENTED_EDGE('',*,*,#21707,.T.);
#28420=ORIENTED_EDGE('',*,*,#22211,.T.);
#28421=ORIENTED_EDGE('',*,*,#22212,.T.);
#28422=ORIENTED_EDGE('',*,*,#22213,.T.);
#28423=ORIENTED_EDGE('',*,*,#21712,.T.);
#28424=ORIENTED_EDGE('',*,*,#21132,.T.);
#28425=ORIENTED_EDGE('',*,*,#21844,.T.);
#28426=ORIENTED_EDGE('',*,*,#21128,.T.);
#28427=ORIENTED_EDGE('',*,*,#21714,.T.);
#28428=ORIENTED_EDGE('',*,*,#22214,.T.);
#28429=ORIENTED_EDGE('',*,*,#22215,.T.);
#28430=ORIENTED_EDGE('',*,*,#22216,.T.);
#28431=ORIENTED_EDGE('',*,*,#21719,.T.);
#28432=ORIENTED_EDGE('',*,*,#22217,.T.);
#28433=ORIENTED_EDGE('',*,*,#22201,.F.);
#28434=ORIENTED_EDGE('',*,*,#22218,.T.);
#28435=ORIENTED_EDGE('',*,*,#21819,.T.);
#28436=ORIENTED_EDGE('',*,*,#22219,.T.);
#28437=ORIENTED_EDGE('',*,*,#21759,.F.);
#28438=ORIENTED_EDGE('',*,*,#22220,.T.);
#28439=ORIENTED_EDGE('',*,*,#22140,.F.);
#28440=ORIENTED_EDGE('',*,*,#21071,.T.);
#28441=ORIENTED_EDGE('',*,*,#22144,.F.);
#28442=ORIENTED_EDGE('',*,*,#22221,.T.);
#28443=ORIENTED_EDGE('',*,*,#21770,.F.);
#28444=ORIENTED_EDGE('',*,*,#22222,.T.);
#28445=ORIENTED_EDGE('',*,*,#21766,.F.);
#28446=ORIENTED_EDGE('',*,*,#21085,.T.);
#28447=ORIENTED_EDGE('',*,*,#22148,.F.);
#28448=ORIENTED_EDGE('',*,*,#22223,.T.);
#28449=ORIENTED_EDGE('',*,*,#22151,.F.);
#28450=ORIENTED_EDGE('',*,*,#22224,.T.);
#28451=ORIENTED_EDGE('',*,*,#21777,.F.);
#28452=ORIENTED_EDGE('',*,*,#22225,.T.);
#28453=ORIENTED_EDGE('',*,*,#21773,.F.);
#28454=ORIENTED_EDGE('',*,*,#21081,.T.);
#28455=ORIENTED_EDGE('',*,*,#22155,.F.);
#28456=ORIENTED_EDGE('',*,*,#22226,.T.);
#28457=ORIENTED_EDGE('',*,*,#22157,.F.);
#28458=ORIENTED_EDGE('',*,*,#21075,.T.);
#28459=ORIENTED_EDGE('',*,*,#21784,.F.);
#28460=ORIENTED_EDGE('',*,*,#22227,.T.);
#28461=ORIENTED_EDGE('',*,*,#21780,.F.);
#28462=ORIENTED_EDGE('',*,*,#22228,.T.);
#28463=ORIENTED_EDGE('',*,*,#22161,.F.);
#28464=ORIENTED_EDGE('',*,*,#22229,.T.);
#28465=ORIENTED_EDGE('',*,*,#21746,.F.);
#28466=ORIENTED_EDGE('',*,*,#22230,.T.);
#28467=ORIENTED_EDGE('',*,*,#22126,.F.);
#28468=ORIENTED_EDGE('',*,*,#22231,.T.);
#28469=ORIENTED_EDGE('',*,*,#22130,.F.);
#28470=ORIENTED_EDGE('',*,*,#22232,.T.);
#28471=ORIENTED_EDGE('',*,*,#21755,.F.);
#28472=ORIENTED_EDGE('',*,*,#21069,.T.);
#28473=ORIENTED_EDGE('',*,*,#21752,.F.);
#28474=ORIENTED_EDGE('',*,*,#22233,.T.);
#28475=ORIENTED_EDGE('',*,*,#22133,.F.);
#28476=ORIENTED_EDGE('',*,*,#22234,.T.);
#28477=ORIENTED_EDGE('',*,*,#21762,.F.);
#28478=ORIENTED_EDGE('',*,*,#22235,.T.);
#28479=ORIENTED_EDGE('',*,*,#22137,.F.);
#28480=ORIENTED_EDGE('',*,*,#22236,.T.);
#28481=ORIENTED_EDGE('',*,*,#21795,.T.);
#28482=ORIENTED_EDGE('',*,*,#22237,.T.);
#28483=ORIENTED_EDGE('',*,*,#22173,.F.);
#28484=ORIENTED_EDGE('',*,*,#22238,.T.);
#28485=ORIENTED_EDGE('',*,*,#22204,.F.);
#28486=ORIENTED_EDGE('',*,*,#22239,.T.);
#28487=ORIENTED_EDGE('',*,*,#21816,.F.);
#28488=ORIENTED_EDGE('',*,*,#21121,.T.);
#28489=ORIENTED_EDGE('',*,*,#21790,.T.);
#28490=ORIENTED_EDGE('',*,*,#22240,.T.);
#28491=ORIENTED_EDGE('',*,*,#22168,.F.);
#28492=ORIENTED_EDGE('',*,*,#22241,.T.);
#28493=ORIENTED_EDGE('',*,*,#22198,.F.);
#28494=ORIENTED_EDGE('',*,*,#21115,.T.);
#28495=ORIENTED_EDGE('',*,*,#21813,.F.);
#28496=ORIENTED_EDGE('',*,*,#22242,.T.);
#28497=ORIENTED_EDGE('',*,*,#21155,.F.);
#28498=ORIENTED_EDGE('',*,*,#21744,.T.);
#28499=ORIENTED_EDGE('',*,*,#21113,.T.);
#28500=ORIENTED_EDGE('',*,*,#22163,.F.);
#28501=ORIENTED_EDGE('',*,*,#21151,.F.);
#28502=ORIENTED_EDGE('',*,*,#21838,.F.);
#28503=ORIENTED_EDGE('',*,*,#22243,.T.);
#28504=ORIENTED_EDGE('',*,*,#22194,.F.);
#28505=ORIENTED_EDGE('',*,*,#21810,.T.);
#28506=ORIENTED_EDGE('',*,*,#21101,.T.);
#28507=ORIENTED_EDGE('',*,*,#22188,.F.);
#28508=ORIENTED_EDGE('',*,*,#22244,.T.);
#28509=ORIENTED_EDGE('',*,*,#22215,.F.);
#28510=ORIENTED_EDGE('',*,*,#22245,.T.);
#28511=ORIENTED_EDGE('',*,*,#21832,.F.);
#28512=ORIENTED_EDGE('',*,*,#22246,.T.);
#28513=ORIENTED_EDGE('',*,*,#21806,.T.);
#28514=ORIENTED_EDGE('',*,*,#22247,.T.);
#28515=ORIENTED_EDGE('',*,*,#22183,.F.);
#28516=ORIENTED_EDGE('',*,*,#21103,.T.);
#28517=ORIENTED_EDGE('',*,*,#22212,.F.);
#28518=ORIENTED_EDGE('',*,*,#22248,.T.);
#28519=ORIENTED_EDGE('',*,*,#21827,.F.);
#28520=ORIENTED_EDGE('',*,*,#22249,.T.);
#28521=ORIENTED_EDGE('',*,*,#22208,.F.);
#28522=ORIENTED_EDGE('',*,*,#22250,.T.);
#28523=ORIENTED_EDGE('',*,*,#21822,.F.);
#28524=ORIENTED_EDGE('',*,*,#22251,.T.);
#28525=ORIENTED_EDGE('',*,*,#21801,.T.);
#28526=ORIENTED_EDGE('',*,*,#22252,.T.);
#28527=ORIENTED_EDGE('',*,*,#22178,.F.);
#28528=ORIENTED_EDGE('',*,*,#21107,.T.);
#28529=ORIENTED_EDGE('',*,*,#21764,.T.);
#28530=ORIENTED_EDGE('',*,*,#22253,.T.);
#28531=ORIENTED_EDGE('',*,*,#22135,.F.);
#28532=ORIENTED_EDGE('',*,*,#22254,.T.);
#28533=ORIENTED_EDGE('',*,*,#22176,.F.);
#28534=ORIENTED_EDGE('',*,*,#22255,.T.);
#28535=ORIENTED_EDGE('',*,*,#21792,.F.);
#28536=ORIENTED_EDGE('',*,*,#21097,.T.);
#28537=ORIENTED_EDGE('',*,*,#21757,.T.);
#28538=ORIENTED_EDGE('',*,*,#22256,.T.);
#28539=ORIENTED_EDGE('',*,*,#22128,.F.);
#28540=ORIENTED_EDGE('',*,*,#22257,.T.);
#28541=ORIENTED_EDGE('',*,*,#22170,.F.);
#28542=ORIENTED_EDGE('',*,*,#21091,.T.);
#28543=ORIENTED_EDGE('',*,*,#21788,.F.);
#28544=ORIENTED_EDGE('',*,*,#22258,.T.);
#28545=ORIENTED_EDGE('',*,*,#21147,.F.);
#28546=ORIENTED_EDGE('',*,*,#21751,.T.);
#28547=ORIENTED_EDGE('',*,*,#21089,.T.);
#28548=ORIENTED_EDGE('',*,*,#22122,.F.);
#28549=ORIENTED_EDGE('',*,*,#21143,.F.);
#28550=ORIENTED_EDGE('',*,*,#21742,.F.);
#28551=ORIENTED_EDGE('',*,*,#22259,.T.);
#28552=ORIENTED_EDGE('',*,*,#22165,.F.);
#28553=ORIENTED_EDGE('',*,*,#21785,.T.);
#28554=ORIENTED_EDGE('',*,*,#21077,.T.);
#28555=ORIENTED_EDGE('',*,*,#22156,.F.);
#28556=ORIENTED_EDGE('',*,*,#22260,.T.);
#28557=ORIENTED_EDGE('',*,*,#22190,.F.);
#28558=ORIENTED_EDGE('',*,*,#22261,.T.);
#28559=ORIENTED_EDGE('',*,*,#21808,.F.);
#28560=ORIENTED_EDGE('',*,*,#22262,.T.);
#28561=ORIENTED_EDGE('',*,*,#21779,.T.);
#28562=ORIENTED_EDGE('',*,*,#22263,.T.);
#28563=ORIENTED_EDGE('',*,*,#22149,.F.);
#28564=ORIENTED_EDGE('',*,*,#21079,.T.);
#28565=ORIENTED_EDGE('',*,*,#22186,.F.);
#28566=ORIENTED_EDGE('',*,*,#22264,.T.);
#28567=ORIENTED_EDGE('',*,*,#21803,.F.);
#28568=ORIENTED_EDGE('',*,*,#22265,.T.);
#28569=ORIENTED_EDGE('',*,*,#22181,.F.);
#28570=ORIENTED_EDGE('',*,*,#22266,.T.);
#28571=ORIENTED_EDGE('',*,*,#21798,.F.);
#28572=ORIENTED_EDGE('',*,*,#22267,.T.);
#28573=ORIENTED_EDGE('',*,*,#21772,.T.);
#28574=ORIENTED_EDGE('',*,*,#22268,.T.);
#28575=ORIENTED_EDGE('',*,*,#22142,.F.);
#28576=ORIENTED_EDGE('',*,*,#21083,.T.);
#28577=ORIENTED_EDGE('',*,*,#22139,.F.);
#28578=ORIENTED_EDGE('',*,*,#22269,.T.);
#28579=ORIENTED_EDGE('',*,*,#21760,.F.);
#28580=ORIENTED_EDGE('',*,*,#21073,.T.);
#28581=ORIENTED_EDGE('',*,*,#22131,.F.);
#28582=ORIENTED_EDGE('',*,*,#21067,.T.);
#28583=ORIENTED_EDGE('',*,*,#21754,.F.);
#28584=ORIENTED_EDGE('',*,*,#22270,.T.);
#28585=ORIENTED_EDGE('',*,*,#21139,.F.);
#28586=ORIENTED_EDGE('',*,*,#21748,.F.);
#28587=ORIENTED_EDGE('',*,*,#22271,.T.);
#28588=ORIENTED_EDGE('',*,*,#22124,.F.);
#28589=ORIENTED_EDGE('',*,*,#22159,.F.);
#28590=ORIENTED_EDGE('',*,*,#22272,.T.);
#28591=ORIENTED_EDGE('',*,*,#21782,.F.);
#28592=ORIENTED_EDGE('',*,*,#22273,.T.);
#28593=ORIENTED_EDGE('',*,*,#22153,.F.);
#28594=ORIENTED_EDGE('',*,*,#22274,.T.);
#28595=ORIENTED_EDGE('',*,*,#21775,.F.);
#28596=ORIENTED_EDGE('',*,*,#22275,.T.);
#28597=ORIENTED_EDGE('',*,*,#22146,.F.);
#28598=ORIENTED_EDGE('',*,*,#22276,.T.);
#28599=ORIENTED_EDGE('',*,*,#21768,.F.);
#28600=ORIENTED_EDGE('',*,*,#22277,.T.);
#28601=ORIENTED_EDGE('',*,*,#22138,.F.);
#28602=ORIENTED_EDGE('',*,*,#22235,.F.);
#28603=ORIENTED_EDGE('',*,*,#21761,.F.);
#28604=ORIENTED_EDGE('',*,*,#22269,.F.);
#28605=ORIENTED_EDGE('',*,*,#22175,.F.);
#28606=ORIENTED_EDGE('',*,*,#21691,.F.);
#28607=ORIENTED_EDGE('',*,*,#21793,.F.);
#28608=ORIENTED_EDGE('',*,*,#22255,.F.);
#28609=ORIENTED_EDGE('',*,*,#21763,.F.);
#28610=ORIENTED_EDGE('',*,*,#22236,.F.);
#28611=ORIENTED_EDGE('',*,*,#22136,.F.);
#28612=ORIENTED_EDGE('',*,*,#22253,.F.);
#28613=ORIENTED_EDGE('',*,*,#22203,.F.);
#28614=ORIENTED_EDGE('',*,*,#21733,.F.);
#28615=ORIENTED_EDGE('',*,*,#21817,.F.);
#28616=ORIENTED_EDGE('',*,*,#22239,.F.);
#28617=ORIENTED_EDGE('',*,*,#21794,.F.);
#28618=ORIENTED_EDGE('',*,*,#21693,.F.);
#28619=ORIENTED_EDGE('',*,*,#22174,.F.);
#28620=ORIENTED_EDGE('',*,*,#22237,.F.);
#28621=ORIENTED_EDGE('',*,*,#21820,.F.);
#28622=ORIENTED_EDGE('',*,*,#22218,.F.);
#28623=ORIENTED_EDGE('',*,*,#22205,.F.);
#28624=ORIENTED_EDGE('',*,*,#21698,.F.);
#28625=ORIENTED_EDGE('',*,*,#21824,.F.);
#28626=ORIENTED_EDGE('',*,*,#21701,.F.);
#28627=ORIENTED_EDGE('',*,*,#22206,.F.);
#28628=ORIENTED_EDGE('',*,*,#21848,.F.);
#28629=ORIENTED_EDGE('',*,*,#21829,.F.);
#28630=ORIENTED_EDGE('',*,*,#21708,.F.);
#28631=ORIENTED_EDGE('',*,*,#22210,.F.);
#28632=ORIENTED_EDGE('',*,*,#21846,.F.);
#28633=ORIENTED_EDGE('',*,*,#21835,.F.);
#28634=ORIENTED_EDGE('',*,*,#21845,.F.);
#28635=ORIENTED_EDGE('',*,*,#22217,.F.);
#28636=ORIENTED_EDGE('',*,*,#21718,.F.);
#28637=ORIENTED_EDGE('',*,*,#21836,.F.);
#28638=ORIENTED_EDGE('',*,*,#21195,.F.);
#28639=ORIENTED_EDGE('',*,*,#22196,.F.);
#28640=ORIENTED_EDGE('',*,*,#21722,.F.);
#28641=ORIENTED_EDGE('',*,*,#21814,.F.);
#28642=ORIENTED_EDGE('',*,*,#21726,.F.);
#28643=ORIENTED_EDGE('',*,*,#22197,.F.);
#28644=ORIENTED_EDGE('',*,*,#21737,.F.);
#28645=ORIENTED_EDGE('',*,*,#21815,.F.);
#28646=ORIENTED_EDGE('',*,*,#21739,.F.);
#28647=ORIENTED_EDGE('',*,*,#22200,.F.);
#28648=ORIENTED_EDGE('',*,*,#21729,.F.);
#28649=ORIENTED_EDGE('',*,*,#21818,.F.);
#28650=ORIENTED_EDGE('',*,*,#21735,.F.);
#28651=ORIENTED_EDGE('',*,*,#22202,.F.);
#28652=ORIENTED_EDGE('',*,*,#22219,.F.);
#28653=ORIENTED_EDGE('',*,*,#22193,.F.);
#28654=ORIENTED_EDGE('',*,*,#21696,.F.);
#28655=ORIENTED_EDGE('',*,*,#21839,.F.);
#28656=ORIENTED_EDGE('',*,*,#21153,.F.);
#28657=ORIENTED_EDGE('',*,*,#22207,.F.);
#28658=ORIENTED_EDGE('',*,*,#21703,.F.);
#28659=ORIENTED_EDGE('',*,*,#21823,.F.);
#28660=ORIENTED_EDGE('',*,*,#22250,.F.);
#28661=ORIENTED_EDGE('',*,*,#21821,.F.);
#28662=ORIENTED_EDGE('',*,*,#21706,.F.);
#28663=ORIENTED_EDGE('',*,*,#22209,.F.);
#28664=ORIENTED_EDGE('',*,*,#22251,.F.);
#28665=ORIENTED_EDGE('',*,*,#22211,.F.);
#28666=ORIENTED_EDGE('',*,*,#21710,.F.);
#28667=ORIENTED_EDGE('',*,*,#21828,.F.);
#28668=ORIENTED_EDGE('',*,*,#22248,.F.);
#28669=ORIENTED_EDGE('',*,*,#21826,.F.);
#28670=ORIENTED_EDGE('',*,*,#21713,.F.);
#28671=ORIENTED_EDGE('',*,*,#22213,.F.);
#28672=ORIENTED_EDGE('',*,*,#22249,.F.);
#28673=ORIENTED_EDGE('',*,*,#22214,.F.);
#28674=ORIENTED_EDGE('',*,*,#21716,.F.);
#28675=ORIENTED_EDGE('',*,*,#21833,.F.);
#28676=ORIENTED_EDGE('',*,*,#22245,.F.);
#28677=ORIENTED_EDGE('',*,*,#21831,.F.);
#28678=ORIENTED_EDGE('',*,*,#21720,.F.);
#28679=ORIENTED_EDGE('',*,*,#22216,.F.);
#28680=ORIENTED_EDGE('',*,*,#22246,.F.);
#28681=ORIENTED_EDGE('',*,*,#21837,.F.);
#28682=ORIENTED_EDGE('',*,*,#21724,.F.);
#28683=ORIENTED_EDGE('',*,*,#22195,.F.);
#28684=ORIENTED_EDGE('',*,*,#22243,.F.);
#28685=ORIENTED_EDGE('',*,*,#21812,.F.);
#28686=ORIENTED_EDGE('',*,*,#21731,.F.);
#28687=ORIENTED_EDGE('',*,*,#22199,.F.);
#28688=ORIENTED_EDGE('',*,*,#22242,.F.);
#28689=ORIENTED_EDGE('',*,*,#22177,.F.);
#28690=ORIENTED_EDGE('',*,*,#21656,.F.);
#28691=ORIENTED_EDGE('',*,*,#21796,.F.);
#28692=ORIENTED_EDGE('',*,*,#22238,.F.);
#28693=ORIENTED_EDGE('',*,*,#21800,.F.);
#28694=ORIENTED_EDGE('',*,*,#21659,.F.);
#28695=ORIENTED_EDGE('',*,*,#22179,.F.);
#28696=ORIENTED_EDGE('',*,*,#22252,.F.);
#28697=ORIENTED_EDGE('',*,*,#21805,.F.);
#28698=ORIENTED_EDGE('',*,*,#21666,.F.);
#28699=ORIENTED_EDGE('',*,*,#22184,.F.);
#28700=ORIENTED_EDGE('',*,*,#22247,.F.);
#28701=ORIENTED_EDGE('',*,*,#22192,.F.);
#28702=ORIENTED_EDGE('',*,*,#21676,.F.);
#28703=ORIENTED_EDGE('',*,*,#21811,.F.);
#28704=ORIENTED_EDGE('',*,*,#22244,.F.);
#28705=ORIENTED_EDGE('',*,*,#22167,.F.);
#28706=ORIENTED_EDGE('',*,*,#21680,.F.);
#28707=ORIENTED_EDGE('',*,*,#21740,.F.);
#28708=ORIENTED_EDGE('',*,*,#21157,.F.);
#28709=ORIENTED_EDGE('',*,*,#21789,.F.);
#28710=ORIENTED_EDGE('',*,*,#21684,.F.);
#28711=ORIENTED_EDGE('',*,*,#22169,.F.);
#28712=ORIENTED_EDGE('',*,*,#22240,.F.);
#28713=ORIENTED_EDGE('',*,*,#22172,.F.);
#28714=ORIENTED_EDGE('',*,*,#21687,.F.);
#28715=ORIENTED_EDGE('',*,*,#21791,.F.);
#28716=ORIENTED_EDGE('',*,*,#22241,.F.);
#28717=ORIENTED_EDGE('',*,*,#22164,.F.);
#28718=ORIENTED_EDGE('',*,*,#21654,.F.);
#28719=ORIENTED_EDGE('',*,*,#21743,.F.);
#28720=ORIENTED_EDGE('',*,*,#21145,.F.);
#28721=ORIENTED_EDGE('',*,*,#22180,.F.);
#28722=ORIENTED_EDGE('',*,*,#21661,.F.);
#28723=ORIENTED_EDGE('',*,*,#21799,.F.);
#28724=ORIENTED_EDGE('',*,*,#22266,.F.);
#28725=ORIENTED_EDGE('',*,*,#21797,.F.);
#28726=ORIENTED_EDGE('',*,*,#21664,.F.);
#28727=ORIENTED_EDGE('',*,*,#22182,.F.);
#28728=ORIENTED_EDGE('',*,*,#22267,.F.);
#28729=ORIENTED_EDGE('',*,*,#22185,.F.);
#28730=ORIENTED_EDGE('',*,*,#21668,.F.);
#28731=ORIENTED_EDGE('',*,*,#21804,.F.);
#28732=ORIENTED_EDGE('',*,*,#22264,.F.);
#28733=ORIENTED_EDGE('',*,*,#21802,.F.);
#28734=ORIENTED_EDGE('',*,*,#21671,.F.);
#28735=ORIENTED_EDGE('',*,*,#22187,.F.);
#28736=ORIENTED_EDGE('',*,*,#22265,.F.);
#28737=ORIENTED_EDGE('',*,*,#22189,.F.);
#28738=ORIENTED_EDGE('',*,*,#21674,.F.);
#28739=ORIENTED_EDGE('',*,*,#21809,.F.);
#28740=ORIENTED_EDGE('',*,*,#22261,.F.);
#28741=ORIENTED_EDGE('',*,*,#21807,.F.);
#28742=ORIENTED_EDGE('',*,*,#21678,.F.);
#28743=ORIENTED_EDGE('',*,*,#22191,.F.);
#28744=ORIENTED_EDGE('',*,*,#22262,.F.);
#28745=ORIENTED_EDGE('',*,*,#21741,.F.);
#28746=ORIENTED_EDGE('',*,*,#21682,.F.);
#28747=ORIENTED_EDGE('',*,*,#22166,.F.);
#28748=ORIENTED_EDGE('',*,*,#22259,.F.);
#28749=ORIENTED_EDGE('',*,*,#21787,.F.);
#28750=ORIENTED_EDGE('',*,*,#21689,.F.);
#28751=ORIENTED_EDGE('',*,*,#22171,.F.);
#28752=ORIENTED_EDGE('',*,*,#22258,.F.);
#28753=ORIENTED_EDGE('',*,*,#22141,.F.);
#28754=ORIENTED_EDGE('',*,*,#22220,.F.);
#28755=ORIENTED_EDGE('',*,*,#21765,.F.);
#28756=ORIENTED_EDGE('',*,*,#22254,.F.);
#28757=ORIENTED_EDGE('',*,*,#21771,.F.);
#28758=ORIENTED_EDGE('',*,*,#22221,.F.);
#28759=ORIENTED_EDGE('',*,*,#22143,.F.);
#28760=ORIENTED_EDGE('',*,*,#22268,.F.);
#28761=ORIENTED_EDGE('',*,*,#21778,.F.);
#28762=ORIENTED_EDGE('',*,*,#22224,.F.);
#28763=ORIENTED_EDGE('',*,*,#22150,.F.);
#28764=ORIENTED_EDGE('',*,*,#22263,.F.);
#28765=ORIENTED_EDGE('',*,*,#22162,.F.);
#28766=ORIENTED_EDGE('',*,*,#22228,.F.);
#28767=ORIENTED_EDGE('',*,*,#21786,.F.);
#28768=ORIENTED_EDGE('',*,*,#22260,.F.);
#28769=ORIENTED_EDGE('',*,*,#22127,.F.);
#28770=ORIENTED_EDGE('',*,*,#22230,.F.);
#28771=ORIENTED_EDGE('',*,*,#21745,.F.);
#28772=ORIENTED_EDGE('',*,*,#21149,.F.);
#28773=ORIENTED_EDGE('',*,*,#21756,.F.);
#28774=ORIENTED_EDGE('',*,*,#22232,.F.);
#28775=ORIENTED_EDGE('',*,*,#22129,.F.);
#28776=ORIENTED_EDGE('',*,*,#22256,.F.);
#28777=ORIENTED_EDGE('',*,*,#22134,.F.);
#28778=ORIENTED_EDGE('',*,*,#22233,.F.);
#28779=ORIENTED_EDGE('',*,*,#21758,.F.);
#28780=ORIENTED_EDGE('',*,*,#22257,.F.);
#28781=ORIENTED_EDGE('',*,*,#22123,.F.);
#28782=ORIENTED_EDGE('',*,*,#21843,.F.);
#28783=ORIENTED_EDGE('',*,*,#21749,.F.);
#28784=ORIENTED_EDGE('',*,*,#21141,.F.);
#28785=ORIENTED_EDGE('',*,*,#22145,.F.);
#28786=ORIENTED_EDGE('',*,*,#22222,.F.);
#28787=ORIENTED_EDGE('',*,*,#21769,.F.);
#28788=ORIENTED_EDGE('',*,*,#22276,.F.);
#28789=ORIENTED_EDGE('',*,*,#21767,.F.);
#28790=ORIENTED_EDGE('',*,*,#22223,.F.);
#28791=ORIENTED_EDGE('',*,*,#22147,.F.);
#28792=ORIENTED_EDGE('',*,*,#22277,.F.);
#28793=ORIENTED_EDGE('',*,*,#22152,.F.);
#28794=ORIENTED_EDGE('',*,*,#22225,.F.);
#28795=ORIENTED_EDGE('',*,*,#21776,.F.);
#28796=ORIENTED_EDGE('',*,*,#22274,.F.);
#28797=ORIENTED_EDGE('',*,*,#21774,.F.);
#28798=ORIENTED_EDGE('',*,*,#22226,.F.);
#28799=ORIENTED_EDGE('',*,*,#22154,.F.);
#28800=ORIENTED_EDGE('',*,*,#22275,.F.);
#28801=ORIENTED_EDGE('',*,*,#22158,.F.);
#28802=ORIENTED_EDGE('',*,*,#22227,.F.);
#28803=ORIENTED_EDGE('',*,*,#21783,.F.);
#28804=ORIENTED_EDGE('',*,*,#22272,.F.);
#28805=ORIENTED_EDGE('',*,*,#21781,.F.);
#28806=ORIENTED_EDGE('',*,*,#22229,.F.);
#28807=ORIENTED_EDGE('',*,*,#22160,.F.);
#28808=ORIENTED_EDGE('',*,*,#22273,.F.);
#28809=ORIENTED_EDGE('',*,*,#21747,.F.);
#28810=ORIENTED_EDGE('',*,*,#22231,.F.);
#28811=ORIENTED_EDGE('',*,*,#22125,.F.);
#28812=ORIENTED_EDGE('',*,*,#22271,.F.);
#28813=ORIENTED_EDGE('',*,*,#21753,.F.);
#28814=ORIENTED_EDGE('',*,*,#22234,.F.);
#28815=ORIENTED_EDGE('',*,*,#22132,.F.);
#28816=ORIENTED_EDGE('',*,*,#22270,.F.);
#28817=ORIENTED_EDGE('',*,*,#22278,.T.);
#28818=ORIENTED_EDGE('',*,*,#21864,.T.);
#28819=ORIENTED_EDGE('',*,*,#22279,.F.);
#28820=ORIENTED_EDGE('',*,*,#21891,.F.);
#28821=ORIENTED_EDGE('',*,*,#22280,.T.);
#28822=ORIENTED_EDGE('',*,*,#21865,.T.);
#28823=ORIENTED_EDGE('',*,*,#22278,.F.);
#28824=ORIENTED_EDGE('',*,*,#21890,.F.);
#28825=ORIENTED_EDGE('',*,*,#22281,.T.);
#28826=ORIENTED_EDGE('',*,*,#21866,.T.);
#28827=ORIENTED_EDGE('',*,*,#22280,.F.);
#28828=ORIENTED_EDGE('',*,*,#21901,.F.);
#28829=ORIENTED_EDGE('',*,*,#22282,.T.);
#28830=ORIENTED_EDGE('',*,*,#21867,.T.);
#28831=ORIENTED_EDGE('',*,*,#22281,.F.);
#28832=ORIENTED_EDGE('',*,*,#21900,.F.);
#28833=ORIENTED_EDGE('',*,*,#22283,.T.);
#28834=ORIENTED_EDGE('',*,*,#21868,.T.);
#28835=ORIENTED_EDGE('',*,*,#22282,.F.);
#28836=ORIENTED_EDGE('',*,*,#21899,.F.);
#28837=ORIENTED_EDGE('',*,*,#22284,.T.);
#28838=ORIENTED_EDGE('',*,*,#21869,.T.);
#28839=ORIENTED_EDGE('',*,*,#22283,.F.);
#28840=ORIENTED_EDGE('',*,*,#21898,.F.);
#28841=ORIENTED_EDGE('',*,*,#22285,.T.);
#28842=ORIENTED_EDGE('',*,*,#21870,.T.);
#28843=ORIENTED_EDGE('',*,*,#22284,.F.);
#28844=ORIENTED_EDGE('',*,*,#21897,.F.);
#28845=ORIENTED_EDGE('',*,*,#22286,.T.);
#28846=ORIENTED_EDGE('',*,*,#21871,.T.);
#28847=ORIENTED_EDGE('',*,*,#22285,.F.);
#28848=ORIENTED_EDGE('',*,*,#21896,.F.);
#28849=ORIENTED_EDGE('',*,*,#22287,.T.);
#28850=ORIENTED_EDGE('',*,*,#21872,.T.);
#28851=ORIENTED_EDGE('',*,*,#22286,.F.);
#28852=ORIENTED_EDGE('',*,*,#21895,.F.);
#28853=ORIENTED_EDGE('',*,*,#22288,.T.);
#28854=ORIENTED_EDGE('',*,*,#21873,.T.);
#28855=ORIENTED_EDGE('',*,*,#22287,.F.);
#28856=ORIENTED_EDGE('',*,*,#21894,.F.);
#28857=ORIENTED_EDGE('',*,*,#22289,.T.);
#28858=ORIENTED_EDGE('',*,*,#21874,.T.);
#28859=ORIENTED_EDGE('',*,*,#22288,.F.);
#28860=ORIENTED_EDGE('',*,*,#21893,.F.);
#28861=ORIENTED_EDGE('',*,*,#22279,.T.);
#28862=ORIENTED_EDGE('',*,*,#21875,.T.);
#28863=ORIENTED_EDGE('',*,*,#22289,.F.);
#28864=ORIENTED_EDGE('',*,*,#21892,.F.);
#28865=ORIENTED_EDGE('',*,*,#22290,.T.);
#28866=ORIENTED_EDGE('',*,*,#21860,.T.);
#28867=ORIENTED_EDGE('',*,*,#22291,.F.);
#28868=ORIENTED_EDGE('',*,*,#21887,.F.);
#28869=ORIENTED_EDGE('',*,*,#22292,.T.);
#28870=ORIENTED_EDGE('',*,*,#21861,.T.);
#28871=ORIENTED_EDGE('',*,*,#22290,.F.);
#28872=ORIENTED_EDGE('',*,*,#21886,.F.);
#28873=ORIENTED_EDGE('',*,*,#22293,.T.);
#28874=ORIENTED_EDGE('',*,*,#21862,.T.);
#28875=ORIENTED_EDGE('',*,*,#22292,.F.);
#28876=ORIENTED_EDGE('',*,*,#21889,.F.);
#28877=ORIENTED_EDGE('',*,*,#22291,.T.);
#28878=ORIENTED_EDGE('',*,*,#21863,.T.);
#28879=ORIENTED_EDGE('',*,*,#22293,.F.);
#28880=ORIENTED_EDGE('',*,*,#21888,.F.);
#28881=ORIENTED_EDGE('',*,*,#21859,.F.);
#28882=ORIENTED_EDGE('',*,*,#21927,.F.);
#28883=ORIENTED_EDGE('',*,*,#21879,.F.);
#28884=ORIENTED_EDGE('',*,*,#21926,.F.);
#28885=ORIENTED_EDGE('',*,*,#21507,.F.);
#28886=ORIENTED_EDGE('',*,*,#21940,.F.);
#28887=ORIENTED_EDGE('',*,*,#21347,.F.);
#28888=ORIENTED_EDGE('',*,*,#21942,.F.);
#28889=ORIENTED_EDGE('',*,*,#21499,.F.);
#28890=ORIENTED_EDGE('',*,*,#21941,.F.);
#28891=ORIENTED_EDGE('',*,*,#21345,.F.);
#28892=ORIENTED_EDGE('',*,*,#21943,.F.);
#28893=ORIENTED_EDGE('',*,*,#21851,.F.);
#28894=ORIENTED_EDGE('',*,*,#21925,.F.);
#28895=ORIENTED_EDGE('',*,*,#21877,.F.);
#28896=ORIENTED_EDGE('',*,*,#21924,.F.);
#28897=ORIENTED_EDGE('',*,*,#22294,.T.);
#28898=ORIENTED_EDGE('',*,*,#21355,.T.);
#28899=ORIENTED_EDGE('',*,*,#21063,.F.);
#28900=ORIENTED_EDGE('',*,*,#21651,.F.);
#28901=ORIENTED_EDGE('',*,*,#21650,.T.);
#28902=ORIENTED_EDGE('',*,*,#22295,.T.);
#28903=ORIENTED_EDGE('',*,*,#21356,.F.);
#28904=ORIENTED_EDGE('',*,*,#22294,.F.);
#28905=ORIENTED_EDGE('',*,*,#21649,.T.);
#28906=ORIENTED_EDGE('',*,*,#21065,.T.);
#28907=ORIENTED_EDGE('',*,*,#21354,.F.);
#28908=ORIENTED_EDGE('',*,*,#22295,.F.);
#28909=ORIENTED_EDGE('',*,*,#21061,.T.);
#28910=ORIENTED_EDGE('',*,*,#21495,.T.);
#28911=ORIENTED_EDGE('',*,*,#22296,.F.);
#28912=ORIENTED_EDGE('',*,*,#21508,.F.);
#28913=ORIENTED_EDGE('',*,*,#21510,.T.);
#28914=ORIENTED_EDGE('',*,*,#22297,.T.);
#28915=ORIENTED_EDGE('',*,*,#21496,.F.);
#28916=ORIENTED_EDGE('',*,*,#21059,.F.);
#28917=ORIENTED_EDGE('',*,*,#22296,.T.);
#28918=ORIENTED_EDGE('',*,*,#21497,.T.);
#28919=ORIENTED_EDGE('',*,*,#22297,.F.);
#28920=ORIENTED_EDGE('',*,*,#21509,.F.);
#28921=ORIENTED_EDGE('',*,*,#21057,.T.);
#28922=ORIENTED_EDGE('',*,*,#21492,.T.);
#28923=ORIENTED_EDGE('',*,*,#22298,.F.);
#28924=ORIENTED_EDGE('',*,*,#21511,.F.);
#28925=ORIENTED_EDGE('',*,*,#21513,.T.);
#28926=ORIENTED_EDGE('',*,*,#22299,.T.);
#28927=ORIENTED_EDGE('',*,*,#21493,.F.);
#28928=ORIENTED_EDGE('',*,*,#21055,.F.);
#28929=ORIENTED_EDGE('',*,*,#22298,.T.);
#28930=ORIENTED_EDGE('',*,*,#21494,.T.);
#28931=ORIENTED_EDGE('',*,*,#22299,.F.);
#28932=ORIENTED_EDGE('',*,*,#21512,.F.);
#28933=ORIENTED_EDGE('',*,*,#22300,.T.);
#28934=ORIENTED_EDGE('',*,*,#21358,.T.);
#28935=ORIENTED_EDGE('',*,*,#21051,.F.);
#28936=ORIENTED_EDGE('',*,*,#21516,.F.);
#28937=ORIENTED_EDGE('',*,*,#21515,.T.);
#28938=ORIENTED_EDGE('',*,*,#22301,.T.);
#28939=ORIENTED_EDGE('',*,*,#21359,.F.);
#28940=ORIENTED_EDGE('',*,*,#22300,.F.);
#28941=ORIENTED_EDGE('',*,*,#21514,.T.);
#28942=ORIENTED_EDGE('',*,*,#21053,.T.);
#28943=ORIENTED_EDGE('',*,*,#21357,.F.);
#28944=ORIENTED_EDGE('',*,*,#22301,.F.);
#28945=ORIENTED_EDGE('',*,*,#21049,.T.);
#28946=ORIENTED_EDGE('',*,*,#21489,.T.);
#28947=ORIENTED_EDGE('',*,*,#22302,.F.);
#28948=ORIENTED_EDGE('',*,*,#21646,.F.);
#28949=ORIENTED_EDGE('',*,*,#21648,.T.);
#28950=ORIENTED_EDGE('',*,*,#22303,.T.);
#28951=ORIENTED_EDGE('',*,*,#21490,.F.);
#28952=ORIENTED_EDGE('',*,*,#21047,.F.);
#28953=ORIENTED_EDGE('',*,*,#22302,.T.);
#28954=ORIENTED_EDGE('',*,*,#21491,.T.);
#28955=ORIENTED_EDGE('',*,*,#22303,.F.);
#28956=ORIENTED_EDGE('',*,*,#21647,.F.);
#28957=ORIENTED_EDGE('',*,*,#22304,.T.);
#28958=ORIENTED_EDGE('',*,*,#21361,.T.);
#28959=ORIENTED_EDGE('',*,*,#21043,.F.);
#28960=ORIENTED_EDGE('',*,*,#21645,.F.);
#28961=ORIENTED_EDGE('',*,*,#21644,.T.);
#28962=ORIENTED_EDGE('',*,*,#22305,.T.);
#28963=ORIENTED_EDGE('',*,*,#21362,.F.);
#28964=ORIENTED_EDGE('',*,*,#22304,.F.);
#28965=ORIENTED_EDGE('',*,*,#21643,.T.);
#28966=ORIENTED_EDGE('',*,*,#21045,.T.);
#28967=ORIENTED_EDGE('',*,*,#21360,.F.);
#28968=ORIENTED_EDGE('',*,*,#22305,.F.);
#28969=ORIENTED_EDGE('',*,*,#22306,.T.);
#28970=ORIENTED_EDGE('',*,*,#21364,.T.);
#28971=ORIENTED_EDGE('',*,*,#21039,.F.);
#28972=ORIENTED_EDGE('',*,*,#21519,.F.);
#28973=ORIENTED_EDGE('',*,*,#21518,.T.);
#28974=ORIENTED_EDGE('',*,*,#22307,.T.);
#28975=ORIENTED_EDGE('',*,*,#21365,.F.);
#28976=ORIENTED_EDGE('',*,*,#22306,.F.);
#28977=ORIENTED_EDGE('',*,*,#21517,.T.);
#28978=ORIENTED_EDGE('',*,*,#21041,.T.);
#28979=ORIENTED_EDGE('',*,*,#21363,.F.);
#28980=ORIENTED_EDGE('',*,*,#22307,.F.);
#28981=ORIENTED_EDGE('',*,*,#21037,.T.);
#28982=ORIENTED_EDGE('',*,*,#21486,.T.);
#28983=ORIENTED_EDGE('',*,*,#22308,.F.);
#28984=ORIENTED_EDGE('',*,*,#21640,.F.);
#28985=ORIENTED_EDGE('',*,*,#21642,.T.);
#28986=ORIENTED_EDGE('',*,*,#22309,.T.);
#28987=ORIENTED_EDGE('',*,*,#21487,.F.);
#28988=ORIENTED_EDGE('',*,*,#21035,.F.);
#28989=ORIENTED_EDGE('',*,*,#22308,.T.);
#28990=ORIENTED_EDGE('',*,*,#21488,.T.);
#28991=ORIENTED_EDGE('',*,*,#22309,.F.);
#28992=ORIENTED_EDGE('',*,*,#21641,.F.);
#28993=ORIENTED_EDGE('',*,*,#21033,.T.);
#28994=ORIENTED_EDGE('',*,*,#21483,.T.);
#28995=ORIENTED_EDGE('',*,*,#22310,.F.);
#28996=ORIENTED_EDGE('',*,*,#21637,.F.);
#28997=ORIENTED_EDGE('',*,*,#21639,.T.);
#28998=ORIENTED_EDGE('',*,*,#22311,.T.);
#28999=ORIENTED_EDGE('',*,*,#21484,.F.);
#29000=ORIENTED_EDGE('',*,*,#21031,.F.);
#29001=ORIENTED_EDGE('',*,*,#22310,.T.);
#29002=ORIENTED_EDGE('',*,*,#21485,.T.);
#29003=ORIENTED_EDGE('',*,*,#22311,.F.);
#29004=ORIENTED_EDGE('',*,*,#21638,.F.);
#29005=ORIENTED_EDGE('',*,*,#21029,.T.);
#29006=ORIENTED_EDGE('',*,*,#21480,.T.);
#29007=ORIENTED_EDGE('',*,*,#22312,.F.);
#29008=ORIENTED_EDGE('',*,*,#21634,.F.);
#29009=ORIENTED_EDGE('',*,*,#21636,.T.);
#29010=ORIENTED_EDGE('',*,*,#22313,.T.);
#29011=ORIENTED_EDGE('',*,*,#21481,.F.);
#29012=ORIENTED_EDGE('',*,*,#21027,.F.);
#29013=ORIENTED_EDGE('',*,*,#22312,.T.);
#29014=ORIENTED_EDGE('',*,*,#21482,.T.);
#29015=ORIENTED_EDGE('',*,*,#22313,.F.);
#29016=ORIENTED_EDGE('',*,*,#21635,.F.);
#29017=ORIENTED_EDGE('',*,*,#21025,.T.);
#29018=ORIENTED_EDGE('',*,*,#21477,.T.);
#29019=ORIENTED_EDGE('',*,*,#22314,.F.);
#29020=ORIENTED_EDGE('',*,*,#21631,.F.);
#29021=ORIENTED_EDGE('',*,*,#21633,.T.);
#29022=ORIENTED_EDGE('',*,*,#22315,.T.);
#29023=ORIENTED_EDGE('',*,*,#21478,.F.);
#29024=ORIENTED_EDGE('',*,*,#21023,.F.);
#29025=ORIENTED_EDGE('',*,*,#22314,.T.);
#29026=ORIENTED_EDGE('',*,*,#21479,.T.);
#29027=ORIENTED_EDGE('',*,*,#22315,.F.);
#29028=ORIENTED_EDGE('',*,*,#21632,.F.);
#29029=ORIENTED_EDGE('',*,*,#22316,.T.);
#29030=ORIENTED_EDGE('',*,*,#21367,.T.);
#29031=ORIENTED_EDGE('',*,*,#21019,.F.);
#29032=ORIENTED_EDGE('',*,*,#21630,.F.);
#29033=ORIENTED_EDGE('',*,*,#21629,.T.);
#29034=ORIENTED_EDGE('',*,*,#22317,.T.);
#29035=ORIENTED_EDGE('',*,*,#21368,.F.);
#29036=ORIENTED_EDGE('',*,*,#22316,.F.);
#29037=ORIENTED_EDGE('',*,*,#21628,.T.);
#29038=ORIENTED_EDGE('',*,*,#21021,.T.);
#29039=ORIENTED_EDGE('',*,*,#21366,.F.);
#29040=ORIENTED_EDGE('',*,*,#22317,.F.);
#29041=ORIENTED_EDGE('',*,*,#22318,.T.);
#29042=ORIENTED_EDGE('',*,*,#21370,.T.);
#29043=ORIENTED_EDGE('',*,*,#21015,.F.);
#29044=ORIENTED_EDGE('',*,*,#21522,.F.);
#29045=ORIENTED_EDGE('',*,*,#21521,.T.);
#29046=ORIENTED_EDGE('',*,*,#22319,.T.);
#29047=ORIENTED_EDGE('',*,*,#21371,.F.);
#29048=ORIENTED_EDGE('',*,*,#22318,.F.);
#29049=ORIENTED_EDGE('',*,*,#21520,.T.);
#29050=ORIENTED_EDGE('',*,*,#21017,.T.);
#29051=ORIENTED_EDGE('',*,*,#21369,.F.);
#29052=ORIENTED_EDGE('',*,*,#22319,.F.);
#29053=ORIENTED_EDGE('',*,*,#22320,.T.);
#29054=ORIENTED_EDGE('',*,*,#21373,.T.);
#29055=ORIENTED_EDGE('',*,*,#21011,.F.);
#29056=ORIENTED_EDGE('',*,*,#21627,.F.);
#29057=ORIENTED_EDGE('',*,*,#21626,.T.);
#29058=ORIENTED_EDGE('',*,*,#22321,.T.);
#29059=ORIENTED_EDGE('',*,*,#21374,.F.);
#29060=ORIENTED_EDGE('',*,*,#22320,.F.);
#29061=ORIENTED_EDGE('',*,*,#21625,.T.);
#29062=ORIENTED_EDGE('',*,*,#21013,.T.);
#29063=ORIENTED_EDGE('',*,*,#21372,.F.);
#29064=ORIENTED_EDGE('',*,*,#22321,.F.);
#29065=ORIENTED_EDGE('',*,*,#22322,.T.);
#29066=ORIENTED_EDGE('',*,*,#21376,.T.);
#29067=ORIENTED_EDGE('',*,*,#21007,.F.);
#29068=ORIENTED_EDGE('',*,*,#21525,.F.);
#29069=ORIENTED_EDGE('',*,*,#21524,.T.);
#29070=ORIENTED_EDGE('',*,*,#22323,.T.);
#29071=ORIENTED_EDGE('',*,*,#21377,.F.);
#29072=ORIENTED_EDGE('',*,*,#22322,.F.);
#29073=ORIENTED_EDGE('',*,*,#21523,.T.);
#29074=ORIENTED_EDGE('',*,*,#21009,.T.);
#29075=ORIENTED_EDGE('',*,*,#21375,.F.);
#29076=ORIENTED_EDGE('',*,*,#22323,.F.);
#29077=ORIENTED_EDGE('',*,*,#22324,.T.);
#29078=ORIENTED_EDGE('',*,*,#21379,.T.);
#29079=ORIENTED_EDGE('',*,*,#21003,.F.);
#29080=ORIENTED_EDGE('',*,*,#21624,.F.);
#29081=ORIENTED_EDGE('',*,*,#21623,.T.);
#29082=ORIENTED_EDGE('',*,*,#22325,.T.);
#29083=ORIENTED_EDGE('',*,*,#21380,.F.);
#29084=ORIENTED_EDGE('',*,*,#22324,.F.);
#29085=ORIENTED_EDGE('',*,*,#21622,.T.);
#29086=ORIENTED_EDGE('',*,*,#21005,.T.);
#29087=ORIENTED_EDGE('',*,*,#21378,.F.);
#29088=ORIENTED_EDGE('',*,*,#22325,.F.);
#29089=ORIENTED_EDGE('',*,*,#22326,.T.);
#29090=ORIENTED_EDGE('',*,*,#21382,.T.);
#29091=ORIENTED_EDGE('',*,*,#20999,.F.);
#29092=ORIENTED_EDGE('',*,*,#21528,.F.);
#29093=ORIENTED_EDGE('',*,*,#21527,.T.);
#29094=ORIENTED_EDGE('',*,*,#22327,.T.);
#29095=ORIENTED_EDGE('',*,*,#21383,.F.);
#29096=ORIENTED_EDGE('',*,*,#22326,.F.);
#29097=ORIENTED_EDGE('',*,*,#21526,.T.);
#29098=ORIENTED_EDGE('',*,*,#21001,.T.);
#29099=ORIENTED_EDGE('',*,*,#21381,.F.);
#29100=ORIENTED_EDGE('',*,*,#22327,.F.);
#29101=ORIENTED_EDGE('',*,*,#22328,.T.);
#29102=ORIENTED_EDGE('',*,*,#21385,.T.);
#29103=ORIENTED_EDGE('',*,*,#20995,.F.);
#29104=ORIENTED_EDGE('',*,*,#21621,.F.);
#29105=ORIENTED_EDGE('',*,*,#21620,.T.);
#29106=ORIENTED_EDGE('',*,*,#22329,.T.);
#29107=ORIENTED_EDGE('',*,*,#21386,.F.);
#29108=ORIENTED_EDGE('',*,*,#22328,.F.);
#29109=ORIENTED_EDGE('',*,*,#21619,.T.);
#29110=ORIENTED_EDGE('',*,*,#20997,.T.);
#29111=ORIENTED_EDGE('',*,*,#21384,.F.);
#29112=ORIENTED_EDGE('',*,*,#22329,.F.);
#29113=ORIENTED_EDGE('',*,*,#20993,.T.);
#29114=ORIENTED_EDGE('',*,*,#21474,.T.);
#29115=ORIENTED_EDGE('',*,*,#22330,.F.);
#29116=ORIENTED_EDGE('',*,*,#21529,.F.);
#29117=ORIENTED_EDGE('',*,*,#21531,.T.);
#29118=ORIENTED_EDGE('',*,*,#22331,.T.);
#29119=ORIENTED_EDGE('',*,*,#21475,.F.);
#29120=ORIENTED_EDGE('',*,*,#20991,.F.);
#29121=ORIENTED_EDGE('',*,*,#22330,.T.);
#29122=ORIENTED_EDGE('',*,*,#21476,.T.);
#29123=ORIENTED_EDGE('',*,*,#22331,.F.);
#29124=ORIENTED_EDGE('',*,*,#21530,.F.);
#29125=ORIENTED_EDGE('',*,*,#20989,.T.);
#29126=ORIENTED_EDGE('',*,*,#21471,.T.);
#29127=ORIENTED_EDGE('',*,*,#22332,.F.);
#29128=ORIENTED_EDGE('',*,*,#21532,.F.);
#29129=ORIENTED_EDGE('',*,*,#21534,.T.);
#29130=ORIENTED_EDGE('',*,*,#22333,.T.);
#29131=ORIENTED_EDGE('',*,*,#21472,.F.);
#29132=ORIENTED_EDGE('',*,*,#20987,.F.);
#29133=ORIENTED_EDGE('',*,*,#22332,.T.);
#29134=ORIENTED_EDGE('',*,*,#21473,.T.);
#29135=ORIENTED_EDGE('',*,*,#22333,.F.);
#29136=ORIENTED_EDGE('',*,*,#21533,.F.);
#29137=ORIENTED_EDGE('',*,*,#20985,.T.);
#29138=ORIENTED_EDGE('',*,*,#21468,.T.);
#29139=ORIENTED_EDGE('',*,*,#22334,.F.);
#29140=ORIENTED_EDGE('',*,*,#21535,.F.);
#29141=ORIENTED_EDGE('',*,*,#21537,.T.);
#29142=ORIENTED_EDGE('',*,*,#22335,.T.);
#29143=ORIENTED_EDGE('',*,*,#21469,.F.);
#29144=ORIENTED_EDGE('',*,*,#20983,.F.);
#29145=ORIENTED_EDGE('',*,*,#22334,.T.);
#29146=ORIENTED_EDGE('',*,*,#21470,.T.);
#29147=ORIENTED_EDGE('',*,*,#22335,.F.);
#29148=ORIENTED_EDGE('',*,*,#21536,.F.);
#29149=ORIENTED_EDGE('',*,*,#20981,.T.);
#29150=ORIENTED_EDGE('',*,*,#21465,.T.);
#29151=ORIENTED_EDGE('',*,*,#22336,.F.);
#29152=ORIENTED_EDGE('',*,*,#21538,.F.);
#29153=ORIENTED_EDGE('',*,*,#21540,.T.);
#29154=ORIENTED_EDGE('',*,*,#22337,.T.);
#29155=ORIENTED_EDGE('',*,*,#21466,.F.);
#29156=ORIENTED_EDGE('',*,*,#20979,.F.);
#29157=ORIENTED_EDGE('',*,*,#22336,.T.);
#29158=ORIENTED_EDGE('',*,*,#21467,.T.);
#29159=ORIENTED_EDGE('',*,*,#22337,.F.);
#29160=ORIENTED_EDGE('',*,*,#21539,.F.);
#29161=ORIENTED_EDGE('',*,*,#20977,.T.);
#29162=ORIENTED_EDGE('',*,*,#21462,.T.);
#29163=ORIENTED_EDGE('',*,*,#22338,.F.);
#29164=ORIENTED_EDGE('',*,*,#21541,.F.);
#29165=ORIENTED_EDGE('',*,*,#21543,.T.);
#29166=ORIENTED_EDGE('',*,*,#22339,.T.);
#29167=ORIENTED_EDGE('',*,*,#21463,.F.);
#29168=ORIENTED_EDGE('',*,*,#20975,.F.);
#29169=ORIENTED_EDGE('',*,*,#22338,.T.);
#29170=ORIENTED_EDGE('',*,*,#21464,.T.);
#29171=ORIENTED_EDGE('',*,*,#22339,.F.);
#29172=ORIENTED_EDGE('',*,*,#21542,.F.);
#29173=ORIENTED_EDGE('',*,*,#22340,.T.);
#29174=ORIENTED_EDGE('',*,*,#21388,.T.);
#29175=ORIENTED_EDGE('',*,*,#20971,.F.);
#29176=ORIENTED_EDGE('',*,*,#21546,.F.);
#29177=ORIENTED_EDGE('',*,*,#21545,.T.);
#29178=ORIENTED_EDGE('',*,*,#22341,.T.);
#29179=ORIENTED_EDGE('',*,*,#21389,.F.);
#29180=ORIENTED_EDGE('',*,*,#22340,.F.);
#29181=ORIENTED_EDGE('',*,*,#21544,.T.);
#29182=ORIENTED_EDGE('',*,*,#20973,.T.);
#29183=ORIENTED_EDGE('',*,*,#21387,.F.);
#29184=ORIENTED_EDGE('',*,*,#22341,.F.);
#29185=ORIENTED_EDGE('',*,*,#22342,.T.);
#29186=ORIENTED_EDGE('',*,*,#21459,.T.);
#29187=ORIENTED_EDGE('',*,*,#20967,.F.);
#29188=ORIENTED_EDGE('',*,*,#21616,.F.);
#29189=ORIENTED_EDGE('',*,*,#22343,.T.);
#29190=ORIENTED_EDGE('',*,*,#21460,.T.);
#29191=ORIENTED_EDGE('',*,*,#22342,.F.);
#29192=ORIENTED_EDGE('',*,*,#21618,.F.);
#29193=ORIENTED_EDGE('',*,*,#21617,.T.);
#29194=ORIENTED_EDGE('',*,*,#20969,.T.);
#29195=ORIENTED_EDGE('',*,*,#21461,.F.);
#29196=ORIENTED_EDGE('',*,*,#22343,.F.);
#29197=ORIENTED_EDGE('',*,*,#21613,.T.);
#29198=ORIENTED_EDGE('',*,*,#22344,.T.);
#29199=ORIENTED_EDGE('',*,*,#21390,.F.);
#29200=ORIENTED_EDGE('',*,*,#20963,.F.);
#29201=ORIENTED_EDGE('',*,*,#21615,.T.);
#29202=ORIENTED_EDGE('',*,*,#22345,.T.);
#29203=ORIENTED_EDGE('',*,*,#21391,.F.);
#29204=ORIENTED_EDGE('',*,*,#22344,.F.);
#29205=ORIENTED_EDGE('',*,*,#20965,.T.);
#29206=ORIENTED_EDGE('',*,*,#21392,.T.);
#29207=ORIENTED_EDGE('',*,*,#22345,.F.);
#29208=ORIENTED_EDGE('',*,*,#21614,.F.);
#29209=ORIENTED_EDGE('',*,*,#21547,.T.);
#29210=ORIENTED_EDGE('',*,*,#22346,.T.);
#29211=ORIENTED_EDGE('',*,*,#21393,.F.);
#29212=ORIENTED_EDGE('',*,*,#20959,.F.);
#29213=ORIENTED_EDGE('',*,*,#21549,.T.);
#29214=ORIENTED_EDGE('',*,*,#22347,.T.);
#29215=ORIENTED_EDGE('',*,*,#21394,.F.);
#29216=ORIENTED_EDGE('',*,*,#22346,.F.);
#29217=ORIENTED_EDGE('',*,*,#20961,.T.);
#29218=ORIENTED_EDGE('',*,*,#21395,.T.);
#29219=ORIENTED_EDGE('',*,*,#22347,.F.);
#29220=ORIENTED_EDGE('',*,*,#21548,.F.);
#29221=ORIENTED_EDGE('',*,*,#22348,.T.);
#29222=ORIENTED_EDGE('',*,*,#21456,.T.);
#29223=ORIENTED_EDGE('',*,*,#20955,.F.);
#29224=ORIENTED_EDGE('',*,*,#21610,.F.);
#29225=ORIENTED_EDGE('',*,*,#22349,.T.);
#29226=ORIENTED_EDGE('',*,*,#21457,.T.);
#29227=ORIENTED_EDGE('',*,*,#22348,.F.);
#29228=ORIENTED_EDGE('',*,*,#21612,.F.);
#29229=ORIENTED_EDGE('',*,*,#21611,.T.);
#29230=ORIENTED_EDGE('',*,*,#20957,.T.);
#29231=ORIENTED_EDGE('',*,*,#21458,.F.);
#29232=ORIENTED_EDGE('',*,*,#22349,.F.);
#29233=ORIENTED_EDGE('',*,*,#21607,.T.);
#29234=ORIENTED_EDGE('',*,*,#22350,.T.);
#29235=ORIENTED_EDGE('',*,*,#21396,.F.);
#29236=ORIENTED_EDGE('',*,*,#20951,.F.);
#29237=ORIENTED_EDGE('',*,*,#21609,.T.);
#29238=ORIENTED_EDGE('',*,*,#22351,.T.);
#29239=ORIENTED_EDGE('',*,*,#21397,.F.);
#29240=ORIENTED_EDGE('',*,*,#22350,.F.);
#29241=ORIENTED_EDGE('',*,*,#20953,.T.);
#29242=ORIENTED_EDGE('',*,*,#21398,.T.);
#29243=ORIENTED_EDGE('',*,*,#22351,.F.);
#29244=ORIENTED_EDGE('',*,*,#21608,.F.);
#29245=ORIENTED_EDGE('',*,*,#22352,.T.);
#29246=ORIENTED_EDGE('',*,*,#21453,.T.);
#29247=ORIENTED_EDGE('',*,*,#20947,.F.);
#29248=ORIENTED_EDGE('',*,*,#21550,.F.);
#29249=ORIENTED_EDGE('',*,*,#22353,.T.);
#29250=ORIENTED_EDGE('',*,*,#21454,.T.);
#29251=ORIENTED_EDGE('',*,*,#22352,.F.);
#29252=ORIENTED_EDGE('',*,*,#21552,.F.);
#29253=ORIENTED_EDGE('',*,*,#21551,.T.);
#29254=ORIENTED_EDGE('',*,*,#20949,.T.);
#29255=ORIENTED_EDGE('',*,*,#21455,.F.);
#29256=ORIENTED_EDGE('',*,*,#22353,.F.);
#29257=ORIENTED_EDGE('',*,*,#22354,.T.);
#29258=ORIENTED_EDGE('',*,*,#21450,.T.);
#29259=ORIENTED_EDGE('',*,*,#20943,.F.);
#29260=ORIENTED_EDGE('',*,*,#21553,.F.);
#29261=ORIENTED_EDGE('',*,*,#22355,.T.);
#29262=ORIENTED_EDGE('',*,*,#21451,.T.);
#29263=ORIENTED_EDGE('',*,*,#22354,.F.);
#29264=ORIENTED_EDGE('',*,*,#21555,.F.);
#29265=ORIENTED_EDGE('',*,*,#21554,.T.);
#29266=ORIENTED_EDGE('',*,*,#20945,.T.);
#29267=ORIENTED_EDGE('',*,*,#21452,.F.);
#29268=ORIENTED_EDGE('',*,*,#22355,.F.);
#29269=ORIENTED_EDGE('',*,*,#21556,.T.);
#29270=ORIENTED_EDGE('',*,*,#22356,.T.);
#29271=ORIENTED_EDGE('',*,*,#21399,.F.);
#29272=ORIENTED_EDGE('',*,*,#20939,.F.);
#29273=ORIENTED_EDGE('',*,*,#21558,.T.);
#29274=ORIENTED_EDGE('',*,*,#22357,.T.);
#29275=ORIENTED_EDGE('',*,*,#21400,.F.);
#29276=ORIENTED_EDGE('',*,*,#22356,.F.);
#29277=ORIENTED_EDGE('',*,*,#20941,.T.);
#29278=ORIENTED_EDGE('',*,*,#21401,.T.);
#29279=ORIENTED_EDGE('',*,*,#22357,.F.);
#29280=ORIENTED_EDGE('',*,*,#21557,.F.);
#29281=ORIENTED_EDGE('',*,*,#21604,.T.);
#29282=ORIENTED_EDGE('',*,*,#22358,.T.);
#29283=ORIENTED_EDGE('',*,*,#21402,.F.);
#29284=ORIENTED_EDGE('',*,*,#20935,.F.);
#29285=ORIENTED_EDGE('',*,*,#21606,.T.);
#29286=ORIENTED_EDGE('',*,*,#22359,.T.);
#29287=ORIENTED_EDGE('',*,*,#21403,.F.);
#29288=ORIENTED_EDGE('',*,*,#22358,.F.);
#29289=ORIENTED_EDGE('',*,*,#20937,.T.);
#29290=ORIENTED_EDGE('',*,*,#21404,.T.);
#29291=ORIENTED_EDGE('',*,*,#22359,.F.);
#29292=ORIENTED_EDGE('',*,*,#21605,.F.);
#29293=ORIENTED_EDGE('',*,*,#21559,.T.);
#29294=ORIENTED_EDGE('',*,*,#22360,.T.);
#29295=ORIENTED_EDGE('',*,*,#21405,.F.);
#29296=ORIENTED_EDGE('',*,*,#20931,.F.);
#29297=ORIENTED_EDGE('',*,*,#21561,.T.);
#29298=ORIENTED_EDGE('',*,*,#22361,.T.);
#29299=ORIENTED_EDGE('',*,*,#21406,.F.);
#29300=ORIENTED_EDGE('',*,*,#22360,.F.);
#29301=ORIENTED_EDGE('',*,*,#20933,.T.);
#29302=ORIENTED_EDGE('',*,*,#21407,.T.);
#29303=ORIENTED_EDGE('',*,*,#22361,.F.);
#29304=ORIENTED_EDGE('',*,*,#21560,.F.);
#29305=ORIENTED_EDGE('',*,*,#21601,.T.);
#29306=ORIENTED_EDGE('',*,*,#22362,.T.);
#29307=ORIENTED_EDGE('',*,*,#21408,.F.);
#29308=ORIENTED_EDGE('',*,*,#20927,.F.);
#29309=ORIENTED_EDGE('',*,*,#21603,.T.);
#29310=ORIENTED_EDGE('',*,*,#22363,.T.);
#29311=ORIENTED_EDGE('',*,*,#21409,.F.);
#29312=ORIENTED_EDGE('',*,*,#22362,.F.);
#29313=ORIENTED_EDGE('',*,*,#20929,.T.);
#29314=ORIENTED_EDGE('',*,*,#21410,.T.);
#29315=ORIENTED_EDGE('',*,*,#22363,.F.);
#29316=ORIENTED_EDGE('',*,*,#21602,.F.);
#29317=ORIENTED_EDGE('',*,*,#22364,.T.);
#29318=ORIENTED_EDGE('',*,*,#21447,.T.);
#29319=ORIENTED_EDGE('',*,*,#20923,.F.);
#29320=ORIENTED_EDGE('',*,*,#21562,.F.);
#29321=ORIENTED_EDGE('',*,*,#22365,.T.);
#29322=ORIENTED_EDGE('',*,*,#21448,.T.);
#29323=ORIENTED_EDGE('',*,*,#22364,.F.);
#29324=ORIENTED_EDGE('',*,*,#21564,.F.);
#29325=ORIENTED_EDGE('',*,*,#21563,.T.);
#29326=ORIENTED_EDGE('',*,*,#20925,.T.);
#29327=ORIENTED_EDGE('',*,*,#21449,.F.);
#29328=ORIENTED_EDGE('',*,*,#22365,.F.);
#29329=ORIENTED_EDGE('',*,*,#22366,.T.);
#29330=ORIENTED_EDGE('',*,*,#21444,.T.);
#29331=ORIENTED_EDGE('',*,*,#20919,.F.);
#29332=ORIENTED_EDGE('',*,*,#21565,.F.);
#29333=ORIENTED_EDGE('',*,*,#22367,.T.);
#29334=ORIENTED_EDGE('',*,*,#21445,.T.);
#29335=ORIENTED_EDGE('',*,*,#22366,.F.);
#29336=ORIENTED_EDGE('',*,*,#21567,.F.);
#29337=ORIENTED_EDGE('',*,*,#21566,.T.);
#29338=ORIENTED_EDGE('',*,*,#20921,.T.);
#29339=ORIENTED_EDGE('',*,*,#21446,.F.);
#29340=ORIENTED_EDGE('',*,*,#22367,.F.);
#29341=ORIENTED_EDGE('',*,*,#22368,.T.);
#29342=ORIENTED_EDGE('',*,*,#21441,.T.);
#29343=ORIENTED_EDGE('',*,*,#20915,.F.);
#29344=ORIENTED_EDGE('',*,*,#21568,.F.);
#29345=ORIENTED_EDGE('',*,*,#22369,.T.);
#29346=ORIENTED_EDGE('',*,*,#21442,.T.);
#29347=ORIENTED_EDGE('',*,*,#22368,.F.);
#29348=ORIENTED_EDGE('',*,*,#21570,.F.);
#29349=ORIENTED_EDGE('',*,*,#21569,.T.);
#29350=ORIENTED_EDGE('',*,*,#20917,.T.);
#29351=ORIENTED_EDGE('',*,*,#21443,.F.);
#29352=ORIENTED_EDGE('',*,*,#22369,.F.);
#29353=ORIENTED_EDGE('',*,*,#22370,.T.);
#29354=ORIENTED_EDGE('',*,*,#21438,.T.);
#29355=ORIENTED_EDGE('',*,*,#20911,.F.);
#29356=ORIENTED_EDGE('',*,*,#21571,.F.);
#29357=ORIENTED_EDGE('',*,*,#22371,.T.);
#29358=ORIENTED_EDGE('',*,*,#21439,.T.);
#29359=ORIENTED_EDGE('',*,*,#22370,.F.);
#29360=ORIENTED_EDGE('',*,*,#21573,.F.);
#29361=ORIENTED_EDGE('',*,*,#21572,.T.);
#29362=ORIENTED_EDGE('',*,*,#20913,.T.);
#29363=ORIENTED_EDGE('',*,*,#21440,.F.);
#29364=ORIENTED_EDGE('',*,*,#22371,.F.);
#29365=ORIENTED_EDGE('',*,*,#22372,.T.);
#29366=ORIENTED_EDGE('',*,*,#21435,.T.);
#29367=ORIENTED_EDGE('',*,*,#20907,.F.);
#29368=ORIENTED_EDGE('',*,*,#21574,.F.);
#29369=ORIENTED_EDGE('',*,*,#22373,.T.);
#29370=ORIENTED_EDGE('',*,*,#21436,.T.);
#29371=ORIENTED_EDGE('',*,*,#22372,.F.);
#29372=ORIENTED_EDGE('',*,*,#21576,.F.);
#29373=ORIENTED_EDGE('',*,*,#21575,.T.);
#29374=ORIENTED_EDGE('',*,*,#20909,.T.);
#29375=ORIENTED_EDGE('',*,*,#21437,.F.);
#29376=ORIENTED_EDGE('',*,*,#22373,.F.);
#29377=ORIENTED_EDGE('',*,*,#22374,.T.);
#29378=ORIENTED_EDGE('',*,*,#21432,.T.);
#29379=ORIENTED_EDGE('',*,*,#20903,.F.);
#29380=ORIENTED_EDGE('',*,*,#21577,.F.);
#29381=ORIENTED_EDGE('',*,*,#22375,.T.);
#29382=ORIENTED_EDGE('',*,*,#21433,.T.);
#29383=ORIENTED_EDGE('',*,*,#22374,.F.);
#29384=ORIENTED_EDGE('',*,*,#21579,.F.);
#29385=ORIENTED_EDGE('',*,*,#21578,.T.);
#29386=ORIENTED_EDGE('',*,*,#20905,.T.);
#29387=ORIENTED_EDGE('',*,*,#21434,.F.);
#29388=ORIENTED_EDGE('',*,*,#22375,.F.);
#29389=ORIENTED_EDGE('',*,*,#22376,.T.);
#29390=ORIENTED_EDGE('',*,*,#21429,.T.);
#29391=ORIENTED_EDGE('',*,*,#20899,.F.);
#29392=ORIENTED_EDGE('',*,*,#21580,.F.);
#29393=ORIENTED_EDGE('',*,*,#22377,.T.);
#29394=ORIENTED_EDGE('',*,*,#21430,.T.);
#29395=ORIENTED_EDGE('',*,*,#22376,.F.);
#29396=ORIENTED_EDGE('',*,*,#21582,.F.);
#29397=ORIENTED_EDGE('',*,*,#21581,.T.);
#29398=ORIENTED_EDGE('',*,*,#20901,.T.);
#29399=ORIENTED_EDGE('',*,*,#21431,.F.);
#29400=ORIENTED_EDGE('',*,*,#22377,.F.);
#29401=ORIENTED_EDGE('',*,*,#21583,.T.);
#29402=ORIENTED_EDGE('',*,*,#22378,.T.);
#29403=ORIENTED_EDGE('',*,*,#21411,.F.);
#29404=ORIENTED_EDGE('',*,*,#20895,.F.);
#29405=ORIENTED_EDGE('',*,*,#21585,.T.);
#29406=ORIENTED_EDGE('',*,*,#22379,.T.);
#29407=ORIENTED_EDGE('',*,*,#21412,.F.);
#29408=ORIENTED_EDGE('',*,*,#22378,.F.);
#29409=ORIENTED_EDGE('',*,*,#20897,.T.);
#29410=ORIENTED_EDGE('',*,*,#21413,.T.);
#29411=ORIENTED_EDGE('',*,*,#22379,.F.);
#29412=ORIENTED_EDGE('',*,*,#21584,.F.);
#29413=ORIENTED_EDGE('',*,*,#21598,.T.);
#29414=ORIENTED_EDGE('',*,*,#22380,.T.);
#29415=ORIENTED_EDGE('',*,*,#21414,.F.);
#29416=ORIENTED_EDGE('',*,*,#20891,.F.);
#29417=ORIENTED_EDGE('',*,*,#21600,.T.);
#29418=ORIENTED_EDGE('',*,*,#22381,.T.);
#29419=ORIENTED_EDGE('',*,*,#21415,.F.);
#29420=ORIENTED_EDGE('',*,*,#22380,.F.);
#29421=ORIENTED_EDGE('',*,*,#20893,.T.);
#29422=ORIENTED_EDGE('',*,*,#21416,.T.);
#29423=ORIENTED_EDGE('',*,*,#22381,.F.);
#29424=ORIENTED_EDGE('',*,*,#21599,.F.);
#29425=ORIENTED_EDGE('',*,*,#21586,.T.);
#29426=ORIENTED_EDGE('',*,*,#22382,.T.);
#29427=ORIENTED_EDGE('',*,*,#21417,.F.);
#29428=ORIENTED_EDGE('',*,*,#20887,.F.);
#29429=ORIENTED_EDGE('',*,*,#21588,.T.);
#29430=ORIENTED_EDGE('',*,*,#22383,.T.);
#29431=ORIENTED_EDGE('',*,*,#21418,.F.);
#29432=ORIENTED_EDGE('',*,*,#22382,.F.);
#29433=ORIENTED_EDGE('',*,*,#20889,.T.);
#29434=ORIENTED_EDGE('',*,*,#21419,.T.);
#29435=ORIENTED_EDGE('',*,*,#22383,.F.);
#29436=ORIENTED_EDGE('',*,*,#21587,.F.);
#29437=ORIENTED_EDGE('',*,*,#21595,.T.);
#29438=ORIENTED_EDGE('',*,*,#22384,.T.);
#29439=ORIENTED_EDGE('',*,*,#21420,.F.);
#29440=ORIENTED_EDGE('',*,*,#20883,.F.);
#29441=ORIENTED_EDGE('',*,*,#21597,.T.);
#29442=ORIENTED_EDGE('',*,*,#22385,.T.);
#29443=ORIENTED_EDGE('',*,*,#21421,.F.);
#29444=ORIENTED_EDGE('',*,*,#22384,.F.);
#29445=ORIENTED_EDGE('',*,*,#20885,.T.);
#29446=ORIENTED_EDGE('',*,*,#21422,.T.);
#29447=ORIENTED_EDGE('',*,*,#22385,.F.);
#29448=ORIENTED_EDGE('',*,*,#21596,.F.);
#29449=ORIENTED_EDGE('',*,*,#21589,.T.);
#29450=ORIENTED_EDGE('',*,*,#22386,.T.);
#29451=ORIENTED_EDGE('',*,*,#21423,.F.);
#29452=ORIENTED_EDGE('',*,*,#20879,.F.);
#29453=ORIENTED_EDGE('',*,*,#21591,.T.);
#29454=ORIENTED_EDGE('',*,*,#22387,.T.);
#29455=ORIENTED_EDGE('',*,*,#21424,.F.);
#29456=ORIENTED_EDGE('',*,*,#22386,.F.);
#29457=ORIENTED_EDGE('',*,*,#20881,.T.);
#29458=ORIENTED_EDGE('',*,*,#21425,.T.);
#29459=ORIENTED_EDGE('',*,*,#22387,.F.);
#29460=ORIENTED_EDGE('',*,*,#21590,.F.);
#29461=ORIENTED_EDGE('',*,*,#22388,.T.);
#29462=ORIENTED_EDGE('',*,*,#21426,.T.);
#29463=ORIENTED_EDGE('',*,*,#20875,.F.);
#29464=ORIENTED_EDGE('',*,*,#21592,.F.);
#29465=ORIENTED_EDGE('',*,*,#22389,.T.);
#29466=ORIENTED_EDGE('',*,*,#21427,.T.);
#29467=ORIENTED_EDGE('',*,*,#22388,.F.);
#29468=ORIENTED_EDGE('',*,*,#21594,.F.);
#29469=ORIENTED_EDGE('',*,*,#21593,.T.);
#29470=ORIENTED_EDGE('',*,*,#20877,.T.);
#29471=ORIENTED_EDGE('',*,*,#21428,.F.);
#29472=ORIENTED_EDGE('',*,*,#22389,.F.);
#29473=ORIENTED_EDGE('',*,*,#21271,.F.);
#29474=ORIENTED_EDGE('',*,*,#21340,.F.);
#29475=ORIENTED_EDGE('',*,*,#21210,.T.);
#29476=ORIENTED_EDGE('',*,*,#22390,.T.);
#29477=ORIENTED_EDGE('',*,*,#21272,.F.);
#29478=ORIENTED_EDGE('',*,*,#22390,.F.);
#29479=ORIENTED_EDGE('',*,*,#21209,.T.);
#29480=ORIENTED_EDGE('',*,*,#22391,.T.);
#29481=ORIENTED_EDGE('',*,*,#21273,.F.);
#29482=ORIENTED_EDGE('',*,*,#22391,.F.);
#29483=ORIENTED_EDGE('',*,*,#21208,.T.);
#29484=ORIENTED_EDGE('',*,*,#22392,.T.);
#29485=ORIENTED_EDGE('',*,*,#21275,.F.);
#29486=ORIENTED_EDGE('',*,*,#22393,.F.);
#29487=ORIENTED_EDGE('',*,*,#21206,.T.);
#29488=ORIENTED_EDGE('',*,*,#22394,.T.);
#29489=ORIENTED_EDGE('',*,*,#21276,.F.);
#29490=ORIENTED_EDGE('',*,*,#22394,.F.);
#29491=ORIENTED_EDGE('',*,*,#21205,.T.);
#29492=ORIENTED_EDGE('',*,*,#22395,.T.);
#29493=ORIENTED_EDGE('',*,*,#21277,.F.);
#29494=ORIENTED_EDGE('',*,*,#22395,.F.);
#29495=ORIENTED_EDGE('',*,*,#21204,.T.);
#29496=ORIENTED_EDGE('',*,*,#21342,.T.);
#29497=ORIENTED_EDGE('',*,*,#22396,.F.);
#29498=ORIENTED_EDGE('',*,*,#22397,.F.);
#29499=ORIENTED_EDGE('',*,*,#22393,.T.);
#29500=ORIENTED_EDGE('',*,*,#22398,.T.);
#29501=ORIENTED_EDGE('',*,*,#22399,.F.);
#29502=ORIENTED_EDGE('',*,*,#22400,.T.);
#29503=ORIENTED_EDGE('',*,*,#22401,.T.);
#29504=ORIENTED_EDGE('',*,*,#22392,.F.);
#29505=ORIENTED_EDGE('',*,*,#21274,.F.);
#29506=ORIENTED_EDGE('',*,*,#22401,.F.);
#29507=ORIENTED_EDGE('',*,*,#21326,.T.);
#29508=ORIENTED_EDGE('',*,*,#22398,.F.);
#29509=ORIENTED_EDGE('',*,*,#21207,.T.);
#29510=ORIENTED_EDGE('',*,*,#22397,.T.);
#29511=ORIENTED_EDGE('',*,*,#21305,.T.);
#29512=ORIENTED_EDGE('',*,*,#22399,.T.);
#29513=ORIENTED_EDGE('',*,*,#22400,.F.);
#29514=ORIENTED_EDGE('',*,*,#21304,.T.);
#29515=ORIENTED_EDGE('',*,*,#22402,.F.);
#29516=ORIENTED_EDGE('',*,*,#21327,.F.);
#29517=ORIENTED_EDGE('',*,*,#22396,.T.);
#29518=ORIENTED_EDGE('',*,*,#21331,.F.);
#29519=ORIENTED_EDGE('',*,*,#22403,.T.);
#29520=ORIENTED_EDGE('',*,*,#21306,.T.);
#29521=ORIENTED_EDGE('',*,*,#21309,.T.);
#29522=ORIENTED_EDGE('',*,*,#22404,.F.);
#29523=ORIENTED_EDGE('',*,*,#21328,.F.);
#29524=ORIENTED_EDGE('',*,*,#22402,.T.);
#29525=ORIENTED_EDGE('',*,*,#21308,.T.);
#29526=ORIENTED_EDGE('',*,*,#22405,.F.);
#29527=ORIENTED_EDGE('',*,*,#21329,.F.);
#29528=ORIENTED_EDGE('',*,*,#22404,.T.);
#29529=ORIENTED_EDGE('',*,*,#21307,.T.);
#29530=ORIENTED_EDGE('',*,*,#22403,.F.);
#29531=ORIENTED_EDGE('',*,*,#21330,.F.);
#29532=ORIENTED_EDGE('',*,*,#22405,.T.);
#29533=ORIENTED_EDGE('',*,*,#22406,.F.);
#29534=ORIENTED_EDGE('',*,*,#21332,.T.);
#29535=ORIENTED_EDGE('',*,*,#22407,.F.);
#29536=ORIENTED_EDGE('',*,*,#21316,.F.);
#29537=ORIENTED_EDGE('',*,*,#21312,.T.);
#29538=ORIENTED_EDGE('',*,*,#22408,.F.);
#29539=ORIENTED_EDGE('',*,*,#21334,.F.);
#29540=ORIENTED_EDGE('',*,*,#22409,.F.);
#29541=ORIENTED_EDGE('',*,*,#22409,.T.);
#29542=ORIENTED_EDGE('',*,*,#21333,.T.);
#29543=ORIENTED_EDGE('',*,*,#22406,.T.);
#29544=ORIENTED_EDGE('',*,*,#22410,.T.);
#29545=ORIENTED_EDGE('',*,*,#22411,.T.);
#29546=ORIENTED_EDGE('',*,*,#22412,.T.);
#29547=ORIENTED_EDGE('',*,*,#22407,.T.);
#29548=ORIENTED_EDGE('',*,*,#21335,.T.);
#29549=ORIENTED_EDGE('',*,*,#22408,.T.);
#29550=ORIENTED_EDGE('',*,*,#22413,.T.);
#29551=ORIENTED_EDGE('',*,*,#22414,.T.);
#29552=ORIENTED_EDGE('',*,*,#22415,.T.);
#29553=ORIENTED_EDGE('',*,*,#21311,.F.);
#29554=ORIENTED_EDGE('',*,*,#22416,.T.);
#29555=ORIENTED_EDGE('',*,*,#22417,.T.);
#29556=ORIENTED_EDGE('',*,*,#22418,.T.);
#29557=ORIENTED_EDGE('',*,*,#22419,.T.);
#29558=ORIENTED_EDGE('',*,*,#22420,.T.);
#29559=ORIENTED_EDGE('',*,*,#22421,.T.);
#29560=ORIENTED_EDGE('',*,*,#22422,.T.);
#29561=ORIENTED_EDGE('',*,*,#21313,.F.);
#29562=ORIENTED_EDGE('',*,*,#22412,.F.);
#29563=ORIENTED_EDGE('',*,*,#22423,.F.);
#29564=ORIENTED_EDGE('',*,*,#22424,.F.);
#29565=ORIENTED_EDGE('',*,*,#22425,.F.);
#29566=ORIENTED_EDGE('',*,*,#22426,.F.);
#29567=ORIENTED_EDGE('',*,*,#22427,.F.);
#29568=ORIENTED_EDGE('',*,*,#22413,.F.);
#29569=ORIENTED_EDGE('',*,*,#21315,.F.);
#29570=ORIENTED_EDGE('',*,*,#22428,.T.);
#29571=ORIENTED_EDGE('',*,*,#22429,.F.);
#29572=ORIENTED_EDGE('',*,*,#22430,.T.);
#29573=ORIENTED_EDGE('',*,*,#22431,.F.);
#29574=ORIENTED_EDGE('',*,*,#22432,.T.);
#29575=ORIENTED_EDGE('',*,*,#22433,.F.);
#29576=ORIENTED_EDGE('',*,*,#22434,.T.);
#29577=ORIENTED_EDGE('',*,*,#21317,.F.);
#29578=ORIENTED_EDGE('',*,*,#22415,.F.);
#29579=ORIENTED_EDGE('',*,*,#22435,.T.);
#29580=ORIENTED_EDGE('',*,*,#22436,.F.);
#29581=ORIENTED_EDGE('',*,*,#22437,.T.);
#29582=ORIENTED_EDGE('',*,*,#22438,.F.);
#29583=ORIENTED_EDGE('',*,*,#22439,.T.);
#29584=ORIENTED_EDGE('',*,*,#22410,.F.);
#29585=ORIENTED_EDGE('',*,*,#22438,.T.);
#29586=ORIENTED_EDGE('',*,*,#22440,.T.);
#29587=ORIENTED_EDGE('',*,*,#22424,.T.);
#29588=ORIENTED_EDGE('',*,*,#22441,.T.);
#29589=ORIENTED_EDGE('',*,*,#22436,.T.);
#29590=ORIENTED_EDGE('',*,*,#22442,.T.);
#29591=ORIENTED_EDGE('',*,*,#22426,.T.);
#29592=ORIENTED_EDGE('',*,*,#22443,.T.);
#29593=ORIENTED_EDGE('',*,*,#22423,.T.);
#29594=ORIENTED_EDGE('',*,*,#22411,.F.);
#29595=ORIENTED_EDGE('',*,*,#22439,.F.);
#29596=ORIENTED_EDGE('',*,*,#22441,.F.);
#29597=ORIENTED_EDGE('',*,*,#22435,.F.);
#29598=ORIENTED_EDGE('',*,*,#22414,.F.);
#29599=ORIENTED_EDGE('',*,*,#22427,.T.);
#29600=ORIENTED_EDGE('',*,*,#22442,.F.);
#29601=ORIENTED_EDGE('',*,*,#22425,.T.);
#29602=ORIENTED_EDGE('',*,*,#22440,.F.);
#29603=ORIENTED_EDGE('',*,*,#22437,.F.);
#29604=ORIENTED_EDGE('',*,*,#22443,.F.);
#29605=ORIENTED_EDGE('',*,*,#20871,.F.);
#29606=ORIENTED_EDGE('',*,*,#22430,.F.);
#29607=ORIENTED_EDGE('',*,*,#22444,.F.);
#29608=ORIENTED_EDGE('',*,*,#22420,.F.);
#29609=ORIENTED_EDGE('',*,*,#22445,.F.);
#29610=ORIENTED_EDGE('',*,*,#22432,.F.);
#29611=ORIENTED_EDGE('',*,*,#22446,.F.);
#29612=ORIENTED_EDGE('',*,*,#22418,.F.);
#29613=ORIENTED_EDGE('',*,*,#22447,.F.);
#29614=ORIENTED_EDGE('',*,*,#22434,.F.);
#29615=ORIENTED_EDGE('',*,*,#22448,.F.);
#29616=ORIENTED_EDGE('',*,*,#22416,.F.);
#29617=ORIENTED_EDGE('',*,*,#21310,.F.);
#29618=ORIENTED_EDGE('',*,*,#22428,.F.);
#29619=ORIENTED_EDGE('',*,*,#21314,.F.);
#29620=ORIENTED_EDGE('',*,*,#22422,.F.);
#29621=ORIENTED_EDGE('',*,*,#22449,.F.);
#29622=ORIENTED_EDGE('',*,*,#22421,.F.);
#29623=ORIENTED_EDGE('',*,*,#22444,.T.);
#29624=ORIENTED_EDGE('',*,*,#22429,.T.);
#29625=ORIENTED_EDGE('',*,*,#22449,.T.);
#29626=ORIENTED_EDGE('',*,*,#22433,.T.);
#29627=ORIENTED_EDGE('',*,*,#22447,.T.);
#29628=ORIENTED_EDGE('',*,*,#22417,.F.);
#29629=ORIENTED_EDGE('',*,*,#22448,.T.);
#29630=ORIENTED_EDGE('',*,*,#22419,.F.);
#29631=ORIENTED_EDGE('',*,*,#22446,.T.);
#29632=ORIENTED_EDGE('',*,*,#22431,.T.);
#29633=ORIENTED_EDGE('',*,*,#22445,.T.);
#29634=ORIENTED_EDGE('',*,*,#20873,.T.);
#29635=ORIENTED_EDGE('',*,*,#22450,.T.);
#29636=ORIENTED_EDGE('',*,*,#21337,.F.);
#29637=ORIENTED_EDGE('',*,*,#22451,.T.);
#29638=ORIENTED_EDGE('',*,*,#21324,.F.);
#29639=ORIENTED_EDGE('',*,*,#21320,.T.);
#29640=ORIENTED_EDGE('',*,*,#22452,.T.);
#29641=ORIENTED_EDGE('',*,*,#21339,.T.);
#29642=ORIENTED_EDGE('',*,*,#22453,.T.);
#29643=ORIENTED_EDGE('',*,*,#22451,.F.);
#29644=ORIENTED_EDGE('',*,*,#21336,.F.);
#29645=ORIENTED_EDGE('',*,*,#22452,.F.);
#29646=ORIENTED_EDGE('',*,*,#22454,.F.);
#29647=ORIENTED_EDGE('',*,*,#22455,.F.);
#29648=ORIENTED_EDGE('',*,*,#22456,.F.);
#29649=ORIENTED_EDGE('',*,*,#22453,.F.);
#29650=ORIENTED_EDGE('',*,*,#21338,.F.);
#29651=ORIENTED_EDGE('',*,*,#22450,.F.);
#29652=ORIENTED_EDGE('',*,*,#22457,.F.);
#29653=ORIENTED_EDGE('',*,*,#22458,.F.);
#29654=ORIENTED_EDGE('',*,*,#22459,.F.);
#29655=ORIENTED_EDGE('',*,*,#21319,.F.);
#29656=ORIENTED_EDGE('',*,*,#22460,.F.);
#29657=ORIENTED_EDGE('',*,*,#22461,.F.);
#29658=ORIENTED_EDGE('',*,*,#22462,.F.);
#29659=ORIENTED_EDGE('',*,*,#22463,.F.);
#29660=ORIENTED_EDGE('',*,*,#22464,.F.);
#29661=ORIENTED_EDGE('',*,*,#22465,.F.);
#29662=ORIENTED_EDGE('',*,*,#22466,.F.);
#29663=ORIENTED_EDGE('',*,*,#21321,.F.);
#29664=ORIENTED_EDGE('',*,*,#22459,.T.);
#29665=ORIENTED_EDGE('',*,*,#22467,.T.);
#29666=ORIENTED_EDGE('',*,*,#22468,.T.);
#29667=ORIENTED_EDGE('',*,*,#22469,.T.);
#29668=ORIENTED_EDGE('',*,*,#22470,.T.);
#29669=ORIENTED_EDGE('',*,*,#22471,.T.);
#29670=ORIENTED_EDGE('',*,*,#22454,.T.);
#29671=ORIENTED_EDGE('',*,*,#21323,.F.);
#29672=ORIENTED_EDGE('',*,*,#22472,.F.);
#29673=ORIENTED_EDGE('',*,*,#22473,.T.);
#29674=ORIENTED_EDGE('',*,*,#22474,.F.);
#29675=ORIENTED_EDGE('',*,*,#22475,.T.);
#29676=ORIENTED_EDGE('',*,*,#22476,.F.);
#29677=ORIENTED_EDGE('',*,*,#22477,.T.);
#29678=ORIENTED_EDGE('',*,*,#22478,.F.);
#29679=ORIENTED_EDGE('',*,*,#21325,.F.);
#29680=ORIENTED_EDGE('',*,*,#22456,.T.);
#29681=ORIENTED_EDGE('',*,*,#22479,.F.);
#29682=ORIENTED_EDGE('',*,*,#22480,.T.);
#29683=ORIENTED_EDGE('',*,*,#22481,.F.);
#29684=ORIENTED_EDGE('',*,*,#22482,.T.);
#29685=ORIENTED_EDGE('',*,*,#22483,.F.);
#29686=ORIENTED_EDGE('',*,*,#22457,.T.);
#29687=ORIENTED_EDGE('',*,*,#22480,.F.);
#29688=ORIENTED_EDGE('',*,*,#22484,.F.);
#29689=ORIENTED_EDGE('',*,*,#22470,.F.);
#29690=ORIENTED_EDGE('',*,*,#22485,.F.);
#29691=ORIENTED_EDGE('',*,*,#22482,.F.);
#29692=ORIENTED_EDGE('',*,*,#22486,.F.);
#29693=ORIENTED_EDGE('',*,*,#22468,.F.);
#29694=ORIENTED_EDGE('',*,*,#22487,.F.);
#29695=ORIENTED_EDGE('',*,*,#22471,.F.);
#29696=ORIENTED_EDGE('',*,*,#22484,.T.);
#29697=ORIENTED_EDGE('',*,*,#22479,.T.);
#29698=ORIENTED_EDGE('',*,*,#22455,.T.);
#29699=ORIENTED_EDGE('',*,*,#22483,.T.);
#29700=ORIENTED_EDGE('',*,*,#22487,.T.);
#29701=ORIENTED_EDGE('',*,*,#22467,.F.);
#29702=ORIENTED_EDGE('',*,*,#22458,.T.);
#29703=ORIENTED_EDGE('',*,*,#22469,.F.);
#29704=ORIENTED_EDGE('',*,*,#22486,.T.);
#29705=ORIENTED_EDGE('',*,*,#22481,.T.);
#29706=ORIENTED_EDGE('',*,*,#22485,.T.);
#29707=ORIENTED_EDGE('',*,*,#20868,.T.);
#29708=ORIENTED_EDGE('',*,*,#22476,.T.);
#29709=ORIENTED_EDGE('',*,*,#22488,.T.);
#29710=ORIENTED_EDGE('',*,*,#22462,.T.);
#29711=ORIENTED_EDGE('',*,*,#22489,.T.);
#29712=ORIENTED_EDGE('',*,*,#22474,.T.);
#29713=ORIENTED_EDGE('',*,*,#22490,.T.);
#29714=ORIENTED_EDGE('',*,*,#22464,.T.);
#29715=ORIENTED_EDGE('',*,*,#22491,.T.);
#29716=ORIENTED_EDGE('',*,*,#22472,.T.);
#29717=ORIENTED_EDGE('',*,*,#21322,.T.);
#29718=ORIENTED_EDGE('',*,*,#22466,.T.);
#29719=ORIENTED_EDGE('',*,*,#22492,.T.);
#29720=ORIENTED_EDGE('',*,*,#22478,.T.);
#29721=ORIENTED_EDGE('',*,*,#22493,.T.);
#29722=ORIENTED_EDGE('',*,*,#22460,.T.);
#29723=ORIENTED_EDGE('',*,*,#21318,.T.);
#29724=ORIENTED_EDGE('',*,*,#22461,.T.);
#29725=ORIENTED_EDGE('',*,*,#22493,.F.);
#29726=ORIENTED_EDGE('',*,*,#22477,.F.);
#29727=ORIENTED_EDGE('',*,*,#22489,.F.);
#29728=ORIENTED_EDGE('',*,*,#22473,.F.);
#29729=ORIENTED_EDGE('',*,*,#22492,.F.);
#29730=ORIENTED_EDGE('',*,*,#22465,.T.);
#29731=ORIENTED_EDGE('',*,*,#22490,.F.);
#29732=ORIENTED_EDGE('',*,*,#22463,.T.);
#29733=ORIENTED_EDGE('',*,*,#22488,.F.);
#29734=ORIENTED_EDGE('',*,*,#22475,.F.);
#29735=ORIENTED_EDGE('',*,*,#22491,.F.);
#29736=ORIENTED_EDGE('',*,*,#20870,.F.);
#29737=ORIENTED_EDGE('',*,*,#21257,.F.);
#29738=ORIENTED_EDGE('',*,*,#21300,.F.);
#29739=ORIENTED_EDGE('',*,*,#21196,.T.);
#29740=ORIENTED_EDGE('',*,*,#22494,.T.);
#29741=ORIENTED_EDGE('',*,*,#21258,.F.);
#29742=ORIENTED_EDGE('',*,*,#22494,.F.);
#29743=ORIENTED_EDGE('',*,*,#21223,.T.);
#29744=ORIENTED_EDGE('',*,*,#22495,.T.);
#29745=ORIENTED_EDGE('',*,*,#21259,.F.);
#29746=ORIENTED_EDGE('',*,*,#22495,.F.);
#29747=ORIENTED_EDGE('',*,*,#21222,.T.);
#29748=ORIENTED_EDGE('',*,*,#22496,.T.);
#29749=ORIENTED_EDGE('',*,*,#21261,.F.);
#29750=ORIENTED_EDGE('',*,*,#22497,.F.);
#29751=ORIENTED_EDGE('',*,*,#21220,.T.);
#29752=ORIENTED_EDGE('',*,*,#22498,.T.);
#29753=ORIENTED_EDGE('',*,*,#21262,.F.);
#29754=ORIENTED_EDGE('',*,*,#22498,.F.);
#29755=ORIENTED_EDGE('',*,*,#21219,.T.);
#29756=ORIENTED_EDGE('',*,*,#22499,.T.);
#29757=ORIENTED_EDGE('',*,*,#21263,.F.);
#29758=ORIENTED_EDGE('',*,*,#22499,.F.);
#29759=ORIENTED_EDGE('',*,*,#21218,.T.);
#29760=ORIENTED_EDGE('',*,*,#21302,.T.);
#29761=ORIENTED_EDGE('',*,*,#22500,.F.);
#29762=ORIENTED_EDGE('',*,*,#22501,.F.);
#29763=ORIENTED_EDGE('',*,*,#22497,.T.);
#29764=ORIENTED_EDGE('',*,*,#22502,.T.);
#29765=ORIENTED_EDGE('',*,*,#22503,.F.);
#29766=ORIENTED_EDGE('',*,*,#22504,.T.);
#29767=ORIENTED_EDGE('',*,*,#22505,.T.);
#29768=ORIENTED_EDGE('',*,*,#22496,.F.);
#29769=ORIENTED_EDGE('',*,*,#21260,.F.);
#29770=ORIENTED_EDGE('',*,*,#22505,.F.);
#29771=ORIENTED_EDGE('',*,*,#22506,.T.);
#29772=ORIENTED_EDGE('',*,*,#22502,.F.);
#29773=ORIENTED_EDGE('',*,*,#21221,.T.);
#29774=ORIENTED_EDGE('',*,*,#22501,.T.);
#29775=ORIENTED_EDGE('',*,*,#22507,.T.);
#29776=ORIENTED_EDGE('',*,*,#22503,.T.);
#29777=ORIENTED_EDGE('',*,*,#22508,.F.);
#29778=ORIENTED_EDGE('',*,*,#22500,.T.);
#29779=ORIENTED_EDGE('',*,*,#22509,.T.);
#29780=ORIENTED_EDGE('',*,*,#22510,.T.);
#29781=ORIENTED_EDGE('',*,*,#22511,.T.);
#29782=ORIENTED_EDGE('',*,*,#22504,.F.);
#29783=ORIENTED_EDGE('',*,*,#22512,.F.);
#29784=ORIENTED_EDGE('',*,*,#22513,.F.);
#29785=ORIENTED_EDGE('',*,*,#22506,.F.);
#29786=ORIENTED_EDGE('',*,*,#22511,.F.);
#29787=ORIENTED_EDGE('',*,*,#22514,.F.);
#29788=ORIENTED_EDGE('',*,*,#22515,.F.);
#29789=ORIENTED_EDGE('',*,*,#22516,.F.);
#29790=ORIENTED_EDGE('',*,*,#22509,.F.);
#29791=ORIENTED_EDGE('',*,*,#22512,.T.);
#29792=ORIENTED_EDGE('',*,*,#22507,.F.);
#29793=ORIENTED_EDGE('',*,*,#22508,.T.);
#29794=ORIENTED_EDGE('',*,*,#22517,.T.);
#29795=ORIENTED_EDGE('',*,*,#22518,.T.);
#29796=ORIENTED_EDGE('',*,*,#22519,.T.);
#29797=ORIENTED_EDGE('',*,*,#22519,.F.);
#29798=ORIENTED_EDGE('',*,*,#22520,.F.);
#29799=ORIENTED_EDGE('',*,*,#22514,.T.);
#29800=ORIENTED_EDGE('',*,*,#22513,.T.);
#29801=ORIENTED_EDGE('',*,*,#22518,.F.);
#29802=ORIENTED_EDGE('',*,*,#22521,.F.);
#29803=ORIENTED_EDGE('',*,*,#22515,.T.);
#29804=ORIENTED_EDGE('',*,*,#22520,.T.);
#29805=ORIENTED_EDGE('',*,*,#22517,.F.);
#29806=ORIENTED_EDGE('',*,*,#22510,.F.);
#29807=ORIENTED_EDGE('',*,*,#22516,.T.);
#29808=ORIENTED_EDGE('',*,*,#22521,.T.);
#37719=CYLINDRICAL_SURFACE('',#39985,1.75);
#37720=CYLINDRICAL_SURFACE('',#39988,1.75);
#37721=CYLINDRICAL_SURFACE('',#39991,1.75);
#37722=CYLINDRICAL_SURFACE('',#39994,1.75);
#37723=CYLINDRICAL_SURFACE('',#39997,1.25);
#37724=CYLINDRICAL_SURFACE('',#40000,1.25);
#37725=CYLINDRICAL_SURFACE('',#40003,1.5);
#37726=CYLINDRICAL_SURFACE('',#40006,1.5);
#37727=CYLINDRICAL_SURFACE('',#40009,1.5);
#37728=CYLINDRICAL_SURFACE('',#40012,1.5);
#37729=CYLINDRICAL_SURFACE('',#40015,1.5);
#37730=CYLINDRICAL_SURFACE('',#40018,1.5);
#37731=CYLINDRICAL_SURFACE('',#40021,1.5);
#37732=CYLINDRICAL_SURFACE('',#40024,1.5);
#37733=CYLINDRICAL_SURFACE('',#40027,1.5);
#37734=CYLINDRICAL_SURFACE('',#40030,1.5);
#37735=CYLINDRICAL_SURFACE('',#40033,1.5);
#37736=CYLINDRICAL_SURFACE('',#40036,1.5);
#37737=CYLINDRICAL_SURFACE('',#40039,1.5);
#37738=CYLINDRICAL_SURFACE('',#40042,1.5);
#37739=CYLINDRICAL_SURFACE('',#40045,1.5);
#37740=CYLINDRICAL_SURFACE('',#40048,1.5);
#37741=CYLINDRICAL_SURFACE('',#40051,1.5);
#37742=CYLINDRICAL_SURFACE('',#40054,1.5);
#37743=CYLINDRICAL_SURFACE('',#40057,1.5);
#37744=CYLINDRICAL_SURFACE('',#40060,1.5);
#37745=CYLINDRICAL_SURFACE('',#40063,1.5);
#37746=CYLINDRICAL_SURFACE('',#40066,1.5);
#37747=CYLINDRICAL_SURFACE('',#40069,1.5);
#37748=CYLINDRICAL_SURFACE('',#40072,1.5);
#37749=CYLINDRICAL_SURFACE('',#40075,1.5);
#37750=CYLINDRICAL_SURFACE('',#40078,1.5);
#37751=CYLINDRICAL_SURFACE('',#40081,1.5);
#37752=CYLINDRICAL_SURFACE('',#40084,1.5);
#37753=CYLINDRICAL_SURFACE('',#40087,1.5);
#37754=CYLINDRICAL_SURFACE('',#40090,1.5);
#37755=CYLINDRICAL_SURFACE('',#40093,1.5);
#37756=CYLINDRICAL_SURFACE('',#40096,1.5);
#37757=CYLINDRICAL_SURFACE('',#40099,1.5);
#37758=CYLINDRICAL_SURFACE('',#40102,1.5);
#37759=CYLINDRICAL_SURFACE('',#40105,1.5);
#37760=CYLINDRICAL_SURFACE('',#40108,1.5);
#37761=CYLINDRICAL_SURFACE('',#40111,1.5);
#37762=CYLINDRICAL_SURFACE('',#40114,1.5);
#37763=CYLINDRICAL_SURFACE('',#40117,1.5);
#37764=CYLINDRICAL_SURFACE('',#40120,1.5);
#37765=CYLINDRICAL_SURFACE('',#40123,1.5);
#37766=CYLINDRICAL_SURFACE('',#40126,1.5);
#37767=CYLINDRICAL_SURFACE('',#40129,1.5);
#37768=CYLINDRICAL_SURFACE('',#40132,1.5);
#37769=CYLINDRICAL_SURFACE('',#40135,1.5);
#37770=CYLINDRICAL_SURFACE('',#40138,1.5);
#37771=CYLINDRICAL_SURFACE('',#40141,1.5);
#37772=CYLINDRICAL_SURFACE('',#40144,1.5);
#37773=CYLINDRICAL_SURFACE('',#40147,1.5);
#37774=CYLINDRICAL_SURFACE('',#40150,1.5);
#37775=CYLINDRICAL_SURFACE('',#40153,1.5);
#37776=CYLINDRICAL_SURFACE('',#40156,1.5);
#37777=CYLINDRICAL_SURFACE('',#40159,1.5);
#37778=CYLINDRICAL_SURFACE('',#40162,1.5);
#37779=CYLINDRICAL_SURFACE('',#40165,1.5);
#37780=CYLINDRICAL_SURFACE('',#40168,1.5);
#37781=CYLINDRICAL_SURFACE('',#40171,1.5);
#37782=CYLINDRICAL_SURFACE('',#40174,1.5);
#37783=CYLINDRICAL_SURFACE('',#40177,1.5);
#37784=CYLINDRICAL_SURFACE('',#40180,1.5);
#37785=CYLINDRICAL_SURFACE('',#40183,1.5);
#37786=CYLINDRICAL_SURFACE('',#40186,1.5);
#37787=CYLINDRICAL_SURFACE('',#40189,1.5);
#37788=CYLINDRICAL_SURFACE('',#40192,1.5);
#37789=CYLINDRICAL_SURFACE('',#40195,1.5);
#37790=CYLINDRICAL_SURFACE('',#40198,1.5);
#37791=CYLINDRICAL_SURFACE('',#40201,1.74999999999999);
#37792=CYLINDRICAL_SURFACE('',#40204,1.74999999999998);
#37793=CYLINDRICAL_SURFACE('',#40207,1.75);
#37794=CYLINDRICAL_SURFACE('',#40210,1.75);
#37795=CYLINDRICAL_SURFACE('',#40227,1.25);
#37796=CYLINDRICAL_SURFACE('',#40230,1.25);
#37797=CYLINDRICAL_SURFACE('',#40233,1.25);
#37798=CYLINDRICAL_SURFACE('',#40236,1.25);
#37799=CYLINDRICAL_SURFACE('',#40459,1.5);
#37800=CYLINDRICAL_SURFACE('',#40461,1.5);
#37801=CYLINDRICAL_SURFACE('',#40463,1.5);
#37802=CYLINDRICAL_SURFACE('',#40465,1.5);
#37803=CYLINDRICAL_SURFACE('',#40467,1.6);
#37804=CYLINDRICAL_SURFACE('',#40468,0.799999999999995);
#37805=CYLINDRICAL_SURFACE('',#40474,1.5);
#37806=CYLINDRICAL_SURFACE('',#40475,1.5);
#37807=CYLINDRICAL_SURFACE('',#40476,1.6);
#37808=CYLINDRICAL_SURFACE('',#40477,0.799999999999995);
#37809=CYLINDRICAL_SURFACE('',#40483,1.5);
#37810=CYLINDRICAL_SURFACE('',#40484,1.5);
#37811=CYLINDRICAL_SURFACE('',#40491,2.);
#37812=CYLINDRICAL_SURFACE('',#40494,2.);
#37813=CYLINDRICAL_SURFACE('',#40511,1.5);
#37814=CYLINDRICAL_SURFACE('',#40512,1.5);
#37815=CYLINDRICAL_SURFACE('',#40516,2.3);
#37816=CYLINDRICAL_SURFACE('',#40517,2.3);
#37817=CYLINDRICAL_SURFACE('',#40518,1.20000000000001);
#37818=CYLINDRICAL_SURFACE('',#40519,1.2);
#37819=CYLINDRICAL_SURFACE('',#40529,2.);
#37820=CYLINDRICAL_SURFACE('',#40532,2.);
#37821=CYLINDRICAL_SURFACE('',#40549,1.5);
#37822=CYLINDRICAL_SURFACE('',#40550,1.5);
#37823=CYLINDRICAL_SURFACE('',#40554,2.3);
#37824=CYLINDRICAL_SURFACE('',#40555,2.3);
#37825=CYLINDRICAL_SURFACE('',#40556,1.20000000000001);
#37826=CYLINDRICAL_SURFACE('',#40557,1.2);
#37827=CYLINDRICAL_SURFACE('',#40567,2.);
#37828=CYLINDRICAL_SURFACE('',#40570,2.);
#37829=CYLINDRICAL_SURFACE('',#40587,1.5);
#37830=CYLINDRICAL_SURFACE('',#40588,1.5);
#37831=CYLINDRICAL_SURFACE('',#40592,2.3);
#37832=CYLINDRICAL_SURFACE('',#40593,2.3);
#37833=CYLINDRICAL_SURFACE('',#40594,1.2);
#37834=CYLINDRICAL_SURFACE('',#40595,1.2);
#37835=CYLINDRICAL_SURFACE('',#40605,2.);
#37836=CYLINDRICAL_SURFACE('',#40608,2.);
#37837=CYLINDRICAL_SURFACE('',#40625,1.5);
#37838=CYLINDRICAL_SURFACE('',#40626,1.5);
#37839=CYLINDRICAL_SURFACE('',#40630,2.3);
#37840=CYLINDRICAL_SURFACE('',#40631,2.3);
#37841=CYLINDRICAL_SURFACE('',#40632,1.2);
#37842=CYLINDRICAL_SURFACE('',#40633,1.2);
#37843=CYLINDRICAL_SURFACE('',#40703,1.5);
#37844=CYLINDRICAL_SURFACE('',#40704,1.5);
#37845=CYLINDRICAL_SURFACE('',#40705,1.5);
#37846=CYLINDRICAL_SURFACE('',#40706,1.5);
#37847=CYLINDRICAL_SURFACE('',#40707,1.5);
#37848=CYLINDRICAL_SURFACE('',#40708,1.5);
#37849=CYLINDRICAL_SURFACE('',#40709,1.5);
#37850=CYLINDRICAL_SURFACE('',#40710,1.5);
#37851=CYLINDRICAL_SURFACE('',#40711,1.5);
#37852=CYLINDRICAL_SURFACE('',#40712,1.5);
#37853=CYLINDRICAL_SURFACE('',#40713,1.5);
#37854=CYLINDRICAL_SURFACE('',#40714,1.5);
#37855=CYLINDRICAL_SURFACE('',#40715,1.5);
#37856=CYLINDRICAL_SURFACE('',#40716,1.5);
#37857=CYLINDRICAL_SURFACE('',#40717,1.5);
#37858=CYLINDRICAL_SURFACE('',#40718,1.5);
#37859=CYLINDRICAL_SURFACE('',#40719,1.5);
#37860=CYLINDRICAL_SURFACE('',#40720,1.5);
#37861=CYLINDRICAL_SURFACE('',#40721,1.5);
#37862=CYLINDRICAL_SURFACE('',#40722,1.5);
#37863=CYLINDRICAL_SURFACE('',#40723,1.5);
#37864=CYLINDRICAL_SURFACE('',#40724,1.5);
#37865=CYLINDRICAL_SURFACE('',#40725,1.5);
#37866=CYLINDRICAL_SURFACE('',#40726,1.5);
#37867=CYLINDRICAL_SURFACE('',#40727,1.5);
#37868=CYLINDRICAL_SURFACE('',#40728,1.5);
#37869=CYLINDRICAL_SURFACE('',#40729,1.5);
#37870=CYLINDRICAL_SURFACE('',#40730,1.5);
#37871=CYLINDRICAL_SURFACE('',#40731,1.5);
#37872=CYLINDRICAL_SURFACE('',#40732,1.5);
#37873=CYLINDRICAL_SURFACE('',#40733,1.5);
#37874=CYLINDRICAL_SURFACE('',#40734,1.5);
#37875=CYLINDRICAL_SURFACE('',#40735,1.5);
#37876=CYLINDRICAL_SURFACE('',#40736,1.5);
#37877=CYLINDRICAL_SURFACE('',#40737,1.5);
#37878=CYLINDRICAL_SURFACE('',#40738,1.5);
#37879=CYLINDRICAL_SURFACE('',#40739,1.5);
#37880=CYLINDRICAL_SURFACE('',#40740,1.5);
#37881=CYLINDRICAL_SURFACE('',#40741,1.5);
#37882=CYLINDRICAL_SURFACE('',#40742,1.5);
#37883=CYLINDRICAL_SURFACE('',#40743,1.5);
#37884=CYLINDRICAL_SURFACE('',#40744,1.5);
#37885=CYLINDRICAL_SURFACE('',#40745,1.5);
#37886=CYLINDRICAL_SURFACE('',#40746,1.5);
#37887=CYLINDRICAL_SURFACE('',#40747,1.5);
#37888=CYLINDRICAL_SURFACE('',#40748,1.5);
#37889=CYLINDRICAL_SURFACE('',#40749,1.5);
#37890=CYLINDRICAL_SURFACE('',#40750,1.5);
#37891=CYLINDRICAL_SURFACE('',#40751,1.5);
#37892=CYLINDRICAL_SURFACE('',#40752,1.5);
#37893=CYLINDRICAL_SURFACE('',#40753,1.5);
#37894=CYLINDRICAL_SURFACE('',#40754,1.5);
#37895=CYLINDRICAL_SURFACE('',#40755,1.5);
#37896=CYLINDRICAL_SURFACE('',#40756,1.5);
#37897=CYLINDRICAL_SURFACE('',#40757,2.667);
#37898=CYLINDRICAL_SURFACE('',#40759,2.667);
#37899=CYLINDRICAL_SURFACE('',#40761,2.66699999999999);
#37900=CYLINDRICAL_SURFACE('',#40763,2.667);
#37901=CYLINDRICAL_SURFACE('',#40765,2.667);
#37902=CYLINDRICAL_SURFACE('',#40767,2.667);
#37903=CYLINDRICAL_SURFACE('',#40778,1.5);
#37904=CYLINDRICAL_SURFACE('',#40782,1.5);
#37905=CYLINDRICAL_SURFACE('',#40785,1.5);
#37906=CYLINDRICAL_SURFACE('',#40787,1.5);
#37907=CYLINDRICAL_SURFACE('',#40791,1.5);
#37908=CYLINDRICAL_SURFACE('',#40793,1.5);
#37909=CYLINDRICAL_SURFACE('',#40796,1.5);
#37910=CYLINDRICAL_SURFACE('',#40800,1.5);
#37911=CYLINDRICAL_SURFACE('',#40803,1.5);
#37912=CYLINDRICAL_SURFACE('',#40806,1.5);
#37913=CYLINDRICAL_SURFACE('',#40809,1.5);
#37914=CYLINDRICAL_SURFACE('',#40811,1.5);
#37915=CYLINDRICAL_SURFACE('',#40814,1.5);
#37916=CYLINDRICAL_SURFACE('',#40817,1.5);
#37917=CYLINDRICAL_SURFACE('',#40820,1.5);
#37918=CYLINDRICAL_SURFACE('',#40823,1.5);
#37919=CYLINDRICAL_SURFACE('',#40826,1.5);
#37920=CYLINDRICAL_SURFACE('',#40829,1.5);
#37921=CYLINDRICAL_SURFACE('',#40833,1.5);
#37922=CYLINDRICAL_SURFACE('',#40836,1.5);
#37923=CYLINDRICAL_SURFACE('',#40839,1.5);
#37924=CYLINDRICAL_SURFACE('',#40842,1.5);
#37925=CYLINDRICAL_SURFACE('',#40845,1.5);
#37926=CYLINDRICAL_SURFACE('',#40847,1.5);
#37927=CYLINDRICAL_SURFACE('',#40850,1.5);
#37928=CYLINDRICAL_SURFACE('',#40853,1.5);
#37929=CYLINDRICAL_SURFACE('',#40856,1.5);
#37930=CYLINDRICAL_SURFACE('',#40859,1.5);
#37931=CYLINDRICAL_SURFACE('',#40862,1.5);
#37932=CYLINDRICAL_SURFACE('',#40865,1.5);
#37933=CYLINDRICAL_SURFACE('',#40868,1.5);
#37934=CYLINDRICAL_SURFACE('',#40871,1.5);
#37935=CYLINDRICAL_SURFACE('',#40874,1.5);
#37936=CYLINDRICAL_SURFACE('',#40877,1.5);
#37937=CYLINDRICAL_SURFACE('',#40880,1.5);
#37938=CYLINDRICAL_SURFACE('',#40883,1.5);
#37939=CYLINDRICAL_SURFACE('',#40886,1.5);
#37940=CYLINDRICAL_SURFACE('',#40889,1.5);
#37941=CYLINDRICAL_SURFACE('',#40892,1.5);
#37942=CYLINDRICAL_SURFACE('',#40895,1.5);
#37943=CYLINDRICAL_SURFACE('',#40898,1.5);
#37944=CYLINDRICAL_SURFACE('',#40901,1.5);
#37945=CYLINDRICAL_SURFACE('',#40904,1.5);
#37946=CYLINDRICAL_SURFACE('',#40907,1.5);
#37947=CYLINDRICAL_SURFACE('',#40910,1.5);
#37948=CYLINDRICAL_SURFACE('',#40913,1.5);
#37949=CYLINDRICAL_SURFACE('',#40916,1.5);
#37950=CYLINDRICAL_SURFACE('',#40919,1.5);
#37951=CYLINDRICAL_SURFACE('',#40933,1.59999999999999);
#37952=CYLINDRICAL_SURFACE('',#40934,0.799999999999995);
#37953=CYLINDRICAL_SURFACE('',#40937,4.);
#37954=CYLINDRICAL_SURFACE('',#40939,4.);
#37955=CYLINDRICAL_SURFACE('',#40946,2.);
#37956=CYLINDRICAL_SURFACE('',#40949,2.);
#37957=CYLINDRICAL_SURFACE('',#40966,1.5);
#37958=CYLINDRICAL_SURFACE('',#40967,1.5);
#37959=CYLINDRICAL_SURFACE('',#40971,2.3);
#37960=CYLINDRICAL_SURFACE('',#40972,2.3);
#37961=CYLINDRICAL_SURFACE('',#40973,1.2);
#37962=CYLINDRICAL_SURFACE('',#40974,1.2);
#37963=CYLINDRICAL_SURFACE('',#40984,2.);
#37964=CYLINDRICAL_SURFACE('',#40987,2.);
#37965=CYLINDRICAL_SURFACE('',#41004,1.5);
#37966=CYLINDRICAL_SURFACE('',#41005,1.5);
#37967=CYLINDRICAL_SURFACE('',#41009,2.3);
#37968=CYLINDRICAL_SURFACE('',#41010,2.3);
#37969=CYLINDRICAL_SURFACE('',#41011,1.2);
#37970=CYLINDRICAL_SURFACE('',#41012,1.2);
#37971=CYLINDRICAL_SURFACE('',#41028,1.59999999999999);
#37972=CYLINDRICAL_SURFACE('',#41029,0.799999999999995);
#37973=CYLINDRICAL_SURFACE('',#41038,4.);
#37974=CYLINDRICAL_SURFACE('',#41040,4.);
#38019=ADVANCED_FACE('',(#2331),#37719,.F.);
#38020=ADVANCED_FACE('',(#2332),#37720,.F.);
#38021=ADVANCED_FACE('',(#2333),#37721,.F.);
#38022=ADVANCED_FACE('',(#2334),#37722,.F.);
#38023=ADVANCED_FACE('',(#2335),#37723,.F.);
#38024=ADVANCED_FACE('',(#2336),#37724,.F.);
#38025=ADVANCED_FACE('',(#2337),#37725,.F.);
#38026=ADVANCED_FACE('',(#2338),#37726,.F.);
#38027=ADVANCED_FACE('',(#2339),#37727,.F.);
#38028=ADVANCED_FACE('',(#2340),#37728,.F.);
#38029=ADVANCED_FACE('',(#2341),#37729,.F.);
#38030=ADVANCED_FACE('',(#2342),#37730,.F.);
#38031=ADVANCED_FACE('',(#2343),#37731,.F.);
#38032=ADVANCED_FACE('',(#2344),#37732,.F.);
#38033=ADVANCED_FACE('',(#2345),#37733,.F.);
#38034=ADVANCED_FACE('',(#2346),#37734,.F.);
#38035=ADVANCED_FACE('',(#2347),#37735,.F.);
#38036=ADVANCED_FACE('',(#2348),#37736,.F.);
#38037=ADVANCED_FACE('',(#2349),#37737,.F.);
#38038=ADVANCED_FACE('',(#2350),#37738,.F.);
#38039=ADVANCED_FACE('',(#2351),#37739,.F.);
#38040=ADVANCED_FACE('',(#2352),#37740,.F.);
#38041=ADVANCED_FACE('',(#2353),#37741,.F.);
#38042=ADVANCED_FACE('',(#2354),#37742,.F.);
#38043=ADVANCED_FACE('',(#2355),#37743,.F.);
#38044=ADVANCED_FACE('',(#2356),#37744,.F.);
#38045=ADVANCED_FACE('',(#2357),#37745,.F.);
#38046=ADVANCED_FACE('',(#2358),#37746,.F.);
#38047=ADVANCED_FACE('',(#2359),#37747,.F.);
#38048=ADVANCED_FACE('',(#2360),#37748,.F.);
#38049=ADVANCED_FACE('',(#2361),#37749,.F.);
#38050=ADVANCED_FACE('',(#2362),#37750,.F.);
#38051=ADVANCED_FACE('',(#2363),#37751,.F.);
#38052=ADVANCED_FACE('',(#2364),#37752,.F.);
#38053=ADVANCED_FACE('',(#2365),#37753,.F.);
#38054=ADVANCED_FACE('',(#2366),#37754,.F.);
#38055=ADVANCED_FACE('',(#2367),#37755,.F.);
#38056=ADVANCED_FACE('',(#2368),#37756,.F.);
#38057=ADVANCED_FACE('',(#2369),#37757,.F.);
#38058=ADVANCED_FACE('',(#2370),#37758,.F.);
#38059=ADVANCED_FACE('',(#2371),#37759,.F.);
#38060=ADVANCED_FACE('',(#2372),#37760,.F.);
#38061=ADVANCED_FACE('',(#2373),#37761,.F.);
#38062=ADVANCED_FACE('',(#2374),#37762,.F.);
#38063=ADVANCED_FACE('',(#2375),#37763,.F.);
#38064=ADVANCED_FACE('',(#2376),#37764,.F.);
#38065=ADVANCED_FACE('',(#2377),#37765,.F.);
#38066=ADVANCED_FACE('',(#2378),#37766,.F.);
#38067=ADVANCED_FACE('',(#2379),#37767,.F.);
#38068=ADVANCED_FACE('',(#2380),#37768,.F.);
#38069=ADVANCED_FACE('',(#2381),#37769,.F.);
#38070=ADVANCED_FACE('',(#2382),#37770,.F.);
#38071=ADVANCED_FACE('',(#2383),#37771,.F.);
#38072=ADVANCED_FACE('',(#2384),#37772,.F.);
#38073=ADVANCED_FACE('',(#2385),#37773,.F.);
#38074=ADVANCED_FACE('',(#2386),#37774,.F.);
#38075=ADVANCED_FACE('',(#2387),#37775,.F.);
#38076=ADVANCED_FACE('',(#2388),#37776,.F.);
#38077=ADVANCED_FACE('',(#2389),#37777,.F.);
#38078=ADVANCED_FACE('',(#2390),#37778,.F.);
#38079=ADVANCED_FACE('',(#2391),#37779,.F.);
#38080=ADVANCED_FACE('',(#2392),#37780,.F.);
#38081=ADVANCED_FACE('',(#2393),#37781,.F.);
#38082=ADVANCED_FACE('',(#2394),#37782,.F.);
#38083=ADVANCED_FACE('',(#2395),#37783,.F.);
#38084=ADVANCED_FACE('',(#2396),#37784,.F.);
#38085=ADVANCED_FACE('',(#2397),#37785,.F.);
#38086=ADVANCED_FACE('',(#2398),#37786,.F.);
#38087=ADVANCED_FACE('',(#2399),#37787,.F.);
#38088=ADVANCED_FACE('',(#2400),#37788,.F.);
#38089=ADVANCED_FACE('',(#2401),#37789,.F.);
#38090=ADVANCED_FACE('',(#2402),#37790,.F.);
#38091=ADVANCED_FACE('',(#2403),#2285,.T.);
#38092=ADVANCED_FACE('',(#2404),#2286,.T.);
#38093=ADVANCED_FACE('',(#2405),#2287,.T.);
#38094=ADVANCED_FACE('',(#2406),#2288,.T.);
#38095=ADVANCED_FACE('',(#2407),#2289,.T.);
#38096=ADVANCED_FACE('',(#2408),#37791,.F.);
#38097=ADVANCED_FACE('',(#2409),#37792,.F.);
#38098=ADVANCED_FACE('',(#2410),#37793,.F.);
#38099=ADVANCED_FACE('',(#2411),#37794,.F.);
#38100=ADVANCED_FACE('',(#2412),#2181,.F.);
#38101=ADVANCED_FACE('',(#2413),#2182,.F.);
#38102=ADVANCED_FACE('',(#2414),#2183,.T.);
#38103=ADVANCED_FACE('',(#2415),#2184,.T.);
#38104=ADVANCED_FACE('',(#2416),#37795,.F.);
#38105=ADVANCED_FACE('',(#2417),#37796,.F.);
#38106=ADVANCED_FACE('',(#2418),#37797,.F.);
#38107=ADVANCED_FACE('',(#2419),#37798,.F.);
#38108=ADVANCED_FACE('',(#2420),#2290,.F.);
#38109=ADVANCED_FACE('',(#2421,#48,#49,#50,#51),#629,.F.);
#38110=ADVANCED_FACE('',(#2422,#52,#53,#54,#55),#630,.T.);
#38111=ADVANCED_FACE('',(#2423),#631,.T.);
#38112=ADVANCED_FACE('',(#2424),#632,.T.);
#38113=ADVANCED_FACE('',(#2425,#56,#57),#633,.T.);
#38114=ADVANCED_FACE('',(#2426,#58,#59),#634,.F.);
#38115=ADVANCED_FACE('',(#2427),#635,.T.);
#38116=ADVANCED_FACE('',(#2428),#636,.T.);
#38117=ADVANCED_FACE('',(#2429,#60,#61,#62,#63,#64,#65,#66,#67,#68,#69,
#70,#71,#72,#73,#74,#75,#76,#77,#78,#79,#80,#81,#82,#83,#84,#85,#86,#87,
#88,#89,#90,#91,#92,#93,#94,#95,#96,#97,#98,#99,#100,#101,#102,#103,#104,
#105,#106,#107),#637,.T.);
#38118=ADVANCED_FACE('',(#2430,#108,#109,#110,#111,#112,#113,#114,#115,
#116,#117,#118,#119,#120,#121,#122,#123,#124,#125,#126,#127,#128,#129,#130,
#131,#132,#133,#134,#135,#136,#137,#138,#139,#140,#141,#142,#143,#144,#145,
#146,#147,#148,#149,#150,#151,#152,#153,#154,#155),#638,.F.);
#38119=ADVANCED_FACE('',(#2431),#639,.T.);
#38120=ADVANCED_FACE('',(#2432),#640,.T.);
#38121=ADVANCED_FACE('',(#2433),#641,.T.);
#38122=ADVANCED_FACE('',(#2434),#642,.T.);
#38123=ADVANCED_FACE('',(#2435),#643,.T.);
#38124=ADVANCED_FACE('',(#2436),#644,.T.);
#38125=ADVANCED_FACE('',(#2437),#645,.T.);
#38126=ADVANCED_FACE('',(#2438),#646,.T.);
#38127=ADVANCED_FACE('',(#2439),#647,.T.);
#38128=ADVANCED_FACE('',(#2440),#648,.T.);
#38129=ADVANCED_FACE('',(#2441),#649,.T.);
#38130=ADVANCED_FACE('',(#2442),#650,.T.);
#38131=ADVANCED_FACE('',(#2443),#651,.T.);
#38132=ADVANCED_FACE('',(#2444),#652,.T.);
#38133=ADVANCED_FACE('',(#2445),#653,.T.);
#38134=ADVANCED_FACE('',(#2446),#654,.T.);
#38135=ADVANCED_FACE('',(#2447),#655,.T.);
#38136=ADVANCED_FACE('',(#2448),#656,.T.);
#38137=ADVANCED_FACE('',(#2449),#657,.T.);
#38138=ADVANCED_FACE('',(#2450),#658,.T.);
#38139=ADVANCED_FACE('',(#2451),#659,.T.);
#38140=ADVANCED_FACE('',(#2452),#660,.T.);
#38141=ADVANCED_FACE('',(#2453),#661,.T.);
#38142=ADVANCED_FACE('',(#2454),#662,.T.);
#38143=ADVANCED_FACE('',(#2455),#2291,.F.);
#38144=ADVANCED_FACE('',(#2456,#156,#157,#158,#159,#160,#161,#162,#163,
#164,#165,#166,#167,#168,#169,#170,#171,#172,#173),#663,.F.);
#38145=ADVANCED_FACE('',(#2457),#2292,.F.);
#38146=ADVANCED_FACE('',(#2458),#664,.T.);
#38147=ADVANCED_FACE('',(#2459),#2293,.F.);
#38148=ADVANCED_FACE('',(#2460),#2294,.F.);
#38149=ADVANCED_FACE('',(#2461),#2295,.F.);
#38150=ADVANCED_FACE('',(#2462,#174,#175,#176,#177,#178,#179,#180,#181,
#182,#183,#184),#665,.T.);
#38151=ADVANCED_FACE('',(#2463,#185,#186,#187,#188,#189,#190,#191,#192,
#193,#194,#195),#666,.F.);
#38152=ADVANCED_FACE('',(#2464),#37799,.F.);
#38153=ADVANCED_FACE('',(#2465),#667,.F.);
#38154=ADVANCED_FACE('',(#2466),#37800,.F.);
#38155=ADVANCED_FACE('',(#2467),#668,.F.);
#38156=ADVANCED_FACE('',(#2468),#37801,.F.);
#38157=ADVANCED_FACE('',(#2469),#669,.F.);
#38158=ADVANCED_FACE('',(#2470),#37802,.F.);
#38159=ADVANCED_FACE('',(#2471),#670,.F.);
#38160=ADVANCED_FACE('',(#2472),#2296,.T.);
#38161=ADVANCED_FACE('',(#2473),#2297,.T.);
#38162=ADVANCED_FACE('',(#2474),#37803,.T.);
#38163=ADVANCED_FACE('',(#2475),#37804,.F.);
#38164=ADVANCED_FACE('',(#2476),#671,.F.);
#38165=ADVANCED_FACE('',(#2477),#672,.T.);
#38166=ADVANCED_FACE('',(#2478),#673,.T.);
#38167=ADVANCED_FACE('',(#2479),#674,.T.);
#38168=ADVANCED_FACE('',(#2480),#675,.F.);
#38169=ADVANCED_FACE('',(#2481),#37805,.F.);
#38170=ADVANCED_FACE('',(#2482),#37806,.F.);
#38171=ADVANCED_FACE('',(#2483),#2298,.T.);
#38172=ADVANCED_FACE('',(#2484),#2299,.T.);
#38173=ADVANCED_FACE('',(#2485),#37807,.T.);
#38174=ADVANCED_FACE('',(#2486),#37808,.F.);
#38175=ADVANCED_FACE('',(#2487),#676,.F.);
#38176=ADVANCED_FACE('',(#2488),#677,.F.);
#38177=ADVANCED_FACE('',(#2489),#678,.T.);
#38178=ADVANCED_FACE('',(#2490),#679,.T.);
#38179=ADVANCED_FACE('',(#2491),#680,.F.);
#38180=ADVANCED_FACE('',(#2492),#37809,.F.);
#38181=ADVANCED_FACE('',(#2493),#37810,.F.);
#38182=ADVANCED_FACE('',(#2494),#681,.T.);
#38183=ADVANCED_FACE('',(#2495),#682,.F.);
#38184=ADVANCED_FACE('',(#2496),#37811,.T.);
#38185=ADVANCED_FACE('',(#2497),#37812,.T.);
#38186=ADVANCED_FACE('',(#2498),#683,.F.);
#38187=ADVANCED_FACE('',(#2499),#684,.T.);
#38188=ADVANCED_FACE('',(#2500),#37813,.F.);
#38189=ADVANCED_FACE('',(#2501),#37814,.F.);
#38190=ADVANCED_FACE('',(#2502),#685,.F.);
#38191=ADVANCED_FACE('',(#2503),#686,.F.);
#38192=ADVANCED_FACE('',(#2504,#196),#687,.F.);
#38193=ADVANCED_FACE('',(#2505),#37815,.T.);
#38194=ADVANCED_FACE('',(#2506),#37816,.T.);
#38195=ADVANCED_FACE('',(#2507),#37817,.F.);
#38196=ADVANCED_FACE('',(#2508),#37818,.F.);
#38197=ADVANCED_FACE('',(#2509),#688,.T.);
#38198=ADVANCED_FACE('',(#2510),#689,.T.);
#38199=ADVANCED_FACE('',(#2511,#197),#690,.T.);
#38200=ADVANCED_FACE('',(#2512),#691,.T.);
#38201=ADVANCED_FACE('',(#2513),#692,.F.);
#38202=ADVANCED_FACE('',(#2514),#37819,.T.);
#38203=ADVANCED_FACE('',(#2515),#37820,.T.);
#38204=ADVANCED_FACE('',(#2516),#693,.F.);
#38205=ADVANCED_FACE('',(#2517),#694,.T.);
#38206=ADVANCED_FACE('',(#2518),#37821,.F.);
#38207=ADVANCED_FACE('',(#2519),#37822,.F.);
#38208=ADVANCED_FACE('',(#2520),#695,.F.);
#38209=ADVANCED_FACE('',(#2521),#696,.F.);
#38210=ADVANCED_FACE('',(#2522,#198),#697,.F.);
#38211=ADVANCED_FACE('',(#2523),#37823,.T.);
#38212=ADVANCED_FACE('',(#2524),#37824,.T.);
#38213=ADVANCED_FACE('',(#2525),#37825,.F.);
#38214=ADVANCED_FACE('',(#2526),#37826,.F.);
#38215=ADVANCED_FACE('',(#2527),#698,.T.);
#38216=ADVANCED_FACE('',(#2528),#699,.T.);
#38217=ADVANCED_FACE('',(#2529,#199),#700,.T.);
#38218=ADVANCED_FACE('',(#2530),#701,.T.);
#38219=ADVANCED_FACE('',(#2531),#702,.F.);
#38220=ADVANCED_FACE('',(#2532),#37827,.T.);
#38221=ADVANCED_FACE('',(#2533),#37828,.T.);
#38222=ADVANCED_FACE('',(#2534),#703,.F.);
#38223=ADVANCED_FACE('',(#2535),#704,.T.);
#38224=ADVANCED_FACE('',(#2536),#37829,.F.);
#38225=ADVANCED_FACE('',(#2537),#37830,.F.);
#38226=ADVANCED_FACE('',(#2538),#705,.F.);
#38227=ADVANCED_FACE('',(#2539),#706,.F.);
#38228=ADVANCED_FACE('',(#2540,#200),#707,.F.);
#38229=ADVANCED_FACE('',(#2541),#37831,.T.);
#38230=ADVANCED_FACE('',(#2542),#37832,.T.);
#38231=ADVANCED_FACE('',(#2543),#37833,.F.);
#38232=ADVANCED_FACE('',(#2544),#37834,.F.);
#38233=ADVANCED_FACE('',(#2545),#708,.T.);
#38234=ADVANCED_FACE('',(#2546),#709,.T.);
#38235=ADVANCED_FACE('',(#2547,#201),#710,.T.);
#38236=ADVANCED_FACE('',(#2548),#711,.T.);
#38237=ADVANCED_FACE('',(#2549),#712,.F.);
#38238=ADVANCED_FACE('',(#2550),#37835,.T.);
#38239=ADVANCED_FACE('',(#2551),#37836,.T.);
#38240=ADVANCED_FACE('',(#2552),#713,.F.);
#38241=ADVANCED_FACE('',(#2553),#714,.T.);
#38242=ADVANCED_FACE('',(#2554),#37837,.F.);
#38243=ADVANCED_FACE('',(#2555),#37838,.F.);
#38244=ADVANCED_FACE('',(#2556),#715,.F.);
#38245=ADVANCED_FACE('',(#2557),#716,.F.);
#38246=ADVANCED_FACE('',(#2558,#202),#717,.F.);
#38247=ADVANCED_FACE('',(#2559),#37839,.T.);
#38248=ADVANCED_FACE('',(#2560),#37840,.T.);
#38249=ADVANCED_FACE('',(#2561),#37841,.F.);
#38250=ADVANCED_FACE('',(#2562),#37842,.F.);
#38251=ADVANCED_FACE('',(#2563),#718,.T.);
#38252=ADVANCED_FACE('',(#2564),#719,.T.);
#38253=ADVANCED_FACE('',(#2565,#203),#720,.T.);
#38254=ADVANCED_FACE('',(#2566,#204,#205,#206,#207,#208,#209,#210,#211,
#212,#213,#214,#215,#216,#217,#218,#219,#220,#221),#721,.T.);
#38255=ADVANCED_FACE('',(#2567),#2300,.F.);
#38256=ADVANCED_FACE('',(#2568),#722,.T.);
#38257=ADVANCED_FACE('',(#2569),#723,.T.);
#38258=ADVANCED_FACE('',(#2570),#724,.T.);
#38259=ADVANCED_FACE('',(#2571),#725,.T.);
#38260=ADVANCED_FACE('',(#2572),#726,.T.);
#38261=ADVANCED_FACE('',(#2573),#727,.T.);
#38262=ADVANCED_FACE('',(#2574),#728,.T.);
#38263=ADVANCED_FACE('',(#2575),#729,.T.);
#38264=ADVANCED_FACE('',(#2576),#730,.T.);
#38265=ADVANCED_FACE('',(#2577),#731,.T.);
#38266=ADVANCED_FACE('',(#2578),#732,.T.);
#38267=ADVANCED_FACE('',(#2579),#2301,.T.);
#38268=ADVANCED_FACE('',(#2580),#2302,.T.);
#38269=ADVANCED_FACE('',(#2581),#2303,.T.);
#38270=ADVANCED_FACE('',(#2582),#2304,.T.);
#38271=ADVANCED_FACE('',(#2583),#2305,.T.);
#38272=ADVANCED_FACE('',(#2584),#2306,.T.);
#38273=ADVANCED_FACE('',(#2585),#2307,.T.);
#38274=ADVANCED_FACE('',(#2586),#2308,.T.);
#38275=ADVANCED_FACE('',(#2587),#2309,.T.);
#38276=ADVANCED_FACE('',(#2588),#2310,.T.);
#38277=ADVANCED_FACE('',(#2589),#2311,.T.);
#38278=ADVANCED_FACE('',(#2590),#2312,.T.);
#38279=ADVANCED_FACE('',(#2591),#2313,.T.);
#38280=ADVANCED_FACE('',(#2592),#2314,.T.);
#38281=ADVANCED_FACE('',(#2593),#2315,.T.);
#38282=ADVANCED_FACE('',(#2594),#2316,.T.);
#38283=ADVANCED_FACE('',(#2595),#2317,.T.);
#38284=ADVANCED_FACE('',(#2596),#2318,.T.);
#38285=ADVANCED_FACE('',(#2597),#2319,.T.);
#38286=ADVANCED_FACE('',(#2598),#2320,.T.);
#38287=ADVANCED_FACE('',(#2599),#2321,.T.);
#38288=ADVANCED_FACE('',(#2600),#2322,.T.);
#38289=ADVANCED_FACE('',(#2601),#2323,.T.);
#38290=ADVANCED_FACE('',(#2602),#2324,.T.);
#38291=ADVANCED_FACE('',(#2603),#2325,.T.);
#38292=ADVANCED_FACE('',(#2604),#2326,.T.);
#38293=ADVANCED_FACE('',(#2605),#2327,.T.);
#38294=ADVANCED_FACE('',(#2606),#2328,.T.);
#38295=ADVANCED_FACE('',(#2607),#2329,.T.);
#38296=ADVANCED_FACE('',(#2608),#2330,.T.);
#38297=ADVANCED_FACE('',(#2609),#37843,.F.);
#38298=ADVANCED_FACE('',(#2610),#37844,.F.);
#38299=ADVANCED_FACE('',(#2611),#37845,.F.);
#38300=ADVANCED_FACE('',(#2612),#37846,.F.);
#38301=ADVANCED_FACE('',(#2613),#37847,.F.);
#38302=ADVANCED_FACE('',(#2614),#37848,.F.);
#38303=ADVANCED_FACE('',(#2615),#37849,.F.);
#38304=ADVANCED_FACE('',(#2616),#37850,.F.);
#38305=ADVANCED_FACE('',(#2617),#37851,.F.);
#38306=ADVANCED_FACE('',(#2618),#37852,.F.);
#38307=ADVANCED_FACE('',(#2619),#37853,.F.);
#38308=ADVANCED_FACE('',(#2620),#37854,.F.);
#38309=ADVANCED_FACE('',(#2621),#37855,.F.);
#38310=ADVANCED_FACE('',(#2622),#37856,.F.);
#38311=ADVANCED_FACE('',(#2623),#37857,.F.);
#38312=ADVANCED_FACE('',(#2624),#37858,.F.);
#38313=ADVANCED_FACE('',(#2625),#37859,.F.);
#38314=ADVANCED_FACE('',(#2626),#37860,.F.);
#38315=ADVANCED_FACE('',(#2627),#37861,.F.);
#38316=ADVANCED_FACE('',(#2628),#37862,.F.);
#38317=ADVANCED_FACE('',(#2629),#37863,.F.);
#38318=ADVANCED_FACE('',(#2630),#37864,.F.);
#38319=ADVANCED_FACE('',(#2631),#37865,.F.);
#38320=ADVANCED_FACE('',(#2632),#37866,.F.);
#38321=ADVANCED_FACE('',(#2633),#37867,.F.);
#38322=ADVANCED_FACE('',(#2634),#37868,.F.);
#38323=ADVANCED_FACE('',(#2635),#37869,.F.);
#38324=ADVANCED_FACE('',(#2636),#37870,.F.);
#38325=ADVANCED_FACE('',(#2637),#37871,.F.);
#38326=ADVANCED_FACE('',(#2638),#37872,.F.);
#38327=ADVANCED_FACE('',(#2639),#37873,.F.);
#38328=ADVANCED_FACE('',(#2640),#37874,.F.);
#38329=ADVANCED_FACE('',(#2641),#37875,.F.);
#38330=ADVANCED_FACE('',(#2642),#37876,.F.);
#38331=ADVANCED_FACE('',(#2643),#37877,.F.);
#38332=ADVANCED_FACE('',(#2644),#37878,.F.);
#38333=ADVANCED_FACE('',(#2645),#37879,.F.);
#38334=ADVANCED_FACE('',(#2646),#37880,.F.);
#38335=ADVANCED_FACE('',(#2647),#37881,.F.);
#38336=ADVANCED_FACE('',(#2648),#37882,.F.);
#38337=ADVANCED_FACE('',(#2649),#37883,.F.);
#38338=ADVANCED_FACE('',(#2650),#37884,.F.);
#38339=ADVANCED_FACE('',(#2651),#37885,.F.);
#38340=ADVANCED_FACE('',(#2652),#37886,.F.);
#38341=ADVANCED_FACE('',(#2653),#37887,.F.);
#38342=ADVANCED_FACE('',(#2654),#37888,.F.);
#38343=ADVANCED_FACE('',(#2655),#37889,.F.);
#38344=ADVANCED_FACE('',(#2656),#37890,.F.);
#38345=ADVANCED_FACE('',(#2657),#37891,.F.);
#38346=ADVANCED_FACE('',(#2658),#37892,.F.);
#38347=ADVANCED_FACE('',(#2659),#37893,.F.);
#38348=ADVANCED_FACE('',(#2660),#37894,.F.);
#38349=ADVANCED_FACE('',(#2661),#37895,.F.);
#38350=ADVANCED_FACE('',(#2662),#37896,.F.);
#38351=ADVANCED_FACE('',(#2663),#37897,.F.);
#38352=ADVANCED_FACE('',(#2664),#733,.F.);
#38353=ADVANCED_FACE('',(#2665),#37898,.F.);
#38354=ADVANCED_FACE('',(#2666),#734,.F.);
#38355=ADVANCED_FACE('',(#2667),#37899,.F.);
#38356=ADVANCED_FACE('',(#2668),#735,.F.);
#38357=ADVANCED_FACE('',(#2669),#37900,.F.);
#38358=ADVANCED_FACE('',(#2670),#736,.F.);
#38359=ADVANCED_FACE('',(#2671),#37901,.F.);
#38360=ADVANCED_FACE('',(#2672),#737,.F.);
#38361=ADVANCED_FACE('',(#2673),#37902,.F.);
#38362=ADVANCED_FACE('',(#2674),#738,.F.);
#38363=ADVANCED_FACE('',(#2675),#739,.F.);
#38364=ADVANCED_FACE('',(#2676),#740,.F.);
#38365=ADVANCED_FACE('',(#2677),#741,.F.);
#38366=ADVANCED_FACE('',(#2678),#742,.F.);
#38367=ADVANCED_FACE('',(#2679),#743,.F.);
#38368=ADVANCED_FACE('',(#2680),#744,.T.);
#38369=ADVANCED_FACE('',(#2681),#745,.F.);
#38370=ADVANCED_FACE('',(#2682),#746,.F.);
#38371=ADVANCED_FACE('',(#2683),#747,.F.);
#38372=ADVANCED_FACE('',(#2684),#37903,.F.);
#38373=ADVANCED_FACE('',(#2685),#748,.T.);
#38374=ADVANCED_FACE('',(#2686),#749,.F.);
#38375=ADVANCED_FACE('',(#2687),#750,.T.);
#38376=ADVANCED_FACE('',(#2688),#37904,.F.);
#38377=ADVANCED_FACE('',(#2689),#751,.F.);
#38378=ADVANCED_FACE('',(#2690),#752,.T.);
#38379=ADVANCED_FACE('',(#2691),#37905,.F.);
#38380=ADVANCED_FACE('',(#2692),#753,.F.);
#38381=ADVANCED_FACE('',(#2693),#37906,.F.);
#38382=ADVANCED_FACE('',(#2694),#754,.T.);
#38383=ADVANCED_FACE('',(#2695),#755,.F.);
#38384=ADVANCED_FACE('',(#2696),#756,.T.);
#38385=ADVANCED_FACE('',(#2697),#37907,.F.);
#38386=ADVANCED_FACE('',(#2698),#757,.F.);
#38387=ADVANCED_FACE('',(#2699),#37908,.F.);
#38388=ADVANCED_FACE('',(#2700),#758,.T.);
#38389=ADVANCED_FACE('',(#2701),#759,.F.);
#38390=ADVANCED_FACE('',(#2702),#37909,.F.);
#38391=ADVANCED_FACE('',(#2703),#760,.T.);
#38392=ADVANCED_FACE('',(#2704),#761,.F.);
#38393=ADVANCED_FACE('',(#2705),#762,.T.);
#38394=ADVANCED_FACE('',(#2706),#37910,.F.);
#38395=ADVANCED_FACE('',(#2707),#763,.F.);
#38396=ADVANCED_FACE('',(#2708),#764,.T.);
#38397=ADVANCED_FACE('',(#2709),#37911,.F.);
#38398=ADVANCED_FACE('',(#2710),#765,.F.);
#38399=ADVANCED_FACE('',(#2711),#766,.T.);
#38400=ADVANCED_FACE('',(#2712),#37912,.F.);
#38401=ADVANCED_FACE('',(#2713),#767,.F.);
#38402=ADVANCED_FACE('',(#2714),#768,.T.);
#38403=ADVANCED_FACE('',(#2715),#37913,.F.);
#38404=ADVANCED_FACE('',(#2716),#769,.F.);
#38405=ADVANCED_FACE('',(#2717),#37914,.F.);
#38406=ADVANCED_FACE('',(#2718),#770,.T.);
#38407=ADVANCED_FACE('',(#2719),#771,.F.);
#38408=ADVANCED_FACE('',(#2720),#37915,.F.);
#38409=ADVANCED_FACE('',(#2721),#772,.T.);
#38410=ADVANCED_FACE('',(#2722),#773,.F.);
#38411=ADVANCED_FACE('',(#2723),#37916,.F.);
#38412=ADVANCED_FACE('',(#2724),#774,.T.);
#38413=ADVANCED_FACE('',(#2725),#775,.F.);
#38414=ADVANCED_FACE('',(#2726),#37917,.F.);
#38415=ADVANCED_FACE('',(#2727),#776,.T.);
#38416=ADVANCED_FACE('',(#2728),#777,.F.);
#38417=ADVANCED_FACE('',(#2729),#37918,.F.);
#38418=ADVANCED_FACE('',(#2730),#778,.T.);
#38419=ADVANCED_FACE('',(#2731),#779,.F.);
#38420=ADVANCED_FACE('',(#2732),#37919,.F.);
#38421=ADVANCED_FACE('',(#2733),#780,.T.);
#38422=ADVANCED_FACE('',(#2734),#781,.F.);
#38423=ADVANCED_FACE('',(#2735),#37920,.F.);
#38424=ADVANCED_FACE('',(#2736),#782,.T.);
#38425=ADVANCED_FACE('',(#2737),#783,.F.);
#38426=ADVANCED_FACE('',(#2738),#784,.T.);
#38427=ADVANCED_FACE('',(#2739),#37921,.F.);
#38428=ADVANCED_FACE('',(#2740),#785,.F.);
#38429=ADVANCED_FACE('',(#2741),#786,.T.);
#38430=ADVANCED_FACE('',(#2742),#37922,.F.);
#38431=ADVANCED_FACE('',(#2743),#787,.F.);
#38432=ADVANCED_FACE('',(#2744),#788,.T.);
#38433=ADVANCED_FACE('',(#2745),#37923,.F.);
#38434=ADVANCED_FACE('',(#2746),#789,.F.);
#38435=ADVANCED_FACE('',(#2747),#790,.T.);
#38436=ADVANCED_FACE('',(#2748),#37924,.F.);
#38437=ADVANCED_FACE('',(#2749),#791,.F.);
#38438=ADVANCED_FACE('',(#2750),#792,.T.);
#38439=ADVANCED_FACE('',(#2751),#37925,.F.);
#38440=ADVANCED_FACE('',(#2752),#793,.F.);
#38441=ADVANCED_FACE('',(#2753),#37926,.F.);
#38442=ADVANCED_FACE('',(#2754),#794,.T.);
#38443=ADVANCED_FACE('',(#2755),#795,.F.);
#38444=ADVANCED_FACE('',(#2756),#37927,.F.);
#38445=ADVANCED_FACE('',(#2757),#796,.T.);
#38446=ADVANCED_FACE('',(#2758),#797,.T.);
#38447=ADVANCED_FACE('',(#2759),#37928,.F.);
#38448=ADVANCED_FACE('',(#2760),#798,.F.);
#38449=ADVANCED_FACE('',(#2761),#799,.T.);
#38450=ADVANCED_FACE('',(#2762),#37929,.F.);
#38451=ADVANCED_FACE('',(#2763),#800,.F.);
#38452=ADVANCED_FACE('',(#2764),#801,.F.);
#38453=ADVANCED_FACE('',(#2765),#37930,.F.);
#38454=ADVANCED_FACE('',(#2766),#802,.T.);
#38455=ADVANCED_FACE('',(#2767),#803,.T.);
#38456=ADVANCED_FACE('',(#2768),#37931,.F.);
#38457=ADVANCED_FACE('',(#2769),#804,.F.);
#38458=ADVANCED_FACE('',(#2770),#805,.F.);
#38459=ADVANCED_FACE('',(#2771),#37932,.F.);
#38460=ADVANCED_FACE('',(#2772),#806,.T.);
#38461=ADVANCED_FACE('',(#2773),#807,.F.);
#38462=ADVANCED_FACE('',(#2774),#37933,.F.);
#38463=ADVANCED_FACE('',(#2775),#808,.T.);
#38464=ADVANCED_FACE('',(#2776),#809,.T.);
#38465=ADVANCED_FACE('',(#2777),#37934,.F.);
#38466=ADVANCED_FACE('',(#2778),#810,.F.);
#38467=ADVANCED_FACE('',(#2779),#811,.T.);
#38468=ADVANCED_FACE('',(#2780),#37935,.F.);
#38469=ADVANCED_FACE('',(#2781),#812,.F.);
#38470=ADVANCED_FACE('',(#2782),#813,.T.);
#38471=ADVANCED_FACE('',(#2783),#37936,.F.);
#38472=ADVANCED_FACE('',(#2784),#814,.F.);
#38473=ADVANCED_FACE('',(#2785),#815,.T.);
#38474=ADVANCED_FACE('',(#2786),#37937,.F.);
#38475=ADVANCED_FACE('',(#2787),#816,.F.);
#38476=ADVANCED_FACE('',(#2788),#817,.F.);
#38477=ADVANCED_FACE('',(#2789),#37938,.F.);
#38478=ADVANCED_FACE('',(#2790),#818,.T.);
#38479=ADVANCED_FACE('',(#2791),#819,.F.);
#38480=ADVANCED_FACE('',(#2792),#37939,.F.);
#38481=ADVANCED_FACE('',(#2793),#820,.T.);
#38482=ADVANCED_FACE('',(#2794),#821,.F.);
#38483=ADVANCED_FACE('',(#2795),#37940,.F.);
#38484=ADVANCED_FACE('',(#2796),#822,.T.);
#38485=ADVANCED_FACE('',(#2797),#823,.F.);
#38486=ADVANCED_FACE('',(#2798),#37941,.F.);
#38487=ADVANCED_FACE('',(#2799),#824,.T.);
#38488=ADVANCED_FACE('',(#2800),#825,.F.);
#38489=ADVANCED_FACE('',(#2801),#37942,.F.);
#38490=ADVANCED_FACE('',(#2802),#826,.T.);
#38491=ADVANCED_FACE('',(#2803),#827,.F.);
#38492=ADVANCED_FACE('',(#2804),#37943,.F.);
#38493=ADVANCED_FACE('',(#2805),#828,.T.);
#38494=ADVANCED_FACE('',(#2806),#829,.F.);
#38495=ADVANCED_FACE('',(#2807),#37944,.F.);
#38496=ADVANCED_FACE('',(#2808),#830,.T.);
#38497=ADVANCED_FACE('',(#2809),#831,.T.);
#38498=ADVANCED_FACE('',(#2810),#37945,.F.);
#38499=ADVANCED_FACE('',(#2811),#832,.F.);
#38500=ADVANCED_FACE('',(#2812),#833,.T.);
#38501=ADVANCED_FACE('',(#2813),#37946,.F.);
#38502=ADVANCED_FACE('',(#2814),#834,.F.);
#38503=ADVANCED_FACE('',(#2815),#835,.T.);
#38504=ADVANCED_FACE('',(#2816),#37947,.F.);
#38505=ADVANCED_FACE('',(#2817),#836,.F.);
#38506=ADVANCED_FACE('',(#2818),#837,.T.);
#38507=ADVANCED_FACE('',(#2819),#37948,.F.);
#38508=ADVANCED_FACE('',(#2820),#838,.F.);
#38509=ADVANCED_FACE('',(#2821),#839,.T.);
#38510=ADVANCED_FACE('',(#2822),#37949,.F.);
#38511=ADVANCED_FACE('',(#2823),#840,.F.);
#38512=ADVANCED_FACE('',(#2824),#841,.F.);
#38513=ADVANCED_FACE('',(#2825),#37950,.F.);
#38514=ADVANCED_FACE('',(#2826),#842,.T.);
#38515=ADVANCED_FACE('',(#2827),#843,.T.);
#38516=ADVANCED_FACE('',(#2828),#844,.T.);
#38517=ADVANCED_FACE('',(#2829),#845,.T.);
#38518=ADVANCED_FACE('',(#2830),#846,.T.);
#38519=ADVANCED_FACE('',(#2831),#847,.T.);
#38520=ADVANCED_FACE('',(#2832),#848,.T.);
#38521=ADVANCED_FACE('',(#2833),#849,.T.);
#38522=ADVANCED_FACE('',(#2834),#850,.F.);
#38523=ADVANCED_FACE('',(#2835),#37951,.T.);
#38524=ADVANCED_FACE('',(#2836),#37952,.F.);
#38525=ADVANCED_FACE('',(#2837),#851,.F.);
#38526=ADVANCED_FACE('',(#2838),#852,.F.);
#38527=ADVANCED_FACE('',(#2839),#37953,.T.);
#38528=ADVANCED_FACE('',(#2840),#853,.F.);
#38529=ADVANCED_FACE('',(#2841),#37954,.T.);
#38530=ADVANCED_FACE('',(#2842),#854,.T.);
#38531=ADVANCED_FACE('',(#2843),#855,.F.);
#38532=ADVANCED_FACE('',(#2844),#37955,.T.);
#38533=ADVANCED_FACE('',(#2845),#37956,.T.);
#38534=ADVANCED_FACE('',(#2846),#856,.F.);
#38535=ADVANCED_FACE('',(#2847),#857,.T.);
#38536=ADVANCED_FACE('',(#2848),#37957,.F.);
#38537=ADVANCED_FACE('',(#2849),#37958,.F.);
#38538=ADVANCED_FACE('',(#2850),#858,.F.);
#38539=ADVANCED_FACE('',(#2851),#859,.F.);
#38540=ADVANCED_FACE('',(#2852,#222),#860,.F.);
#38541=ADVANCED_FACE('',(#2853),#37959,.T.);
#38542=ADVANCED_FACE('',(#2854),#37960,.T.);
#38543=ADVANCED_FACE('',(#2855),#37961,.F.);
#38544=ADVANCED_FACE('',(#2856),#37962,.F.);
#38545=ADVANCED_FACE('',(#2857),#861,.T.);
#38546=ADVANCED_FACE('',(#2858),#862,.T.);
#38547=ADVANCED_FACE('',(#2859,#223),#863,.T.);
#38548=ADVANCED_FACE('',(#2860),#864,.T.);
#38549=ADVANCED_FACE('',(#2861),#865,.F.);
#38550=ADVANCED_FACE('',(#2862),#37963,.T.);
#38551=ADVANCED_FACE('',(#2863),#37964,.T.);
#38552=ADVANCED_FACE('',(#2864),#866,.T.);
#38553=ADVANCED_FACE('',(#2865),#867,.F.);
#38554=ADVANCED_FACE('',(#2866),#37965,.F.);
#38555=ADVANCED_FACE('',(#2867),#37966,.F.);
#38556=ADVANCED_FACE('',(#2868),#868,.F.);
#38557=ADVANCED_FACE('',(#2869),#869,.F.);
#38558=ADVANCED_FACE('',(#2870,#224),#870,.F.);
#38559=ADVANCED_FACE('',(#2871),#37967,.T.);
#38560=ADVANCED_FACE('',(#2872),#37968,.T.);
#38561=ADVANCED_FACE('',(#2873),#37969,.F.);
#38562=ADVANCED_FACE('',(#2874),#37970,.F.);
#38563=ADVANCED_FACE('',(#2875),#871,.T.);
#38564=ADVANCED_FACE('',(#2876),#872,.T.);
#38565=ADVANCED_FACE('',(#2877,#225),#873,.T.);
#38566=ADVANCED_FACE('',(#2878),#874,.T.);
#38567=ADVANCED_FACE('',(#2879),#875,.T.);
#38568=ADVANCED_FACE('',(#2880),#876,.T.);
#38569=ADVANCED_FACE('',(#2881),#877,.T.);
#38570=ADVANCED_FACE('',(#2882),#878,.T.);
#38571=ADVANCED_FACE('',(#2883),#879,.T.);
#38572=ADVANCED_FACE('',(#2884),#880,.T.);
#38573=ADVANCED_FACE('',(#2885),#881,.F.);
#38574=ADVANCED_FACE('',(#2886),#37971,.T.);
#38575=ADVANCED_FACE('',(#2887),#37972,.F.);
#38576=ADVANCED_FACE('',(#2888),#882,.T.);
#38577=ADVANCED_FACE('',(#2889),#883,.T.);
#38578=ADVANCED_FACE('',(#2890),#884,.F.);
#38579=ADVANCED_FACE('',(#2891),#885,.T.);
#38580=ADVANCED_FACE('',(#2892),#37973,.T.);
#38581=ADVANCED_FACE('',(#2893),#886,.T.);
#38582=ADVANCED_FACE('',(#2894),#37974,.T.);
#39933=CLOSED_SHELL('',(#38019,#38020,#38021,#38022,#38023,#38024,#38025,
#38026,#38027,#38028,#38029,#38030,#38031,#38032,#38033,#38034,#38035,#38036,
#38037,#38038,#38039,#38040,#38041,#38042,#38043,#38044,#38045,#38046,#38047,
#38048,#38049,#38050,#38051,#38052,#38053,#38054,#38055,#38056,#38057,#38058,
#38059,#38060,#38061,#38062,#38063,#38064,#38065,#38066,#38067,#38068,#38069,
#38070,#38071,#38072,#38073,#38074,#38075,#38076,#38077,#38078,#38079,#38080,
#38081,#38082,#38083,#38084,#38085,#38086,#38087,#38088,#38089,#38090,#38091,
#38092,#38093,#38094,#38095,#38096,#38097,#38098,#38099,#38100,#38101,#38102,
#38103,#38104,#38105,#38106,#38107,#38108,#38109,#38110,#38111,#38112,#38113,
#38114,#38115,#38116,#38117,#38118,#38119,#38120,#38121,#38122,#38123,#38124,
#38125,#38126,#38127,#38128,#38129,#38130,#38131,#38132,#38133,#38134,#38135,
#38136,#38137,#38138,#38139,#38140,#38141,#38142,#38143,#38144,#38145,#38146,
#38147,#38148,#38149,#38150,#38151,#38152,#38153,#38154,#38155,#38156,#38157,
#38158,#38159,#38160,#38161,#38162,#38163,#38164,#38165,#38166,#38167,#38168,
#38169,#38170,#38171,#38172,#38173,#38174,#38175,#38176,#38177,#38178,#38179,
#38180,#38181,#38182,#38183,#38184,#38185,#38186,#38187,#38188,#38189,#38190,
#38191,#38192,#38193,#38194,#38195,#38196,#38197,#38198,#38199,#38200,#38201,
#38202,#38203,#38204,#38205,#38206,#38207,#38208,#38209,#38210,#38211,#38212,
#38213,#38214,#38215,#38216,#38217,#38218,#38219,#38220,#38221,#38222,#38223,
#38224,#38225,#38226,#38227,#38228,#38229,#38230,#38231,#38232,#38233,#38234,
#38235,#38236,#38237,#38238,#38239,#38240,#38241,#38242,#38243,#38244,#38245,
#38246,#38247,#38248,#38249,#38250,#38251,#38252,#38253,#38254,#38255,#38256,
#38257,#38258,#38259,#38260,#38261,#38262,#38263,#38264,#38265,#38266,#38267,
#38268,#38269,#38270,#38271,#38272,#38273,#38274,#38275,#38276,#38277,#38278,
#38279,#38280,#38281,#38282,#38283,#38284,#38285,#38286,#38287,#38288,#38289,
#38290,#38291,#38292,#38293,#38294,#38295,#38296,#38297,#38298,#38299,#38300,
#38301,#38302,#38303,#38304,#38305,#38306,#38307,#38308,#38309,#38310,#38311,
#38312,#38313,#38314,#38315,#38316,#38317,#38318,#38319,#38320,#38321,#38322,
#38323,#38324,#38325,#38326,#38327,#38328,#38329,#38330,#38331,#38332,#38333,
#38334,#38335,#38336,#38337,#38338,#38339,#38340,#38341,#38342,#38343,#38344,
#38345,#38346,#38347,#38348,#38349,#38350,#38351,#38352,#38353,#38354,#38355,
#38356,#38357,#38358,#38359,#38360,#38361,#38362,#38363,#38364,#38365,#38366,
#38367,#38368,#38369,#38370,#38371,#38372,#38373,#38374,#38375,#38376,#38377,
#38378,#38379,#38380,#38381,#38382,#38383,#38384,#38385,#38386,#38387,#38388,
#38389,#38390,#38391,#38392,#38393,#38394,#38395,#38396,#38397,#38398,#38399,
#38400,#38401,#38402,#38403,#38404,#38405,#38406,#38407,#38408,#38409,#38410,
#38411,#38412,#38413,#38414,#38415,#38416,#38417,#38418,#38419,#38420,#38421,
#38422,#38423,#38424,#38425,#38426,#38427,#38428,#38429,#38430,#38431,#38432,
#38433,#38434,#38435,#38436,#38437,#38438,#38439,#38440,#38441,#38442,#38443,
#38444,#38445,#38446,#38447,#38448,#38449,#38450,#38451,#38452,#38453,#38454,
#38455,#38456,#38457,#38458,#38459,#38460,#38461,#38462,#38463,#38464,#38465,
#38466,#38467,#38468,#38469,#38470,#38471,#38472,#38473,#38474,#38475,#38476,
#38477,#38478,#38479,#38480,#38481,#38482,#38483,#38484,#38485,#38486,#38487,
#38488,#38489,#38490,#38491,#38492,#38493,#38494,#38495,#38496,#38497,#38498,
#38499,#38500,#38501,#38502,#38503,#38504,#38505,#38506,#38507,#38508,#38509,
#38510,#38511,#38512,#38513,#38514,#38515,#38516,#38517,#38518,#38519,#38520,
#38521,#38522,#38523,#38524,#38525,#38526,#38527,#38528,#38529,#38530,#38531,
#38532,#38533,#38534,#38535,#38536,#38537,#38538,#38539,#38540,#38541,#38542,
#38543,#38544,#38545,#38546,#38547,#38548,#38549,#38550,#38551,#38552,#38553,
#38554,#38555,#38556,#38557,#38558,#38559,#38560,#38561,#38562,#38563,#38564,
#38565,#38566,#38567,#38568,#38569,#38570,#38571,#38572,#38573,#38574,#38575,
#38576,#38577,#38578,#38579,#38580,#38581,#38582));
#39984=AXIS2_PLACEMENT_3D('',#52452,#42516,#42517);
#39985=AXIS2_PLACEMENT_3D('',#52453,#42518,#42519);
#39986=AXIS2_PLACEMENT_3D('',#52455,#42520,#42521);
#39987=AXIS2_PLACEMENT_3D('',#52458,#42523,#42524);
#39988=AXIS2_PLACEMENT_3D('',#52459,#42525,#42526);
#39989=AXIS2_PLACEMENT_3D('',#52461,#42527,#42528);
#39990=AXIS2_PLACEMENT_3D('',#52464,#42530,#42531);
#39991=AXIS2_PLACEMENT_3D('',#52465,#42532,#42533);
#39992=AXIS2_PLACEMENT_3D('',#52467,#42534,#42535);
#39993=AXIS2_PLACEMENT_3D('',#52470,#42537,#42538);
#39994=AXIS2_PLACEMENT_3D('',#52471,#42539,#42540);
#39995=AXIS2_PLACEMENT_3D('',#52473,#42541,#42542);
#39996=AXIS2_PLACEMENT_3D('',#52476,#42544,#42545);
#39997=AXIS2_PLACEMENT_3D('',#52477,#42546,#42547);
#39998=AXIS2_PLACEMENT_3D('',#52479,#42548,#42549);
#39999=AXIS2_PLACEMENT_3D('',#52482,#42551,#42552);
#40000=AXIS2_PLACEMENT_3D('',#52483,#42553,#42554);
#40001=AXIS2_PLACEMENT_3D('',#52485,#42555,#42556);
#40002=AXIS2_PLACEMENT_3D('',#52488,#42558,#42559);
#40003=AXIS2_PLACEMENT_3D('',#52489,#42560,#42561);
#40004=AXIS2_PLACEMENT_3D('',#52492,#42562,#42563);
#40005=AXIS2_PLACEMENT_3D('',#52496,#42565,#42566);
#40006=AXIS2_PLACEMENT_3D('',#52498,#42568,#42569);
#40007=AXIS2_PLACEMENT_3D('',#52501,#42570,#42571);
#40008=AXIS2_PLACEMENT_3D('',#52505,#42573,#42574);
#40009=AXIS2_PLACEMENT_3D('',#52507,#42576,#42577);
#40010=AXIS2_PLACEMENT_3D('',#52510,#42578,#42579);
#40011=AXIS2_PLACEMENT_3D('',#52514,#42581,#42582);
#40012=AXIS2_PLACEMENT_3D('',#52516,#42584,#42585);
#40013=AXIS2_PLACEMENT_3D('',#52519,#42586,#42587);
#40014=AXIS2_PLACEMENT_3D('',#52523,#42589,#42590);
#40015=AXIS2_PLACEMENT_3D('',#52525,#42592,#42593);
#40016=AXIS2_PLACEMENT_3D('',#52528,#42594,#42595);
#40017=AXIS2_PLACEMENT_3D('',#52532,#42597,#42598);
#40018=AXIS2_PLACEMENT_3D('',#52534,#42600,#42601);
#40019=AXIS2_PLACEMENT_3D('',#52537,#42602,#42603);
#40020=AXIS2_PLACEMENT_3D('',#52541,#42605,#42606);
#40021=AXIS2_PLACEMENT_3D('',#52543,#42608,#42609);
#40022=AXIS2_PLACEMENT_3D('',#52546,#42610,#42611);
#40023=AXIS2_PLACEMENT_3D('',#52550,#42613,#42614);
#40024=AXIS2_PLACEMENT_3D('',#52552,#42616,#42617);
#40025=AXIS2_PLACEMENT_3D('',#52555,#42618,#42619);
#40026=AXIS2_PLACEMENT_3D('',#52559,#42621,#42622);
#40027=AXIS2_PLACEMENT_3D('',#52561,#42624,#42625);
#40028=AXIS2_PLACEMENT_3D('',#52564,#42626,#42627);
#40029=AXIS2_PLACEMENT_3D('',#52568,#42629,#42630);
#40030=AXIS2_PLACEMENT_3D('',#52570,#42632,#42633);
#40031=AXIS2_PLACEMENT_3D('',#52573,#42634,#42635);
#40032=AXIS2_PLACEMENT_3D('',#52577,#42637,#42638);
#40033=AXIS2_PLACEMENT_3D('',#52579,#42640,#42641);
#40034=AXIS2_PLACEMENT_3D('',#52582,#42642,#42643);
#40035=AXIS2_PLACEMENT_3D('',#52586,#42645,#42646);
#40036=AXIS2_PLACEMENT_3D('',#52588,#42648,#42649);
#40037=AXIS2_PLACEMENT_3D('',#52591,#42650,#42651);
#40038=AXIS2_PLACEMENT_3D('',#52595,#42653,#42654);
#40039=AXIS2_PLACEMENT_3D('',#52597,#42656,#42657);
#40040=AXIS2_PLACEMENT_3D('',#52600,#42658,#42659);
#40041=AXIS2_PLACEMENT_3D('',#52604,#42661,#42662);
#40042=AXIS2_PLACEMENT_3D('',#52606,#42664,#42665);
#40043=AXIS2_PLACEMENT_3D('',#52609,#42666,#42667);
#40044=AXIS2_PLACEMENT_3D('',#52613,#42669,#42670);
#40045=AXIS2_PLACEMENT_3D('',#52615,#42672,#42673);
#40046=AXIS2_PLACEMENT_3D('',#52618,#42674,#42675);
#40047=AXIS2_PLACEMENT_3D('',#52622,#42677,#42678);
#40048=AXIS2_PLACEMENT_3D('',#52624,#42680,#42681);
#40049=AXIS2_PLACEMENT_3D('',#52627,#42682,#42683);
#40050=AXIS2_PLACEMENT_3D('',#52631,#42685,#42686);
#40051=AXIS2_PLACEMENT_3D('',#52633,#42688,#42689);
#40052=AXIS2_PLACEMENT_3D('',#52636,#42690,#42691);
#40053=AXIS2_PLACEMENT_3D('',#52640,#42693,#42694);
#40054=AXIS2_PLACEMENT_3D('',#52642,#42696,#42697);
#40055=AXIS2_PLACEMENT_3D('',#52645,#42698,#42699);
#40056=AXIS2_PLACEMENT_3D('',#52649,#42701,#42702);
#40057=AXIS2_PLACEMENT_3D('',#52651,#42704,#42705);
#40058=AXIS2_PLACEMENT_3D('',#52654,#42706,#42707);
#40059=AXIS2_PLACEMENT_3D('',#52658,#42709,#42710);
#40060=AXIS2_PLACEMENT_3D('',#52660,#42712,#42713);
#40061=AXIS2_PLACEMENT_3D('',#52663,#42714,#42715);
#40062=AXIS2_PLACEMENT_3D('',#52667,#42717,#42718);
#40063=AXIS2_PLACEMENT_3D('',#52669,#42720,#42721);
#40064=AXIS2_PLACEMENT_3D('',#52672,#42722,#42723);
#40065=AXIS2_PLACEMENT_3D('',#52676,#42725,#42726);
#40066=AXIS2_PLACEMENT_3D('',#52678,#42728,#42729);
#40067=AXIS2_PLACEMENT_3D('',#52681,#42730,#42731);
#40068=AXIS2_PLACEMENT_3D('',#52685,#42733,#42734);
#40069=AXIS2_PLACEMENT_3D('',#52687,#42736,#42737);
#40070=AXIS2_PLACEMENT_3D('',#52690,#42738,#42739);
#40071=AXIS2_PLACEMENT_3D('',#52694,#42741,#42742);
#40072=AXIS2_PLACEMENT_3D('',#52696,#42744,#42745);
#40073=AXIS2_PLACEMENT_3D('',#52699,#42746,#42747);
#40074=AXIS2_PLACEMENT_3D('',#52703,#42749,#42750);
#40075=AXIS2_PLACEMENT_3D('',#52705,#42752,#42753);
#40076=AXIS2_PLACEMENT_3D('',#52708,#42754,#42755);
#40077=AXIS2_PLACEMENT_3D('',#52712,#42757,#42758);
#40078=AXIS2_PLACEMENT_3D('',#52714,#42760,#42761);
#40079=AXIS2_PLACEMENT_3D('',#52717,#42762,#42763);
#40080=AXIS2_PLACEMENT_3D('',#52721,#42765,#42766);
#40081=AXIS2_PLACEMENT_3D('',#52723,#42768,#42769);
#40082=AXIS2_PLACEMENT_3D('',#52726,#42770,#42771);
#40083=AXIS2_PLACEMENT_3D('',#52730,#42773,#42774);
#40084=AXIS2_PLACEMENT_3D('',#52732,#42776,#42777);
#40085=AXIS2_PLACEMENT_3D('',#52735,#42778,#42779);
#40086=AXIS2_PLACEMENT_3D('',#52739,#42781,#42782);
#40087=AXIS2_PLACEMENT_3D('',#52741,#42784,#42785);
#40088=AXIS2_PLACEMENT_3D('',#52744,#42786,#42787);
#40089=AXIS2_PLACEMENT_3D('',#52748,#42789,#42790);
#40090=AXIS2_PLACEMENT_3D('',#52750,#42792,#42793);
#40091=AXIS2_PLACEMENT_3D('',#52753,#42794,#42795);
#40092=AXIS2_PLACEMENT_3D('',#52757,#42797,#42798);
#40093=AXIS2_PLACEMENT_3D('',#52759,#42800,#42801);
#40094=AXIS2_PLACEMENT_3D('',#52762,#42802,#42803);
#40095=AXIS2_PLACEMENT_3D('',#52766,#42805,#42806);
#40096=AXIS2_PLACEMENT_3D('',#52768,#42808,#42809);
#40097=AXIS2_PLACEMENT_3D('',#52771,#42810,#42811);
#40098=AXIS2_PLACEMENT_3D('',#52775,#42813,#42814);
#40099=AXIS2_PLACEMENT_3D('',#52777,#42816,#42817);
#40100=AXIS2_PLACEMENT_3D('',#52780,#42818,#42819);
#40101=AXIS2_PLACEMENT_3D('',#52784,#42821,#42822);
#40102=AXIS2_PLACEMENT_3D('',#52786,#42824,#42825);
#40103=AXIS2_PLACEMENT_3D('',#52789,#42826,#42827);
#40104=AXIS2_PLACEMENT_3D('',#52793,#42829,#42830);
#40105=AXIS2_PLACEMENT_3D('',#52795,#42832,#42833);
#40106=AXIS2_PLACEMENT_3D('',#52798,#42834,#42835);
#40107=AXIS2_PLACEMENT_3D('',#52802,#42837,#42838);
#40108=AXIS2_PLACEMENT_3D('',#52804,#42840,#42841);
#40109=AXIS2_PLACEMENT_3D('',#52807,#42842,#42843);
#40110=AXIS2_PLACEMENT_3D('',#52811,#42845,#42846);
#40111=AXIS2_PLACEMENT_3D('',#52813,#42848,#42849);
#40112=AXIS2_PLACEMENT_3D('',#52816,#42850,#42851);
#40113=AXIS2_PLACEMENT_3D('',#52820,#42853,#42854);
#40114=AXIS2_PLACEMENT_3D('',#52822,#42856,#42857);
#40115=AXIS2_PLACEMENT_3D('',#52825,#42858,#42859);
#40116=AXIS2_PLACEMENT_3D('',#52829,#42861,#42862);
#40117=AXIS2_PLACEMENT_3D('',#52831,#42864,#42865);
#40118=AXIS2_PLACEMENT_3D('',#52834,#42866,#42867);
#40119=AXIS2_PLACEMENT_3D('',#52838,#42869,#42870);
#40120=AXIS2_PLACEMENT_3D('',#52840,#42872,#42873);
#40121=AXIS2_PLACEMENT_3D('',#52843,#42874,#42875);
#40122=AXIS2_PLACEMENT_3D('',#52847,#42877,#42878);
#40123=AXIS2_PLACEMENT_3D('',#52849,#42880,#42881);
#40124=AXIS2_PLACEMENT_3D('',#52852,#42882,#42883);
#40125=AXIS2_PLACEMENT_3D('',#52856,#42885,#42886);
#40126=AXIS2_PLACEMENT_3D('',#52858,#42888,#42889);
#40127=AXIS2_PLACEMENT_3D('',#52861,#42890,#42891);
#40128=AXIS2_PLACEMENT_3D('',#52865,#42893,#42894);
#40129=AXIS2_PLACEMENT_3D('',#52867,#42896,#42897);
#40130=AXIS2_PLACEMENT_3D('',#52870,#42898,#42899);
#40131=AXIS2_PLACEMENT_3D('',#52874,#42901,#42902);
#40132=AXIS2_PLACEMENT_3D('',#52876,#42904,#42905);
#40133=AXIS2_PLACEMENT_3D('',#52879,#42906,#42907);
#40134=AXIS2_PLACEMENT_3D('',#52883,#42909,#42910);
#40135=AXIS2_PLACEMENT_3D('',#52885,#42912,#42913);
#40136=AXIS2_PLACEMENT_3D('',#52888,#42914,#42915);
#40137=AXIS2_PLACEMENT_3D('',#52892,#42917,#42918);
#40138=AXIS2_PLACEMENT_3D('',#52894,#42920,#42921);
#40139=AXIS2_PLACEMENT_3D('',#52897,#42922,#42923);
#40140=AXIS2_PLACEMENT_3D('',#52901,#42925,#42926);
#40141=AXIS2_PLACEMENT_3D('',#52903,#42928,#42929);
#40142=AXIS2_PLACEMENT_3D('',#52906,#42930,#42931);
#40143=AXIS2_PLACEMENT_3D('',#52910,#42933,#42934);
#40144=AXIS2_PLACEMENT_3D('',#52912,#42936,#42937);
#40145=AXIS2_PLACEMENT_3D('',#52915,#42938,#42939);
#40146=AXIS2_PLACEMENT_3D('',#52919,#42941,#42942);
#40147=AXIS2_PLACEMENT_3D('',#52921,#42944,#42945);
#40148=AXIS2_PLACEMENT_3D('',#52924,#42946,#42947);
#40149=AXIS2_PLACEMENT_3D('',#52928,#42949,#42950);
#40150=AXIS2_PLACEMENT_3D('',#52930,#42952,#42953);
#40151=AXIS2_PLACEMENT_3D('',#52933,#42954,#42955);
#40152=AXIS2_PLACEMENT_3D('',#52937,#42957,#42958);
#40153=AXIS2_PLACEMENT_3D('',#52939,#42960,#42961);
#40154=AXIS2_PLACEMENT_3D('',#52942,#42962,#42963);
#40155=AXIS2_PLACEMENT_3D('',#52946,#42965,#42966);
#40156=AXIS2_PLACEMENT_3D('',#52948,#42968,#42969);
#40157=AXIS2_PLACEMENT_3D('',#52951,#42970,#42971);
#40158=AXIS2_PLACEMENT_3D('',#52955,#42973,#42974);
#40159=AXIS2_PLACEMENT_3D('',#52957,#42976,#42977);
#40160=AXIS2_PLACEMENT_3D('',#52960,#42978,#42979);
#40161=AXIS2_PLACEMENT_3D('',#52964,#42981,#42982);
#40162=AXIS2_PLACEMENT_3D('',#52966,#42984,#42985);
#40163=AXIS2_PLACEMENT_3D('',#52969,#42986,#42987);
#40164=AXIS2_PLACEMENT_3D('',#52973,#42989,#42990);
#40165=AXIS2_PLACEMENT_3D('',#52975,#42992,#42993);
#40166=AXIS2_PLACEMENT_3D('',#52978,#42994,#42995);
#40167=AXIS2_PLACEMENT_3D('',#52982,#42997,#42998);
#40168=AXIS2_PLACEMENT_3D('',#52984,#43000,#43001);
#40169=AXIS2_PLACEMENT_3D('',#52987,#43002,#43003);
#40170=AXIS2_PLACEMENT_3D('',#52991,#43005,#43006);
#40171=AXIS2_PLACEMENT_3D('',#52993,#43008,#43009);
#40172=AXIS2_PLACEMENT_3D('',#52996,#43010,#43011);
#40173=AXIS2_PLACEMENT_3D('',#53000,#43013,#43014);
#40174=AXIS2_PLACEMENT_3D('',#53002,#43016,#43017);
#40175=AXIS2_PLACEMENT_3D('',#53005,#43018,#43019);
#40176=AXIS2_PLACEMENT_3D('',#53009,#43021,#43022);
#40177=AXIS2_PLACEMENT_3D('',#53011,#43024,#43025);
#40178=AXIS2_PLACEMENT_3D('',#53014,#43026,#43027);
#40179=AXIS2_PLACEMENT_3D('',#53018,#43029,#43030);
#40180=AXIS2_PLACEMENT_3D('',#53020,#43032,#43033);
#40181=AXIS2_PLACEMENT_3D('',#53023,#43034,#43035);
#40182=AXIS2_PLACEMENT_3D('',#53027,#43037,#43038);
#40183=AXIS2_PLACEMENT_3D('',#53029,#43040,#43041);
#40184=AXIS2_PLACEMENT_3D('',#53032,#43042,#43043);
#40185=AXIS2_PLACEMENT_3D('',#53036,#43045,#43046);
#40186=AXIS2_PLACEMENT_3D('',#53038,#43048,#43049);
#40187=AXIS2_PLACEMENT_3D('',#53041,#43050,#43051);
#40188=AXIS2_PLACEMENT_3D('',#53045,#43053,#43054);
#40189=AXIS2_PLACEMENT_3D('',#53047,#43056,#43057);
#40190=AXIS2_PLACEMENT_3D('',#53050,#43058,#43059);
#40191=AXIS2_PLACEMENT_3D('',#53054,#43061,#43062);
#40192=AXIS2_PLACEMENT_3D('',#53056,#43064,#43065);
#40193=AXIS2_PLACEMENT_3D('',#53059,#43066,#43067);
#40194=AXIS2_PLACEMENT_3D('',#53063,#43069,#43070);
#40195=AXIS2_PLACEMENT_3D('',#53065,#43072,#43073);
#40196=AXIS2_PLACEMENT_3D('',#53068,#43074,#43075);
#40197=AXIS2_PLACEMENT_3D('',#53072,#43077,#43078);
#40198=AXIS2_PLACEMENT_3D('',#53074,#43080,#43081);
#40199=AXIS2_PLACEMENT_3D('',#53077,#43082,#43083);
#40200=AXIS2_PLACEMENT_3D('',#53081,#43085,#43086);
#40201=AXIS2_PLACEMENT_3D('',#53225,#43098,#43099);
#40202=AXIS2_PLACEMENT_3D('',#53227,#43100,#43101);
#40203=AXIS2_PLACEMENT_3D('',#53230,#43103,#43104);
#40204=AXIS2_PLACEMENT_3D('',#53231,#43105,#43106);
#40205=AXIS2_PLACEMENT_3D('',#53233,#43107,#43108);
#40206=AXIS2_PLACEMENT_3D('',#53236,#43110,#43111);
#40207=AXIS2_PLACEMENT_3D('',#53237,#43112,#43113);
#40208=AXIS2_PLACEMENT_3D('',#53239,#43114,#43115);
#40209=AXIS2_PLACEMENT_3D('',#53242,#43117,#43118);
#40210=AXIS2_PLACEMENT_3D('',#53243,#43119,#43120);
#40211=AXIS2_PLACEMENT_3D('',#53245,#43121,#43122);
#40212=AXIS2_PLACEMENT_3D('',#53248,#43124,#43125);
#40213=AXIS2_PLACEMENT_3D('',#53249,#43126,#43127);
#40214=AXIS2_PLACEMENT_3D('',#53251,#43128,#43129);
#40215=AXIS2_PLACEMENT_3D('',#53253,#43130,#43131);
#40216=AXIS2_PLACEMENT_3D('',#53254,#43132,#43133);
#40217=AXIS2_PLACEMENT_3D('',#53255,#43134,#43135);
#40218=AXIS2_PLACEMENT_3D('',#53257,#43136,#43137);
#40219=AXIS2_PLACEMENT_3D('',#53259,#43138,#43139);
#40220=AXIS2_PLACEMENT_3D('',#53260,#43140,#43141);
#40221=AXIS2_PLACEMENT_3D('',#53261,#43142,#43143);
#40222=AXIS2_PLACEMENT_3D('',#53263,#43144,#43145);
#40223=AXIS2_PLACEMENT_3D('',#53264,#43146,#43147);
#40224=AXIS2_PLACEMENT_3D('',#53265,#43148,#43149);
#40225=AXIS2_PLACEMENT_3D('',#53267,#43150,#43151);
#40226=AXIS2_PLACEMENT_3D('',#53268,#43152,#43153);
#40227=AXIS2_PLACEMENT_3D('',#53269,#43154,#43155);
#40228=AXIS2_PLACEMENT_3D('',#53271,#43156,#43157);
#40229=AXIS2_PLACEMENT_3D('',#53274,#43159,#43160);
#40230=AXIS2_PLACEMENT_3D('',#53275,#43161,#43162);
#40231=AXIS2_PLACEMENT_3D('',#53277,#43163,#43164);
#40232=AXIS2_PLACEMENT_3D('',#53280,#43166,#43167);
#40233=AXIS2_PLACEMENT_3D('',#53281,#43168,#43169);
#40234=AXIS2_PLACEMENT_3D('',#53283,#43170,#43171);
#40235=AXIS2_PLACEMENT_3D('',#53286,#43173,#43174);
#40236=AXIS2_PLACEMENT_3D('',#53287,#43175,#43176);
#40237=AXIS2_PLACEMENT_3D('',#53289,#43177,#43178);
#40238=AXIS2_PLACEMENT_3D('',#53292,#43180,#43181);
#40239=AXIS2_PLACEMENT_3D('',#53331,#43184,#43185);
#40240=AXIS2_PLACEMENT_3D('',#53340,#43189,#43190);
#40241=AXIS2_PLACEMENT_3D('',#53344,#43192,#43193);
#40242=AXIS2_PLACEMENT_3D('',#53368,#43205,#43206);
#40243=AXIS2_PLACEMENT_3D('',#53372,#43208,#43209);
#40244=AXIS2_PLACEMENT_3D('',#53452,#43250,#43251);
#40245=AXIS2_PLACEMENT_3D('',#53475,#43262,#43263);
#40246=AXIS2_PLACEMENT_3D('',#53479,#43265,#43266);
#40247=AXIS2_PLACEMENT_3D('',#53503,#43278,#43279);
#40248=AXIS2_PLACEMENT_3D('',#53507,#43281,#43282);
#40249=AXIS2_PLACEMENT_3D('',#53541,#43300,#43301);
#40250=AXIS2_PLACEMENT_3D('',#53544,#43304,#43305);
#40251=AXIS2_PLACEMENT_3D('',#53547,#43308,#43309);
#40252=AXIS2_PLACEMENT_3D('',#53556,#43313,#43314);
#40253=AXIS2_PLACEMENT_3D('',#53559,#43316,#43317);
#40254=AXIS2_PLACEMENT_3D('',#53592,#43334,#43335);
#40255=AXIS2_PLACEMENT_3D('',#53599,#43338,#43339);
#40256=AXIS2_PLACEMENT_3D('',#53603,#43341,#43342);
#40257=AXIS2_PLACEMENT_3D('',#53621,#43352,#43353);
#40258=AXIS2_PLACEMENT_3D('',#53624,#43356,#43357);
#40259=AXIS2_PLACEMENT_3D('',#53627,#43360,#43361);
#40260=AXIS2_PLACEMENT_3D('',#53642,#43368,#43369);
#40261=AXIS2_PLACEMENT_3D('',#53646,#43371,#43372);
#40262=AXIS2_PLACEMENT_3D('',#53652,#43376,#43377);
#40263=AXIS2_PLACEMENT_3D('',#53657,#43380,#43381);
#40264=AXIS2_PLACEMENT_3D('',#53662,#43384,#43385);
#40265=AXIS2_PLACEMENT_3D('',#53667,#43388,#43389);
#40266=AXIS2_PLACEMENT_3D('',#53672,#43392,#43393);
#40267=AXIS2_PLACEMENT_3D('',#53677,#43396,#43397);
#40268=AXIS2_PLACEMENT_3D('',#53682,#43400,#43401);
#40269=AXIS2_PLACEMENT_3D('',#53687,#43404,#43405);
#40270=AXIS2_PLACEMENT_3D('',#53692,#43408,#43409);
#40271=AXIS2_PLACEMENT_3D('',#53697,#43412,#43413);
#40272=AXIS2_PLACEMENT_3D('',#53702,#43416,#43417);
#40273=AXIS2_PLACEMENT_3D('',#53707,#43420,#43421);
#40274=AXIS2_PLACEMENT_3D('',#53711,#43423,#43424);
#40275=AXIS2_PLACEMENT_3D('',#53716,#43427,#43428);
#40276=AXIS2_PLACEMENT_3D('',#53721,#43431,#43432);
#40277=AXIS2_PLACEMENT_3D('',#53726,#43435,#43436);
#40278=AXIS2_PLACEMENT_3D('',#53731,#43439,#43440);
#40279=AXIS2_PLACEMENT_3D('',#53736,#43443,#43444);
#40280=AXIS2_PLACEMENT_3D('',#53741,#43447,#43448);
#40281=AXIS2_PLACEMENT_3D('',#53746,#43451,#43452);
#40282=AXIS2_PLACEMENT_3D('',#53751,#43455,#43456);
#40283=AXIS2_PLACEMENT_3D('',#53756,#43459,#43460);
#40284=AXIS2_PLACEMENT_3D('',#53761,#43463,#43464);
#40285=AXIS2_PLACEMENT_3D('',#53766,#43467,#43468);
#40286=AXIS2_PLACEMENT_3D('',#53771,#43471,#43472);
#40287=AXIS2_PLACEMENT_3D('',#53776,#43475,#43476);
#40288=AXIS2_PLACEMENT_3D('',#53781,#43479,#43480);
#40289=AXIS2_PLACEMENT_3D('',#53786,#43483,#43484);
#40290=AXIS2_PLACEMENT_3D('',#53791,#43487,#43488);
#40291=AXIS2_PLACEMENT_3D('',#53796,#43491,#43492);
#40292=AXIS2_PLACEMENT_3D('',#53801,#43495,#43496);
#40293=AXIS2_PLACEMENT_3D('',#53806,#43499,#43500);
#40294=AXIS2_PLACEMENT_3D('',#53811,#43503,#43504);
#40295=AXIS2_PLACEMENT_3D('',#53816,#43507,#43508);
#40296=AXIS2_PLACEMENT_3D('',#53821,#43511,#43512);
#40297=AXIS2_PLACEMENT_3D('',#53826,#43515,#43516);
#40298=AXIS2_PLACEMENT_3D('',#53832,#43520,#43521);
#40299=AXIS2_PLACEMENT_3D('',#53837,#43524,#43525);
#40300=AXIS2_PLACEMENT_3D('',#53842,#43528,#43529);
#40301=AXIS2_PLACEMENT_3D('',#53847,#43532,#43533);
#40302=AXIS2_PLACEMENT_3D('',#53852,#43536,#43537);
#40303=AXIS2_PLACEMENT_3D('',#53857,#43540,#43541);
#40304=AXIS2_PLACEMENT_3D('',#53862,#43544,#43545);
#40305=AXIS2_PLACEMENT_3D('',#53867,#43548,#43549);
#40306=AXIS2_PLACEMENT_3D('',#53872,#43552,#43553);
#40307=AXIS2_PLACEMENT_3D('',#53877,#43556,#43557);
#40308=AXIS2_PLACEMENT_3D('',#53882,#43560,#43561);
#40309=AXIS2_PLACEMENT_3D('',#53887,#43564,#43565);
#40310=AXIS2_PLACEMENT_3D('',#53888,#43566,#43567);
#40311=AXIS2_PLACEMENT_3D('',#53899,#43572,#43573);
#40312=AXIS2_PLACEMENT_3D('',#53903,#43575,#43576);
#40313=AXIS2_PLACEMENT_3D('',#53912,#43581,#43582);
#40314=AXIS2_PLACEMENT_3D('',#53917,#43585,#43586);
#40315=AXIS2_PLACEMENT_3D('',#53922,#43589,#43590);
#40316=AXIS2_PLACEMENT_3D('',#53927,#43593,#43594);
#40317=AXIS2_PLACEMENT_3D('',#53932,#43597,#43598);
#40318=AXIS2_PLACEMENT_3D('',#53937,#43601,#43602);
#40319=AXIS2_PLACEMENT_3D('',#53942,#43605,#43606);
#40320=AXIS2_PLACEMENT_3D('',#53947,#43609,#43610);
#40321=AXIS2_PLACEMENT_3D('',#53952,#43613,#43614);
#40322=AXIS2_PLACEMENT_3D('',#53957,#43617,#43618);
#40323=AXIS2_PLACEMENT_3D('',#53962,#43621,#43622);
#40324=AXIS2_PLACEMENT_3D('',#53967,#43625,#43626);
#40325=AXIS2_PLACEMENT_3D('',#53972,#43629,#43630);
#40326=AXIS2_PLACEMENT_3D('',#53978,#43634,#43635);
#40327=AXIS2_PLACEMENT_3D('',#53983,#43638,#43639);
#40328=AXIS2_PLACEMENT_3D('',#53988,#43642,#43643);
#40329=AXIS2_PLACEMENT_3D('',#53993,#43646,#43647);
#40330=AXIS2_PLACEMENT_3D('',#53998,#43650,#43651);
#40331=AXIS2_PLACEMENT_3D('',#54003,#43654,#43655);
#40332=AXIS2_PLACEMENT_3D('',#54008,#43658,#43659);
#40333=AXIS2_PLACEMENT_3D('',#54013,#43662,#43663);
#40334=AXIS2_PLACEMENT_3D('',#54018,#43666,#43667);
#40335=AXIS2_PLACEMENT_3D('',#54023,#43670,#43671);
#40336=AXIS2_PLACEMENT_3D('',#54028,#43674,#43675);
#40337=AXIS2_PLACEMENT_3D('',#54033,#43678,#43679);
#40338=AXIS2_PLACEMENT_3D('',#54038,#43682,#43683);
#40339=AXIS2_PLACEMENT_3D('',#54043,#43686,#43687);
#40340=AXIS2_PLACEMENT_3D('',#54048,#43690,#43691);
#40341=AXIS2_PLACEMENT_3D('',#54053,#43694,#43695);
#40342=AXIS2_PLACEMENT_3D('',#54058,#43698,#43699);
#40343=AXIS2_PLACEMENT_3D('',#54063,#43702,#43703);
#40344=AXIS2_PLACEMENT_3D('',#54068,#43706,#43707);
#40345=AXIS2_PLACEMENT_3D('',#54073,#43710,#43711);
#40346=AXIS2_PLACEMENT_3D('',#54078,#43714,#43715);
#40347=AXIS2_PLACEMENT_3D('',#54083,#43718,#43719);
#40348=AXIS2_PLACEMENT_3D('',#54088,#43722,#43723);
#40349=AXIS2_PLACEMENT_3D('',#54093,#43726,#43727);
#40350=AXIS2_PLACEMENT_3D('',#54097,#43729,#43730);
#40351=AXIS2_PLACEMENT_3D('',#54102,#43733,#43734);
#40352=AXIS2_PLACEMENT_3D('',#54107,#43737,#43738);
#40353=AXIS2_PLACEMENT_3D('',#54112,#43741,#43742);
#40354=AXIS2_PLACEMENT_3D('',#54117,#43745,#43746);
#40355=AXIS2_PLACEMENT_3D('',#54122,#43749,#43750);
#40356=AXIS2_PLACEMENT_3D('',#54127,#43753,#43754);
#40357=AXIS2_PLACEMENT_3D('',#54132,#43757,#43758);
#40358=AXIS2_PLACEMENT_3D('',#54137,#43761,#43762);
#40359=AXIS2_PLACEMENT_3D('',#54142,#43765,#43766);
#40360=AXIS2_PLACEMENT_3D('',#54147,#43769,#43770);
#40361=AXIS2_PLACEMENT_3D('',#54149,#43772,#43773);
#40362=AXIS2_PLACEMENT_3D('',#54155,#43777,#43778);
#40363=AXIS2_PLACEMENT_3D('',#54161,#43782,#43783);
#40364=AXIS2_PLACEMENT_3D('',#54170,#43788,#43789);
#40365=AXIS2_PLACEMENT_3D('',#54176,#43793,#43794);
#40366=AXIS2_PLACEMENT_3D('',#54185,#43799,#43800);
#40367=AXIS2_PLACEMENT_3D('',#54191,#43804,#43805);
#40368=AXIS2_PLACEMENT_3D('',#54197,#43809,#43810);
#40369=AXIS2_PLACEMENT_3D('',#54206,#43815,#43816);
#40370=AXIS2_PLACEMENT_3D('',#54215,#43821,#43822);
#40371=AXIS2_PLACEMENT_3D('',#54221,#43826,#43827);
#40372=AXIS2_PLACEMENT_3D('',#54230,#43832,#43833);
#40373=AXIS2_PLACEMENT_3D('',#54239,#43838,#43839);
#40374=AXIS2_PLACEMENT_3D('',#54245,#43843,#43844);
#40375=AXIS2_PLACEMENT_3D('',#54251,#43848,#43849);
#40376=AXIS2_PLACEMENT_3D('',#54260,#43854,#43855);
#40377=AXIS2_PLACEMENT_3D('',#54266,#43859,#43860);
#40378=AXIS2_PLACEMENT_3D('',#54275,#43865,#43866);
#40379=AXIS2_PLACEMENT_3D('',#54281,#43870,#43871);
#40380=AXIS2_PLACEMENT_3D('',#54287,#43875,#43876);
#40381=AXIS2_PLACEMENT_3D('',#54296,#43881,#43882);
#40382=AXIS2_PLACEMENT_3D('',#54305,#43887,#43888);
#40383=AXIS2_PLACEMENT_3D('',#54311,#43892,#43893);
#40384=AXIS2_PLACEMENT_3D('',#54320,#43898,#43899);
#40385=AXIS2_PLACEMENT_3D('',#54387,#43906,#43907);
#40386=AXIS2_PLACEMENT_3D('',#54388,#43908,#43909);
#40387=AXIS2_PLACEMENT_3D('',#54390,#43910,#43911);
#40388=AXIS2_PLACEMENT_3D('',#54396,#43912,#43913);
#40389=AXIS2_PLACEMENT_3D('',#54404,#43914,#43915);
#40390=AXIS2_PLACEMENT_3D('',#54408,#43917,#43918);
#40391=AXIS2_PLACEMENT_3D('',#54417,#43919,#43920);
#40392=AXIS2_PLACEMENT_3D('',#54428,#43923,#43924);
#40393=AXIS2_PLACEMENT_3D('',#54438,#43926,#43927);
#40394=AXIS2_PLACEMENT_3D('',#54448,#43928,#43929);
#40395=AXIS2_PLACEMENT_3D('',#54459,#43931,#43932);
#40396=AXIS2_PLACEMENT_3D('',#54463,#43934,#43935);
#40397=AXIS2_PLACEMENT_3D('',#54473,#43936,#43937);
#40398=AXIS2_PLACEMENT_3D('',#54477,#43939,#43940);
#40399=AXIS2_PLACEMENT_3D('',#54487,#43941,#43942);
#40400=AXIS2_PLACEMENT_3D('',#54491,#43944,#43945);
#40401=AXIS2_PLACEMENT_3D('',#54502,#43947,#43948);
#40402=AXIS2_PLACEMENT_3D('',#54511,#43949,#43950);
#40403=AXIS2_PLACEMENT_3D('',#54515,#43952,#43953);
#40404=AXIS2_PLACEMENT_3D('',#54528,#43955,#43956);
#40405=AXIS2_PLACEMENT_3D('',#54537,#43957,#43958);
#40406=AXIS2_PLACEMENT_3D('',#54548,#43960,#43961);
#40407=AXIS2_PLACEMENT_3D('',#54550,#43962,#43963);
#40408=AXIS2_PLACEMENT_3D('',#54560,#43964,#43965);
#40409=AXIS2_PLACEMENT_3D('',#54570,#43966,#43967);
#40410=AXIS2_PLACEMENT_3D('',#54580,#43968,#43969);
#40411=AXIS2_PLACEMENT_3D('',#54582,#43970,#43971);
#40412=AXIS2_PLACEMENT_3D('',#54592,#43972,#43973);
#40413=AXIS2_PLACEMENT_3D('',#54594,#43974,#43975);
#40414=AXIS2_PLACEMENT_3D('',#54603,#43976,#43977);
#40415=AXIS2_PLACEMENT_3D('',#54605,#43978,#43979);
#40416=AXIS2_PLACEMENT_3D('',#54616,#43980,#43981);
#40417=AXIS2_PLACEMENT_3D('',#54626,#43982,#43983);
#40418=AXIS2_PLACEMENT_3D('',#54628,#43984,#43985);
#40419=AXIS2_PLACEMENT_3D('',#54638,#43986,#43987);
#40420=AXIS2_PLACEMENT_3D('',#54648,#43988,#43989);
#40421=AXIS2_PLACEMENT_3D('',#54658,#43990,#43991);
#40422=AXIS2_PLACEMENT_3D('',#54660,#43992,#43993);
#40423=AXIS2_PLACEMENT_3D('',#54669,#43994,#43995);
#40424=AXIS2_PLACEMENT_3D('',#54670,#43996,#43997);
#40425=AXIS2_PLACEMENT_3D('',#54680,#43998,#43999);
#40426=AXIS2_PLACEMENT_3D('',#54682,#44000,#44001);
#40427=AXIS2_PLACEMENT_3D('',#54697,#44002,#44003);
#40428=AXIS2_PLACEMENT_3D('',#54699,#44004,#44005);
#40429=AXIS2_PLACEMENT_3D('',#54710,#44006,#44007);
#40430=AXIS2_PLACEMENT_3D('',#54712,#44008,#44009);
#40431=AXIS2_PLACEMENT_3D('',#54727,#44010,#44011);
#40432=AXIS2_PLACEMENT_3D('',#54737,#44012,#44013);
#40433=AXIS2_PLACEMENT_3D('',#54739,#44014,#44015);
#40434=AXIS2_PLACEMENT_3D('',#54754,#44016,#44017);
#40435=AXIS2_PLACEMENT_3D('',#54764,#44018,#44019);
#40436=AXIS2_PLACEMENT_3D('',#54779,#44020,#44021);
#40437=AXIS2_PLACEMENT_3D('',#54780,#44022,#44023);
#40438=AXIS2_PLACEMENT_3D('',#54782,#44024,#44025);
#40439=AXIS2_PLACEMENT_3D('',#54789,#44026,#44027);
#40440=AXIS2_PLACEMENT_3D('',#54822,#44028,#44029);
#40441=AXIS2_PLACEMENT_3D('',#54949,#44035,#44036);
#40442=AXIS2_PLACEMENT_3D('',#54960,#44041,#44042);
#40443=AXIS2_PLACEMENT_3D('',#54964,#44044,#44045);
#40444=AXIS2_PLACEMENT_3D('',#54980,#44053,#44054);
#40445=AXIS2_PLACEMENT_3D('',#54984,#44056,#44057);
#40446=AXIS2_PLACEMENT_3D('',#54988,#44059,#44060);
#40447=AXIS2_PLACEMENT_3D('',#54992,#44062,#44063);
#40448=AXIS2_PLACEMENT_3D('',#54996,#44065,#44066);
#40449=AXIS2_PLACEMENT_3D('',#55000,#44068,#44069);
#40450=AXIS2_PLACEMENT_3D('',#55002,#44071,#44072);
#40451=AXIS2_PLACEMENT_3D('',#55017,#44079,#44080);
#40452=AXIS2_PLACEMENT_3D('',#55021,#44082,#44083);
#40453=AXIS2_PLACEMENT_3D('',#55035,#44090,#44091);
#40454=AXIS2_PLACEMENT_3D('',#55039,#44093,#44094);
#40455=AXIS2_PLACEMENT_3D('',#55043,#44096,#44097);
#40456=AXIS2_PLACEMENT_3D('',#55047,#44099,#44100);
#40457=AXIS2_PLACEMENT_3D('',#55051,#44102,#44103);
#40458=AXIS2_PLACEMENT_3D('',#55054,#44105,#44106);
#40459=AXIS2_PLACEMENT_3D('',#55055,#44107,#44108);
#40460=AXIS2_PLACEMENT_3D('',#55060,#44112,#44113);
#40461=AXIS2_PLACEMENT_3D('',#55061,#44114,#44115);
#40462=AXIS2_PLACEMENT_3D('',#55066,#44119,#44120);
#40463=AXIS2_PLACEMENT_3D('',#55067,#44121,#44122);
#40464=AXIS2_PLACEMENT_3D('',#55072,#44126,#44127);
#40465=AXIS2_PLACEMENT_3D('',#55073,#44128,#44129);
#40466=AXIS2_PLACEMENT_3D('',#55078,#44133,#44134);
#40467=AXIS2_PLACEMENT_3D('',#55291,#44139,#44140);
#40468=AXIS2_PLACEMENT_3D('',#55292,#44141,#44142);
#40469=AXIS2_PLACEMENT_3D('',#55293,#44143,#44144);
#40470=AXIS2_PLACEMENT_3D('',#55296,#44147,#44148);
#40471=AXIS2_PLACEMENT_3D('',#55298,#44150,#44151);
#40472=AXIS2_PLACEMENT_3D('',#55301,#44154,#44155);
#40473=AXIS2_PLACEMENT_3D('',#55304,#44158,#44159);
#40474=AXIS2_PLACEMENT_3D('',#55306,#44161,#44162);
#40475=AXIS2_PLACEMENT_3D('',#55307,#44163,#44164);
#40476=AXIS2_PLACEMENT_3D('',#55520,#44169,#44170);
#40477=AXIS2_PLACEMENT_3D('',#55521,#44171,#44172);
#40478=AXIS2_PLACEMENT_3D('',#55522,#44173,#44174);
#40479=AXIS2_PLACEMENT_3D('',#55525,#44177,#44178);
#40480=AXIS2_PLACEMENT_3D('',#55527,#44180,#44181);
#40481=AXIS2_PLACEMENT_3D('',#55530,#44184,#44185);
#40482=AXIS2_PLACEMENT_3D('',#55533,#44188,#44189);
#40483=AXIS2_PLACEMENT_3D('',#55535,#44191,#44192);
#40484=AXIS2_PLACEMENT_3D('',#55536,#44193,#44194);
#40485=AXIS2_PLACEMENT_3D('',#55537,#44195,#44196);
#40486=AXIS2_PLACEMENT_3D('',#55538,#44197,#44198);
#40487=AXIS2_PLACEMENT_3D('',#55539,#44199,#44200);
#40488=AXIS2_PLACEMENT_3D('',#55540,#44201,#44202);
#40489=AXIS2_PLACEMENT_3D('',#55541,#44203,#44204);
#40490=AXIS2_PLACEMENT_3D('',#55542,#44205,#44206);
#40491=AXIS2_PLACEMENT_3D('',#55543,#44207,#44208);
#40492=AXIS2_PLACEMENT_3D('',#55545,#44209,#44210);
#40493=AXIS2_PLACEMENT_3D('',#55548,#44212,#44213);
#40494=AXIS2_PLACEMENT_3D('',#55549,#44214,#44215);
#40495=AXIS2_PLACEMENT_3D('',#55551,#44216,#44217);
#40496=AXIS2_PLACEMENT_3D('',#55554,#44219,#44220);
#40497=AXIS2_PLACEMENT_3D('',#55555,#44221,#44222);
#40498=AXIS2_PLACEMENT_3D('',#55557,#44223,#44224);
#40499=AXIS2_PLACEMENT_3D('',#55561,#44226,#44227);
#40500=AXIS2_PLACEMENT_3D('',#55565,#44229,#44230);
#40501=AXIS2_PLACEMENT_3D('',#55568,#44232,#44233);
#40502=AXIS2_PLACEMENT_3D('',#55572,#44235,#44236);
#40503=AXIS2_PLACEMENT_3D('',#55576,#44238,#44239);
#40504=AXIS2_PLACEMENT_3D('',#55578,#44241,#44242);
#40505=AXIS2_PLACEMENT_3D('',#55580,#44243,#44244);
#40506=AXIS2_PLACEMENT_3D('',#55584,#44246,#44247);
#40507=AXIS2_PLACEMENT_3D('',#55588,#44249,#44250);
#40508=AXIS2_PLACEMENT_3D('',#55591,#44252,#44253);
#40509=AXIS2_PLACEMENT_3D('',#55595,#44255,#44256);
#40510=AXIS2_PLACEMENT_3D('',#55599,#44258,#44259);
#40511=AXIS2_PLACEMENT_3D('',#55601,#44261,#44262);
#40512=AXIS2_PLACEMENT_3D('',#55604,#44265,#44266);
#40513=AXIS2_PLACEMENT_3D('',#55607,#44269,#44270);
#40514=AXIS2_PLACEMENT_3D('',#55608,#44271,#44272);
#40515=AXIS2_PLACEMENT_3D('',#55609,#44273,#44274);
#40516=AXIS2_PLACEMENT_3D('',#55610,#44275,#44276);
#40517=AXIS2_PLACEMENT_3D('',#55613,#44279,#44280);
#40518=AXIS2_PLACEMENT_3D('',#55616,#44283,#44284);
#40519=AXIS2_PLACEMENT_3D('',#55618,#44286,#44287);
#40520=AXIS2_PLACEMENT_3D('',#55620,#44289,#44290);
#40521=AXIS2_PLACEMENT_3D('',#55621,#44291,#44292);
#40522=AXIS2_PLACEMENT_3D('',#55622,#44293,#44294);
#40523=AXIS2_PLACEMENT_3D('',#55623,#44295,#44296);
#40524=AXIS2_PLACEMENT_3D('',#55624,#44297,#44298);
#40525=AXIS2_PLACEMENT_3D('',#55625,#44299,#44300);
#40526=AXIS2_PLACEMENT_3D('',#55626,#44301,#44302);
#40527=AXIS2_PLACEMENT_3D('',#55627,#44303,#44304);
#40528=AXIS2_PLACEMENT_3D('',#55628,#44305,#44306);
#40529=AXIS2_PLACEMENT_3D('',#55629,#44307,#44308);
#40530=AXIS2_PLACEMENT_3D('',#55631,#44309,#44310);
#40531=AXIS2_PLACEMENT_3D('',#55634,#44312,#44313);
#40532=AXIS2_PLACEMENT_3D('',#55635,#44314,#44315);
#40533=AXIS2_PLACEMENT_3D('',#55637,#44316,#44317);
#40534=AXIS2_PLACEMENT_3D('',#55640,#44319,#44320);
#40535=AXIS2_PLACEMENT_3D('',#55641,#44321,#44322);
#40536=AXIS2_PLACEMENT_3D('',#55643,#44323,#44324);
#40537=AXIS2_PLACEMENT_3D('',#55647,#44326,#44327);
#40538=AXIS2_PLACEMENT_3D('',#55651,#44329,#44330);
#40539=AXIS2_PLACEMENT_3D('',#55654,#44332,#44333);
#40540=AXIS2_PLACEMENT_3D('',#55658,#44335,#44336);
#40541=AXIS2_PLACEMENT_3D('',#55662,#44338,#44339);
#40542=AXIS2_PLACEMENT_3D('',#55664,#44341,#44342);
#40543=AXIS2_PLACEMENT_3D('',#55666,#44343,#44344);
#40544=AXIS2_PLACEMENT_3D('',#55670,#44346,#44347);
#40545=AXIS2_PLACEMENT_3D('',#55674,#44349,#44350);
#40546=AXIS2_PLACEMENT_3D('',#55677,#44352,#44353);
#40547=AXIS2_PLACEMENT_3D('',#55681,#44355,#44356);
#40548=AXIS2_PLACEMENT_3D('',#55685,#44358,#44359);
#40549=AXIS2_PLACEMENT_3D('',#55687,#44361,#44362);
#40550=AXIS2_PLACEMENT_3D('',#55690,#44365,#44366);
#40551=AXIS2_PLACEMENT_3D('',#55693,#44369,#44370);
#40552=AXIS2_PLACEMENT_3D('',#55694,#44371,#44372);
#40553=AXIS2_PLACEMENT_3D('',#55695,#44373,#44374);
#40554=AXIS2_PLACEMENT_3D('',#55696,#44375,#44376);
#40555=AXIS2_PLACEMENT_3D('',#55699,#44379,#44380);
#40556=AXIS2_PLACEMENT_3D('',#55702,#44383,#44384);
#40557=AXIS2_PLACEMENT_3D('',#55704,#44386,#44387);
#40558=AXIS2_PLACEMENT_3D('',#55706,#44389,#44390);
#40559=AXIS2_PLACEMENT_3D('',#55707,#44391,#44392);
#40560=AXIS2_PLACEMENT_3D('',#55708,#44393,#44394);
#40561=AXIS2_PLACEMENT_3D('',#55709,#44395,#44396);
#40562=AXIS2_PLACEMENT_3D('',#55710,#44397,#44398);
#40563=AXIS2_PLACEMENT_3D('',#55711,#44399,#44400);
#40564=AXIS2_PLACEMENT_3D('',#55712,#44401,#44402);
#40565=AXIS2_PLACEMENT_3D('',#55713,#44403,#44404);
#40566=AXIS2_PLACEMENT_3D('',#55714,#44405,#44406);
#40567=AXIS2_PLACEMENT_3D('',#55715,#44407,#44408);
#40568=AXIS2_PLACEMENT_3D('',#55717,#44409,#44410);
#40569=AXIS2_PLACEMENT_3D('',#55720,#44412,#44413);
#40570=AXIS2_PLACEMENT_3D('',#55721,#44414,#44415);
#40571=AXIS2_PLACEMENT_3D('',#55723,#44416,#44417);
#40572=AXIS2_PLACEMENT_3D('',#55726,#44419,#44420);
#40573=AXIS2_PLACEMENT_3D('',#55727,#44421,#44422);
#40574=AXIS2_PLACEMENT_3D('',#55729,#44423,#44424);
#40575=AXIS2_PLACEMENT_3D('',#55733,#44426,#44427);
#40576=AXIS2_PLACEMENT_3D('',#55737,#44429,#44430);
#40577=AXIS2_PLACEMENT_3D('',#55740,#44432,#44433);
#40578=AXIS2_PLACEMENT_3D('',#55744,#44435,#44436);
#40579=AXIS2_PLACEMENT_3D('',#55748,#44438,#44439);
#40580=AXIS2_PLACEMENT_3D('',#55750,#44441,#44442);
#40581=AXIS2_PLACEMENT_3D('',#55752,#44443,#44444);
#40582=AXIS2_PLACEMENT_3D('',#55756,#44446,#44447);
#40583=AXIS2_PLACEMENT_3D('',#55760,#44449,#44450);
#40584=AXIS2_PLACEMENT_3D('',#55763,#44452,#44453);
#40585=AXIS2_PLACEMENT_3D('',#55767,#44455,#44456);
#40586=AXIS2_PLACEMENT_3D('',#55771,#44458,#44459);
#40587=AXIS2_PLACEMENT_3D('',#55773,#44461,#44462);
#40588=AXIS2_PLACEMENT_3D('',#55776,#44465,#44466);
#40589=AXIS2_PLACEMENT_3D('',#55779,#44469,#44470);
#40590=AXIS2_PLACEMENT_3D('',#55780,#44471,#44472);
#40591=AXIS2_PLACEMENT_3D('',#55781,#44473,#44474);
#40592=AXIS2_PLACEMENT_3D('',#55782,#44475,#44476);
#40593=AXIS2_PLACEMENT_3D('',#55785,#44479,#44480);
#40594=AXIS2_PLACEMENT_3D('',#55788,#44483,#44484);
#40595=AXIS2_PLACEMENT_3D('',#55790,#44486,#44487);
#40596=AXIS2_PLACEMENT_3D('',#55792,#44489,#44490);
#40597=AXIS2_PLACEMENT_3D('',#55793,#44491,#44492);
#40598=AXIS2_PLACEMENT_3D('',#55794,#44493,#44494);
#40599=AXIS2_PLACEMENT_3D('',#55795,#44495,#44496);
#40600=AXIS2_PLACEMENT_3D('',#55796,#44497,#44498);
#40601=AXIS2_PLACEMENT_3D('',#55797,#44499,#44500);
#40602=AXIS2_PLACEMENT_3D('',#55798,#44501,#44502);
#40603=AXIS2_PLACEMENT_3D('',#55799,#44503,#44504);
#40604=AXIS2_PLACEMENT_3D('',#55800,#44505,#44506);
#40605=AXIS2_PLACEMENT_3D('',#55801,#44507,#44508);
#40606=AXIS2_PLACEMENT_3D('',#55803,#44509,#44510);
#40607=AXIS2_PLACEMENT_3D('',#55806,#44512,#44513);
#40608=AXIS2_PLACEMENT_3D('',#55807,#44514,#44515);
#40609=AXIS2_PLACEMENT_3D('',#55809,#44516,#44517);
#40610=AXIS2_PLACEMENT_3D('',#55812,#44519,#44520);
#40611=AXIS2_PLACEMENT_3D('',#55813,#44521,#44522);
#40612=AXIS2_PLACEMENT_3D('',#55815,#44523,#44524);
#40613=AXIS2_PLACEMENT_3D('',#55819,#44526,#44527);
#40614=AXIS2_PLACEMENT_3D('',#55823,#44529,#44530);
#40615=AXIS2_PLACEMENT_3D('',#55826,#44532,#44533);
#40616=AXIS2_PLACEMENT_3D('',#55830,#44535,#44536);
#40617=AXIS2_PLACEMENT_3D('',#55834,#44538,#44539);
#40618=AXIS2_PLACEMENT_3D('',#55836,#44541,#44542);
#40619=AXIS2_PLACEMENT_3D('',#55838,#44543,#44544);
#40620=AXIS2_PLACEMENT_3D('',#55842,#44546,#44547);
#40621=AXIS2_PLACEMENT_3D('',#55846,#44549,#44550);
#40622=AXIS2_PLACEMENT_3D('',#55849,#44552,#44553);
#40623=AXIS2_PLACEMENT_3D('',#55853,#44555,#44556);
#40624=AXIS2_PLACEMENT_3D('',#55857,#44558,#44559);
#40625=AXIS2_PLACEMENT_3D('',#55859,#44561,#44562);
#40626=AXIS2_PLACEMENT_3D('',#55862,#44565,#44566);
#40627=AXIS2_PLACEMENT_3D('',#55865,#44569,#44570);
#40628=AXIS2_PLACEMENT_3D('',#55866,#44571,#44572);
#40629=AXIS2_PLACEMENT_3D('',#55867,#44573,#44574);
#40630=AXIS2_PLACEMENT_3D('',#55868,#44575,#44576);
#40631=AXIS2_PLACEMENT_3D('',#55871,#44579,#44580);
#40632=AXIS2_PLACEMENT_3D('',#55874,#44583,#44584);
#40633=AXIS2_PLACEMENT_3D('',#55876,#44586,#44587);
#40634=AXIS2_PLACEMENT_3D('',#55878,#44589,#44590);
#40635=AXIS2_PLACEMENT_3D('',#55879,#44591,#44592);
#40636=AXIS2_PLACEMENT_3D('',#55880,#44593,#44594);
#40637=AXIS2_PLACEMENT_3D('',#55881,#44595,#44596);
#40638=AXIS2_PLACEMENT_3D('',#55887,#44597,#44598);
#40639=AXIS2_PLACEMENT_3D('',#55897,#44599,#44600);
#40640=AXIS2_PLACEMENT_3D('',#55900,#44602,#44603);
#40641=AXIS2_PLACEMENT_3D('',#55912,#44604,#44605);
#40642=AXIS2_PLACEMENT_3D('',#55922,#44607,#44608);
#40643=AXIS2_PLACEMENT_3D('',#55925,#44610,#44611);
#40644=AXIS2_PLACEMENT_3D('',#55937,#44612,#44613);
#40645=AXIS2_PLACEMENT_3D('',#55941,#44615,#44616);
#40646=AXIS2_PLACEMENT_3D('',#55950,#44618,#44619);
#40647=AXIS2_PLACEMENT_3D('',#55960,#44620,#44621);
#40648=AXIS2_PLACEMENT_3D('',#55964,#44623,#44624);
#40649=AXIS2_PLACEMENT_3D('',#55974,#44625,#44626);
#40650=AXIS2_PLACEMENT_3D('',#55986,#44628,#44629);
#40651=AXIS2_PLACEMENT_3D('',#55990,#44631,#44632);
#40652=AXIS2_PLACEMENT_3D('',#55999,#44633,#44634);
#40653=AXIS2_PLACEMENT_3D('',#56013,#44637,#44638);
#40654=AXIS2_PLACEMENT_3D('',#56022,#44639,#44640);
#40655=AXIS2_PLACEMENT_3D('',#56025,#44642,#44643);
#40656=AXIS2_PLACEMENT_3D('',#56032,#44644,#44645);
#40657=AXIS2_PLACEMENT_3D('',#56039,#44646,#44647);
#40658=AXIS2_PLACEMENT_3D('',#56040,#44648,#44649);
#40659=AXIS2_PLACEMENT_3D('',#56051,#44650,#44651);
#40660=AXIS2_PLACEMENT_3D('',#56061,#44652,#44653);
#40661=AXIS2_PLACEMENT_3D('',#56062,#44654,#44655);
#40662=AXIS2_PLACEMENT_3D('',#56073,#44656,#44657);
#40663=AXIS2_PLACEMENT_3D('',#56075,#44658,#44659);
#40664=AXIS2_PLACEMENT_3D('',#56084,#44660,#44661);
#40665=AXIS2_PLACEMENT_3D('',#56095,#44662,#44663);
#40666=AXIS2_PLACEMENT_3D('',#56097,#44664,#44665);
#40667=AXIS2_PLACEMENT_3D('',#56106,#44666,#44667);
#40668=AXIS2_PLACEMENT_3D('',#56116,#44668,#44669);
#40669=AXIS2_PLACEMENT_3D('',#56118,#44670,#44671);
#40670=AXIS2_PLACEMENT_3D('',#56128,#44672,#44673);
#40671=AXIS2_PLACEMENT_3D('',#56139,#44674,#44675);
#40672=AXIS2_PLACEMENT_3D('',#56149,#44676,#44677);
#40673=AXIS2_PLACEMENT_3D('',#56150,#44678,#44679);
#40674=AXIS2_PLACEMENT_3D('',#56151,#44680,#44681);
#40675=AXIS2_PLACEMENT_3D('',#56159,#44682,#44683);
#40676=AXIS2_PLACEMENT_3D('',#56160,#44684,#44685);
#40677=AXIS2_PLACEMENT_3D('',#56161,#44686,#44687);
#40678=AXIS2_PLACEMENT_3D('',#56171,#44688,#44689);
#40679=AXIS2_PLACEMENT_3D('',#56172,#44690,#44691);
#40680=AXIS2_PLACEMENT_3D('',#56188,#44692,#44693);
#40681=AXIS2_PLACEMENT_3D('',#56190,#44694,#44695);
#40682=AXIS2_PLACEMENT_3D('',#56199,#44696,#44697);
#40683=AXIS2_PLACEMENT_3D('',#56200,#44698,#44699);
#40684=AXIS2_PLACEMENT_3D('',#56202,#44700,#44701);
#40685=AXIS2_PLACEMENT_3D('',#56213,#44702,#44703);
#40686=AXIS2_PLACEMENT_3D('',#56214,#44704,#44705);
#40687=AXIS2_PLACEMENT_3D('',#56216,#44706,#44707);
#40688=AXIS2_PLACEMENT_3D('',#56226,#44708,#44709);
#40689=AXIS2_PLACEMENT_3D('',#56228,#44710,#44711);
#40690=AXIS2_PLACEMENT_3D('',#56238,#44712,#44713);
#40691=AXIS2_PLACEMENT_3D('',#56239,#44714,#44715);
#40692=AXIS2_PLACEMENT_3D('',#56268,#44718,#44719);
#40693=AXIS2_PLACEMENT_3D('',#56270,#44721,#44722);
#40694=AXIS2_PLACEMENT_3D('',#56273,#44725,#44726);
#40695=AXIS2_PLACEMENT_3D('',#56275,#44728,#44729);
#40696=AXIS2_PLACEMENT_3D('',#56278,#44732,#44733);
#40697=AXIS2_PLACEMENT_3D('',#56280,#44735,#44736);
#40698=AXIS2_PLACEMENT_3D('',#56282,#44738,#44739);
#40699=AXIS2_PLACEMENT_3D('',#56285,#44742,#44743);
#40700=AXIS2_PLACEMENT_3D('',#56288,#44746,#44747);
#40701=AXIS2_PLACEMENT_3D('',#56290,#44749,#44750);
#40702=AXIS2_PLACEMENT_3D('',#56293,#44753,#44754);
#40703=AXIS2_PLACEMENT_3D('',#56773,#44798,#44799);
#40704=AXIS2_PLACEMENT_3D('',#56774,#44800,#44801);
#40705=AXIS2_PLACEMENT_3D('',#56775,#44802,#44803);
#40706=AXIS2_PLACEMENT_3D('',#56776,#44804,#44805);
#40707=AXIS2_PLACEMENT_3D('',#56777,#44806,#44807);
#40708=AXIS2_PLACEMENT_3D('',#56778,#44808,#44809);
#40709=AXIS2_PLACEMENT_3D('',#56779,#44810,#44811);
#40710=AXIS2_PLACEMENT_3D('',#56780,#44812,#44813);
#40711=AXIS2_PLACEMENT_3D('',#56781,#44814,#44815);
#40712=AXIS2_PLACEMENT_3D('',#56782,#44816,#44817);
#40713=AXIS2_PLACEMENT_3D('',#56783,#44818,#44819);
#40714=AXIS2_PLACEMENT_3D('',#56784,#44820,#44821);
#40715=AXIS2_PLACEMENT_3D('',#56785,#44822,#44823);
#40716=AXIS2_PLACEMENT_3D('',#56786,#44824,#44825);
#40717=AXIS2_PLACEMENT_3D('',#56787,#44826,#44827);
#40718=AXIS2_PLACEMENT_3D('',#56788,#44828,#44829);
#40719=AXIS2_PLACEMENT_3D('',#56789,#44830,#44831);
#40720=AXIS2_PLACEMENT_3D('',#56790,#44832,#44833);
#40721=AXIS2_PLACEMENT_3D('',#56791,#44834,#44835);
#40722=AXIS2_PLACEMENT_3D('',#56792,#44836,#44837);
#40723=AXIS2_PLACEMENT_3D('',#56793,#44838,#44839);
#40724=AXIS2_PLACEMENT_3D('',#56794,#44840,#44841);
#40725=AXIS2_PLACEMENT_3D('',#56795,#44842,#44843);
#40726=AXIS2_PLACEMENT_3D('',#56796,#44844,#44845);
#40727=AXIS2_PLACEMENT_3D('',#56797,#44846,#44847);
#40728=AXIS2_PLACEMENT_3D('',#56798,#44848,#44849);
#40729=AXIS2_PLACEMENT_3D('',#56799,#44850,#44851);
#40730=AXIS2_PLACEMENT_3D('',#56800,#44852,#44853);
#40731=AXIS2_PLACEMENT_3D('',#56801,#44854,#44855);
#40732=AXIS2_PLACEMENT_3D('',#56802,#44856,#44857);
#40733=AXIS2_PLACEMENT_3D('',#56803,#44858,#44859);
#40734=AXIS2_PLACEMENT_3D('',#56804,#44860,#44861);
#40735=AXIS2_PLACEMENT_3D('',#56805,#44862,#44863);
#40736=AXIS2_PLACEMENT_3D('',#56806,#44864,#44865);
#40737=AXIS2_PLACEMENT_3D('',#56807,#44866,#44867);
#40738=AXIS2_PLACEMENT_3D('',#56808,#44868,#44869);
#40739=AXIS2_PLACEMENT_3D('',#56809,#44870,#44871);
#40740=AXIS2_PLACEMENT_3D('',#56810,#44872,#44873);
#40741=AXIS2_PLACEMENT_3D('',#56811,#44874,#44875);
#40742=AXIS2_PLACEMENT_3D('',#56812,#44876,#44877);
#40743=AXIS2_PLACEMENT_3D('',#56813,#44878,#44879);
#40744=AXIS2_PLACEMENT_3D('',#56814,#44880,#44881);
#40745=AXIS2_PLACEMENT_3D('',#56815,#44882,#44883);
#40746=AXIS2_PLACEMENT_3D('',#56816,#44884,#44885);
#40747=AXIS2_PLACEMENT_3D('',#56817,#44886,#44887);
#40748=AXIS2_PLACEMENT_3D('',#56818,#44888,#44889);
#40749=AXIS2_PLACEMENT_3D('',#56819,#44890,#44891);
#40750=AXIS2_PLACEMENT_3D('',#56820,#44892,#44893);
#40751=AXIS2_PLACEMENT_3D('',#56821,#44894,#44895);
#40752=AXIS2_PLACEMENT_3D('',#56822,#44896,#44897);
#40753=AXIS2_PLACEMENT_3D('',#56823,#44898,#44899);
#40754=AXIS2_PLACEMENT_3D('',#56824,#44900,#44901);
#40755=AXIS2_PLACEMENT_3D('',#56825,#44902,#44903);
#40756=AXIS2_PLACEMENT_3D('',#56826,#44904,#44905);
#40757=AXIS2_PLACEMENT_3D('',#56827,#44906,#44907);
#40758=AXIS2_PLACEMENT_3D('',#56830,#44910,#44911);
#40759=AXIS2_PLACEMENT_3D('',#56832,#44913,#44914);
#40760=AXIS2_PLACEMENT_3D('',#56834,#44916,#44917);
#40761=AXIS2_PLACEMENT_3D('',#56836,#44919,#44920);
#40762=AXIS2_PLACEMENT_3D('',#56838,#44922,#44923);
#40763=AXIS2_PLACEMENT_3D('',#56840,#44925,#44926);
#40764=AXIS2_PLACEMENT_3D('',#56842,#44928,#44929);
#40765=AXIS2_PLACEMENT_3D('',#56844,#44931,#44932);
#40766=AXIS2_PLACEMENT_3D('',#56846,#44934,#44935);
#40767=AXIS2_PLACEMENT_3D('',#56848,#44937,#44938);
#40768=AXIS2_PLACEMENT_3D('',#56850,#44940,#44941);
#40769=AXIS2_PLACEMENT_3D('',#56851,#44942,#44943);
#40770=AXIS2_PLACEMENT_3D('',#56854,#44946,#44947);
#40771=AXIS2_PLACEMENT_3D('',#56856,#44949,#44950);
#40772=AXIS2_PLACEMENT_3D('',#56858,#44952,#44953);
#40773=AXIS2_PLACEMENT_3D('',#56859,#44954,#44955);
#40774=AXIS2_PLACEMENT_3D('',#56860,#44956,#44957);
#40775=AXIS2_PLACEMENT_3D('',#56861,#44958,#44959);
#40776=AXIS2_PLACEMENT_3D('',#56862,#44960,#44961);
#40777=AXIS2_PLACEMENT_3D('',#56863,#44962,#44963);
#40778=AXIS2_PLACEMENT_3D('',#56865,#44965,#44966);
#40779=AXIS2_PLACEMENT_3D('',#56867,#44968,#44969);
#40780=AXIS2_PLACEMENT_3D('',#56868,#44970,#44971);
#40781=AXIS2_PLACEMENT_3D('',#56870,#44973,#44974);
#40782=AXIS2_PLACEMENT_3D('',#56872,#44976,#44977);
#40783=AXIS2_PLACEMENT_3D('',#56873,#44978,#44979);
#40784=AXIS2_PLACEMENT_3D('',#56875,#44981,#44982);
#40785=AXIS2_PLACEMENT_3D('',#56877,#44984,#44985);
#40786=AXIS2_PLACEMENT_3D('',#56878,#44986,#44987);
#40787=AXIS2_PLACEMENT_3D('',#56880,#44989,#44990);
#40788=AXIS2_PLACEMENT_3D('',#56882,#44992,#44993);
#40789=AXIS2_PLACEMENT_3D('',#56883,#44994,#44995);
#40790=AXIS2_PLACEMENT_3D('',#56885,#44997,#44998);
#40791=AXIS2_PLACEMENT_3D('',#56887,#45000,#45001);
#40792=AXIS2_PLACEMENT_3D('',#56888,#45002,#45003);
#40793=AXIS2_PLACEMENT_3D('',#56890,#45005,#45006);
#40794=AXIS2_PLACEMENT_3D('',#56892,#45008,#45009);
#40795=AXIS2_PLACEMENT_3D('',#56893,#45010,#45011);
#40796=AXIS2_PLACEMENT_3D('',#56895,#45013,#45014);
#40797=AXIS2_PLACEMENT_3D('',#56897,#45016,#45017);
#40798=AXIS2_PLACEMENT_3D('',#56898,#45018,#45019);
#40799=AXIS2_PLACEMENT_3D('',#56900,#45021,#45022);
#40800=AXIS2_PLACEMENT_3D('',#56902,#45024,#45025);
#40801=AXIS2_PLACEMENT_3D('',#56903,#45026,#45027);
#40802=AXIS2_PLACEMENT_3D('',#56905,#45029,#45030);
#40803=AXIS2_PLACEMENT_3D('',#56907,#45032,#45033);
#40804=AXIS2_PLACEMENT_3D('',#56908,#45034,#45035);
#40805=AXIS2_PLACEMENT_3D('',#56910,#45037,#45038);
#40806=AXIS2_PLACEMENT_3D('',#56912,#45040,#45041);
#40807=AXIS2_PLACEMENT_3D('',#56913,#45042,#45043);
#40808=AXIS2_PLACEMENT_3D('',#56915,#45045,#45046);
#40809=AXIS2_PLACEMENT_3D('',#56917,#45048,#45049);
#40810=AXIS2_PLACEMENT_3D('',#56918,#45050,#45051);
#40811=AXIS2_PLACEMENT_3D('',#56920,#45053,#45054);
#40812=AXIS2_PLACEMENT_3D('',#56922,#45056,#45057);
#40813=AXIS2_PLACEMENT_3D('',#56923,#45058,#45059);
#40814=AXIS2_PLACEMENT_3D('',#56925,#45061,#45062);
#40815=AXIS2_PLACEMENT_3D('',#56927,#45064,#45065);
#40816=AXIS2_PLACEMENT_3D('',#56928,#45066,#45067);
#40817=AXIS2_PLACEMENT_3D('',#56930,#45069,#45070);
#40818=AXIS2_PLACEMENT_3D('',#56932,#45072,#45073);
#40819=AXIS2_PLACEMENT_3D('',#56933,#45074,#45075);
#40820=AXIS2_PLACEMENT_3D('',#56935,#45077,#45078);
#40821=AXIS2_PLACEMENT_3D('',#56937,#45080,#45081);
#40822=AXIS2_PLACEMENT_3D('',#56938,#45082,#45083);
#40823=AXIS2_PLACEMENT_3D('',#56940,#45085,#45086);
#40824=AXIS2_PLACEMENT_3D('',#56942,#45088,#45089);
#40825=AXIS2_PLACEMENT_3D('',#56943,#45090,#45091);
#40826=AXIS2_PLACEMENT_3D('',#56945,#45093,#45094);
#40827=AXIS2_PLACEMENT_3D('',#56947,#45096,#45097);
#40828=AXIS2_PLACEMENT_3D('',#56948,#45098,#45099);
#40829=AXIS2_PLACEMENT_3D('',#56950,#45101,#45102);
#40830=AXIS2_PLACEMENT_3D('',#56952,#45104,#45105);
#40831=AXIS2_PLACEMENT_3D('',#56953,#45106,#45107);
#40832=AXIS2_PLACEMENT_3D('',#56955,#45109,#45110);
#40833=AXIS2_PLACEMENT_3D('',#56957,#45112,#45113);
#40834=AXIS2_PLACEMENT_3D('',#56958,#45114,#45115);
#40835=AXIS2_PLACEMENT_3D('',#56960,#45117,#45118);
#40836=AXIS2_PLACEMENT_3D('',#56962,#45120,#45121);
#40837=AXIS2_PLACEMENT_3D('',#56963,#45122,#45123);
#40838=AXIS2_PLACEMENT_3D('',#56965,#45125,#45126);
#40839=AXIS2_PLACEMENT_3D('',#56967,#45128,#45129);
#40840=AXIS2_PLACEMENT_3D('',#56968,#45130,#45131);
#40841=AXIS2_PLACEMENT_3D('',#56970,#45133,#45134);
#40842=AXIS2_PLACEMENT_3D('',#56972,#45136,#45137);
#40843=AXIS2_PLACEMENT_3D('',#56973,#45138,#45139);
#40844=AXIS2_PLACEMENT_3D('',#56975,#45141,#45142);
#40845=AXIS2_PLACEMENT_3D('',#56977,#45144,#45145);
#40846=AXIS2_PLACEMENT_3D('',#56978,#45146,#45147);
#40847=AXIS2_PLACEMENT_3D('',#56980,#45149,#45150);
#40848=AXIS2_PLACEMENT_3D('',#56982,#45152,#45153);
#40849=AXIS2_PLACEMENT_3D('',#56983,#45154,#45155);
#40850=AXIS2_PLACEMENT_3D('',#56985,#45157,#45158);
#40851=AXIS2_PLACEMENT_3D('',#56987,#45160,#45161);
#40852=AXIS2_PLACEMENT_3D('',#56988,#45162,#45163);
#40853=AXIS2_PLACEMENT_3D('',#56990,#45165,#45166);
#40854=AXIS2_PLACEMENT_3D('',#56992,#45168,#45169);
#40855=AXIS2_PLACEMENT_3D('',#56993,#45170,#45171);
#40856=AXIS2_PLACEMENT_3D('',#56995,#45173,#45174);
#40857=AXIS2_PLACEMENT_3D('',#56997,#45176,#45177);
#40858=AXIS2_PLACEMENT_3D('',#56998,#45178,#45179);
#40859=AXIS2_PLACEMENT_3D('',#57000,#45181,#45182);
#40860=AXIS2_PLACEMENT_3D('',#57002,#45184,#45185);
#40861=AXIS2_PLACEMENT_3D('',#57003,#45186,#45187);
#40862=AXIS2_PLACEMENT_3D('',#57005,#45189,#45190);
#40863=AXIS2_PLACEMENT_3D('',#57007,#45192,#45193);
#40864=AXIS2_PLACEMENT_3D('',#57008,#45194,#45195);
#40865=AXIS2_PLACEMENT_3D('',#57010,#45197,#45198);
#40866=AXIS2_PLACEMENT_3D('',#57012,#45200,#45201);
#40867=AXIS2_PLACEMENT_3D('',#57013,#45202,#45203);
#40868=AXIS2_PLACEMENT_3D('',#57015,#45205,#45206);
#40869=AXIS2_PLACEMENT_3D('',#57017,#45208,#45209);
#40870=AXIS2_PLACEMENT_3D('',#57018,#45210,#45211);
#40871=AXIS2_PLACEMENT_3D('',#57020,#45213,#45214);
#40872=AXIS2_PLACEMENT_3D('',#57022,#45216,#45217);
#40873=AXIS2_PLACEMENT_3D('',#57023,#45218,#45219);
#40874=AXIS2_PLACEMENT_3D('',#57025,#45221,#45222);
#40875=AXIS2_PLACEMENT_3D('',#57027,#45224,#45225);
#40876=AXIS2_PLACEMENT_3D('',#57028,#45226,#45227);
#40877=AXIS2_PLACEMENT_3D('',#57030,#45229,#45230);
#40878=AXIS2_PLACEMENT_3D('',#57032,#45232,#45233);
#40879=AXIS2_PLACEMENT_3D('',#57033,#45234,#45235);
#40880=AXIS2_PLACEMENT_3D('',#57035,#45237,#45238);
#40881=AXIS2_PLACEMENT_3D('',#57037,#45240,#45241);
#40882=AXIS2_PLACEMENT_3D('',#57038,#45242,#45243);
#40883=AXIS2_PLACEMENT_3D('',#57040,#45245,#45246);
#40884=AXIS2_PLACEMENT_3D('',#57042,#45248,#45249);
#40885=AXIS2_PLACEMENT_3D('',#57043,#45250,#45251);
#40886=AXIS2_PLACEMENT_3D('',#57045,#45253,#45254);
#40887=AXIS2_PLACEMENT_3D('',#57047,#45256,#45257);
#40888=AXIS2_PLACEMENT_3D('',#57048,#45258,#45259);
#40889=AXIS2_PLACEMENT_3D('',#57050,#45261,#45262);
#40890=AXIS2_PLACEMENT_3D('',#57052,#45264,#45265);
#40891=AXIS2_PLACEMENT_3D('',#57053,#45266,#45267);
#40892=AXIS2_PLACEMENT_3D('',#57055,#45269,#45270);
#40893=AXIS2_PLACEMENT_3D('',#57057,#45272,#45273);
#40894=AXIS2_PLACEMENT_3D('',#57058,#45274,#45275);
#40895=AXIS2_PLACEMENT_3D('',#57060,#45277,#45278);
#40896=AXIS2_PLACEMENT_3D('',#57062,#45280,#45281);
#40897=AXIS2_PLACEMENT_3D('',#57063,#45282,#45283);
#40898=AXIS2_PLACEMENT_3D('',#57065,#45285,#45286);
#40899=AXIS2_PLACEMENT_3D('',#57067,#45288,#45289);
#40900=AXIS2_PLACEMENT_3D('',#57068,#45290,#45291);
#40901=AXIS2_PLACEMENT_3D('',#57070,#45293,#45294);
#40902=AXIS2_PLACEMENT_3D('',#57072,#45296,#45297);
#40903=AXIS2_PLACEMENT_3D('',#57073,#45298,#45299);
#40904=AXIS2_PLACEMENT_3D('',#57075,#45301,#45302);
#40905=AXIS2_PLACEMENT_3D('',#57077,#45304,#45305);
#40906=AXIS2_PLACEMENT_3D('',#57078,#45306,#45307);
#40907=AXIS2_PLACEMENT_3D('',#57080,#45309,#45310);
#40908=AXIS2_PLACEMENT_3D('',#57082,#45312,#45313);
#40909=AXIS2_PLACEMENT_3D('',#57083,#45314,#45315);
#40910=AXIS2_PLACEMENT_3D('',#57085,#45317,#45318);
#40911=AXIS2_PLACEMENT_3D('',#57087,#45320,#45321);
#40912=AXIS2_PLACEMENT_3D('',#57088,#45322,#45323);
#40913=AXIS2_PLACEMENT_3D('',#57090,#45325,#45326);
#40914=AXIS2_PLACEMENT_3D('',#57092,#45328,#45329);
#40915=AXIS2_PLACEMENT_3D('',#57093,#45330,#45331);
#40916=AXIS2_PLACEMENT_3D('',#57095,#45333,#45334);
#40917=AXIS2_PLACEMENT_3D('',#57097,#45336,#45337);
#40918=AXIS2_PLACEMENT_3D('',#57098,#45338,#45339);
#40919=AXIS2_PLACEMENT_3D('',#57100,#45341,#45342);
#40920=AXIS2_PLACEMENT_3D('',#57102,#45344,#45345);
#40921=AXIS2_PLACEMENT_3D('',#57103,#45346,#45347);
#40922=AXIS2_PLACEMENT_3D('',#57105,#45349,#45350);
#40923=AXIS2_PLACEMENT_3D('',#57107,#45352,#45353);
#40924=AXIS2_PLACEMENT_3D('',#57109,#45355,#45356);
#40925=AXIS2_PLACEMENT_3D('',#57112,#45359,#45360);
#40926=AXIS2_PLACEMENT_3D('',#57114,#45362,#45363);
#40927=AXIS2_PLACEMENT_3D('',#57115,#45364,#45365);
#40928=AXIS2_PLACEMENT_3D('',#57117,#45367,#45368);
#40929=AXIS2_PLACEMENT_3D('',#57118,#45369,#45370);
#40930=AXIS2_PLACEMENT_3D('',#57119,#45371,#45372);
#40931=AXIS2_PLACEMENT_3D('',#57120,#45373,#45374);
#40932=AXIS2_PLACEMENT_3D('',#57122,#45376,#45377);
#40933=AXIS2_PLACEMENT_3D('',#57123,#45378,#45379);
#40934=AXIS2_PLACEMENT_3D('',#57124,#45380,#45381);
#40935=AXIS2_PLACEMENT_3D('',#57125,#45382,#45383);
#40936=AXIS2_PLACEMENT_3D('',#57127,#45385,#45386);
#40937=AXIS2_PLACEMENT_3D('',#57129,#45388,#45389);
#40938=AXIS2_PLACEMENT_3D('',#57131,#45391,#45392);
#40939=AXIS2_PLACEMENT_3D('',#57133,#45394,#45395);
#40940=AXIS2_PLACEMENT_3D('',#57134,#45396,#45397);
#40941=AXIS2_PLACEMENT_3D('',#57135,#45398,#45399);
#40942=AXIS2_PLACEMENT_3D('',#57136,#45400,#45401);
#40943=AXIS2_PLACEMENT_3D('',#57137,#45402,#45403);
#40944=AXIS2_PLACEMENT_3D('',#57138,#45404,#45405);
#40945=AXIS2_PLACEMENT_3D('',#57139,#45406,#45407);
#40946=AXIS2_PLACEMENT_3D('',#57140,#45408,#45409);
#40947=AXIS2_PLACEMENT_3D('',#57142,#45410,#45411);
#40948=AXIS2_PLACEMENT_3D('',#57145,#45413,#45414);
#40949=AXIS2_PLACEMENT_3D('',#57146,#45415,#45416);
#40950=AXIS2_PLACEMENT_3D('',#57148,#45417,#45418);
#40951=AXIS2_PLACEMENT_3D('',#57151,#45420,#45421);
#40952=AXIS2_PLACEMENT_3D('',#57152,#45422,#45423);
#40953=AXIS2_PLACEMENT_3D('',#57154,#45424,#45425);
#40954=AXIS2_PLACEMENT_3D('',#57158,#45427,#45428);
#40955=AXIS2_PLACEMENT_3D('',#57162,#45430,#45431);
#40956=AXIS2_PLACEMENT_3D('',#57165,#45433,#45434);
#40957=AXIS2_PLACEMENT_3D('',#57169,#45436,#45437);
#40958=AXIS2_PLACEMENT_3D('',#57173,#45439,#45440);
#40959=AXIS2_PLACEMENT_3D('',#57175,#45442,#45443);
#40960=AXIS2_PLACEMENT_3D('',#57177,#45444,#45445);
#40961=AXIS2_PLACEMENT_3D('',#57181,#45447,#45448);
#40962=AXIS2_PLACEMENT_3D('',#57185,#45450,#45451);
#40963=AXIS2_PLACEMENT_3D('',#57188,#45453,#45454);
#40964=AXIS2_PLACEMENT_3D('',#57192,#45456,#45457);
#40965=AXIS2_PLACEMENT_3D('',#57196,#45459,#45460);
#40966=AXIS2_PLACEMENT_3D('',#57198,#45462,#45463);
#40967=AXIS2_PLACEMENT_3D('',#57201,#45466,#45467);
#40968=AXIS2_PLACEMENT_3D('',#57204,#45470,#45471);
#40969=AXIS2_PLACEMENT_3D('',#57205,#45472,#45473);
#40970=AXIS2_PLACEMENT_3D('',#57206,#45474,#45475);
#40971=AXIS2_PLACEMENT_3D('',#57207,#45476,#45477);
#40972=AXIS2_PLACEMENT_3D('',#57210,#45480,#45481);
#40973=AXIS2_PLACEMENT_3D('',#57213,#45484,#45485);
#40974=AXIS2_PLACEMENT_3D('',#57215,#45487,#45488);
#40975=AXIS2_PLACEMENT_3D('',#57217,#45490,#45491);
#40976=AXIS2_PLACEMENT_3D('',#57218,#45492,#45493);
#40977=AXIS2_PLACEMENT_3D('',#57219,#45494,#45495);
#40978=AXIS2_PLACEMENT_3D('',#57220,#45496,#45497);
#40979=AXIS2_PLACEMENT_3D('',#57221,#45498,#45499);
#40980=AXIS2_PLACEMENT_3D('',#57222,#45500,#45501);
#40981=AXIS2_PLACEMENT_3D('',#57223,#45502,#45503);
#40982=AXIS2_PLACEMENT_3D('',#57224,#45504,#45505);
#40983=AXIS2_PLACEMENT_3D('',#57225,#45506,#45507);
#40984=AXIS2_PLACEMENT_3D('',#57226,#45508,#45509);
#40985=AXIS2_PLACEMENT_3D('',#57228,#45510,#45511);
#40986=AXIS2_PLACEMENT_3D('',#57231,#45513,#45514);
#40987=AXIS2_PLACEMENT_3D('',#57232,#45515,#45516);
#40988=AXIS2_PLACEMENT_3D('',#57234,#45517,#45518);
#40989=AXIS2_PLACEMENT_3D('',#57237,#45520,#45521);
#40990=AXIS2_PLACEMENT_3D('',#57238,#45522,#45523);
#40991=AXIS2_PLACEMENT_3D('',#57240,#45524,#45525);
#40992=AXIS2_PLACEMENT_3D('',#57244,#45527,#45528);
#40993=AXIS2_PLACEMENT_3D('',#57248,#45530,#45531);
#40994=AXIS2_PLACEMENT_3D('',#57251,#45533,#45534);
#40995=AXIS2_PLACEMENT_3D('',#57255,#45536,#45537);
#40996=AXIS2_PLACEMENT_3D('',#57259,#45539,#45540);
#40997=AXIS2_PLACEMENT_3D('',#57261,#45542,#45543);
#40998=AXIS2_PLACEMENT_3D('',#57263,#45544,#45545);
#40999=AXIS2_PLACEMENT_3D('',#57267,#45547,#45548);
#41000=AXIS2_PLACEMENT_3D('',#57271,#45550,#45551);
#41001=AXIS2_PLACEMENT_3D('',#57274,#45553,#45554);
#41002=AXIS2_PLACEMENT_3D('',#57278,#45556,#45557);
#41003=AXIS2_PLACEMENT_3D('',#57282,#45559,#45560);
#41004=AXIS2_PLACEMENT_3D('',#57284,#45562,#45563);
#41005=AXIS2_PLACEMENT_3D('',#57287,#45566,#45567);
#41006=AXIS2_PLACEMENT_3D('',#57290,#45570,#45571);
#41007=AXIS2_PLACEMENT_3D('',#57291,#45572,#45573);
#41008=AXIS2_PLACEMENT_3D('',#57292,#45574,#45575);
#41009=AXIS2_PLACEMENT_3D('',#57293,#45576,#45577);
#41010=AXIS2_PLACEMENT_3D('',#57296,#45580,#45581);
#41011=AXIS2_PLACEMENT_3D('',#57299,#45584,#45585);
#41012=AXIS2_PLACEMENT_3D('',#57301,#45587,#45588);
#41013=AXIS2_PLACEMENT_3D('',#57303,#45590,#45591);
#41014=AXIS2_PLACEMENT_3D('',#57304,#45592,#45593);
#41015=AXIS2_PLACEMENT_3D('',#57305,#45594,#45595);
#41016=AXIS2_PLACEMENT_3D('',#57306,#45596,#45597);
#41017=AXIS2_PLACEMENT_3D('',#57308,#45599,#45600);
#41018=AXIS2_PLACEMENT_3D('',#57310,#45602,#45603);
#41019=AXIS2_PLACEMENT_3D('',#57312,#45605,#45606);
#41020=AXIS2_PLACEMENT_3D('',#57315,#45609,#45610);
#41021=AXIS2_PLACEMENT_3D('',#57317,#45612,#45613);
#41022=AXIS2_PLACEMENT_3D('',#57318,#45614,#45615);
#41023=AXIS2_PLACEMENT_3D('',#57322,#45617,#45618);
#41024=AXIS2_PLACEMENT_3D('',#57323,#45619,#45620);
#41025=AXIS2_PLACEMENT_3D('',#57324,#45621,#45622);
#41026=AXIS2_PLACEMENT_3D('',#57326,#45623,#45624);
#41027=AXIS2_PLACEMENT_3D('',#57329,#45626,#45627);
#41028=AXIS2_PLACEMENT_3D('',#57330,#45628,#45629);
#41029=AXIS2_PLACEMENT_3D('',#57332,#45631,#45632);
#41030=AXIS2_PLACEMENT_3D('',#57334,#45634,#45635);
#41031=AXIS2_PLACEMENT_3D('',#57340,#45639,#45640);
#41032=AXIS2_PLACEMENT_3D('',#57346,#45644,#45645);
#41033=AXIS2_PLACEMENT_3D('',#57348,#45646,#45647);
#41034=AXIS2_PLACEMENT_3D('',#57351,#45649,#45650);
#41035=AXIS2_PLACEMENT_3D('',#57352,#45651,#45652);
#41036=AXIS2_PLACEMENT_3D('',#57354,#45653,#45654);
#41037=AXIS2_PLACEMENT_3D('',#57357,#45656,#45657);
#41038=AXIS2_PLACEMENT_3D('',#57358,#45658,#45659);
#41039=AXIS2_PLACEMENT_3D('',#57360,#45661,#45662);
#41040=AXIS2_PLACEMENT_3D('',#57362,#45664,#45665);
#42516=DIRECTION('axis',(0.,0.,1.));
#42517=DIRECTION('refdir',(1.,0.,0.));
#42518=DIRECTION('center_axis',(-1.,-4.38245930773088E-16,0.));
#42519=DIRECTION('ref_axis',(4.38245930773088E-16,-1.,0.));
#42520=DIRECTION('center_axis',(-1.,-4.38245930773088E-16,0.));
#42521=DIRECTION('ref_axis',(4.38245930773088E-16,-1.,0.));
#42522=DIRECTION('',(-1.,-4.38245930773088E-16,0.));
#42523=DIRECTION('center_axis',(-1.,-4.38245930773088E-16,0.));
#42524=DIRECTION('ref_axis',(-4.38245930773088E-16,1.,0.));
#42525=DIRECTION('center_axis',(-1.,-4.38245930773088E-16,0.));
#42526=DIRECTION('ref_axis',(4.38245930773088E-16,-1.,0.));
#42527=DIRECTION('center_axis',(-1.,-4.38245930773088E-16,0.));
#42528=DIRECTION('ref_axis',(4.38245930773088E-16,-1.,0.));
#42529=DIRECTION('',(-1.,-4.38245930773088E-16,0.));
#42530=DIRECTION('center_axis',(-1.,-4.38245930773088E-16,0.));
#42531=DIRECTION('ref_axis',(4.38245930773088E-16,-1.,0.));
#42532=DIRECTION('center_axis',(-1.,-4.38245930773088E-16,0.));
#42533=DIRECTION('ref_axis',(4.38245930773088E-16,-1.,0.));
#42534=DIRECTION('center_axis',(-1.,-4.38245930773088E-16,0.));
#42535=DIRECTION('ref_axis',(4.38245930773088E-16,-1.,0.));
#42536=DIRECTION('',(-1.,-4.38245930773088E-16,0.));
#42537=DIRECTION('center_axis',(-1.,-4.38245930773088E-16,0.));
#42538=DIRECTION('ref_axis',(-4.38245930773088E-16,1.,0.));
#42539=DIRECTION('center_axis',(-1.,-4.38245930773088E-16,0.));
#42540=DIRECTION('ref_axis',(4.38245930773088E-16,-1.,0.));
#42541=DIRECTION('center_axis',(-1.,-4.38245930773088E-16,0.));
#42542=DIRECTION('ref_axis',(4.38245930773088E-16,-1.,0.));
#42543=DIRECTION('',(-1.,-4.38245930773088E-16,0.));
#42544=DIRECTION('center_axis',(-1.,-4.38245930773088E-16,0.));
#42545=DIRECTION('ref_axis',(4.38245930773088E-16,-1.,0.));
#42546=DIRECTION('center_axis',(0.,0.,-1.));
#42547=DIRECTION('ref_axis',(-1.,0.,0.));
#42548=DIRECTION('center_axis',(0.,0.,-1.));
#42549=DIRECTION('ref_axis',(0.,-1.,0.));
#42550=DIRECTION('',(0.,0.,-1.));
#42551=DIRECTION('center_axis',(0.,0.,-1.));
#42552=DIRECTION('ref_axis',(1.,0.,0.));
#42553=DIRECTION('center_axis',(0.,0.,-1.));
#42554=DIRECTION('ref_axis',(-1.,0.,0.));
#42555=DIRECTION('center_axis',(0.,0.,1.));
#42556=DIRECTION('ref_axis',(0.,-1.,0.));
#42557=DIRECTION('',(0.,0.,-1.));
#42558=DIRECTION('center_axis',(0.,0.,1.));
#42559=DIRECTION('ref_axis',(-1.,0.,0.));
#42560=DIRECTION('center_axis',(1.,1.46081976924362E-16,0.));
#42561=DIRECTION('ref_axis',(-1.46081976924362E-16,1.,0.));
#42562=DIRECTION('center_axis',(1.,1.46081976924362E-16,0.));
#42563=DIRECTION('ref_axis',(-1.46081976924362E-16,1.,0.));
#42564=DIRECTION('',(1.,1.46081976924362E-16,0.));
#42565=DIRECTION('center_axis',(1.,1.92420077553238E-16,0.));
#42566=DIRECTION('ref_axis',(-1.92420077553238E-16,1.,0.));
#42567=DIRECTION('',(1.,1.46081976924362E-16,0.));
#42568=DIRECTION('center_axis',(1.,1.46081976924362E-16,0.));
#42569=DIRECTION('ref_axis',(-1.46081976924362E-16,1.,0.));
#42570=DIRECTION('center_axis',(-1.,-1.46081976924362E-16,0.));
#42571=DIRECTION('ref_axis',(-1.46081976924362E-16,1.,0.));
#42572=DIRECTION('',(1.,1.46081976924362E-16,0.));
#42573=DIRECTION('center_axis',(-1.,-1.92420077553238E-16,0.));
#42574=DIRECTION('ref_axis',(-1.92420077553238E-16,1.,0.));
#42575=DIRECTION('',(1.,1.46081976924362E-16,0.));
#42576=DIRECTION('center_axis',(1.,1.46081976924362E-16,0.));
#42577=DIRECTION('ref_axis',(-1.46081976924362E-16,1.,0.));
#42578=DIRECTION('center_axis',(-1.,-1.46081976924362E-16,0.));
#42579=DIRECTION('ref_axis',(-1.46081976924362E-16,1.,0.));
#42580=DIRECTION('',(1.,1.46081976924362E-16,0.));
#42581=DIRECTION('center_axis',(-1.,-1.92420077553238E-16,0.));
#42582=DIRECTION('ref_axis',(-1.92420077553238E-16,1.,0.));
#42583=DIRECTION('',(1.,1.46081976924362E-16,0.));
#42584=DIRECTION('center_axis',(1.,1.46081976924362E-16,0.));
#42585=DIRECTION('ref_axis',(-1.46081976924362E-16,1.,0.));
#42586=DIRECTION('center_axis',(-1.,-1.46081976924362E-16,0.));
#42587=DIRECTION('ref_axis',(-1.46081976924362E-16,1.,0.));
#42588=DIRECTION('',(1.,1.46081976924362E-16,0.));
#42589=DIRECTION('center_axis',(-1.,-1.92420077553238E-16,0.));
#42590=DIRECTION('ref_axis',(-1.92420077553238E-16,1.,0.));
#42591=DIRECTION('',(1.,1.46081976924362E-16,0.));
#42592=DIRECTION('center_axis',(1.,1.46081976924362E-16,0.));
#42593=DIRECTION('ref_axis',(-1.46081976924362E-16,1.,0.));
#42594=DIRECTION('center_axis',(-1.,-1.46081976924362E-16,0.));
#42595=DIRECTION('ref_axis',(-1.46081976924362E-16,1.,0.));
#42596=DIRECTION('',(1.,1.46081976924362E-16,0.));
#42597=DIRECTION('center_axis',(-1.,-1.92420077553238E-16,0.));
#42598=DIRECTION('ref_axis',(-1.92420077553238E-16,1.,0.));
#42599=DIRECTION('',(1.,1.46081976924362E-16,0.));
#42600=DIRECTION('center_axis',(1.,1.46081976924362E-16,0.));
#42601=DIRECTION('ref_axis',(-1.46081976924362E-16,1.,0.));
#42602=DIRECTION('center_axis',(-1.,-1.46081976924362E-16,0.));
#42603=DIRECTION('ref_axis',(-1.46081976924362E-16,1.,0.));
#42604=DIRECTION('',(1.,1.46081976924362E-16,0.));
#42605=DIRECTION('center_axis',(-1.,-1.92420077553238E-16,0.));
#42606=DIRECTION('ref_axis',(-1.92420077553238E-16,1.,0.));
#42607=DIRECTION('',(1.,1.46081976924362E-16,0.));
#42608=DIRECTION('center_axis',(1.,1.46081976924362E-16,0.));
#42609=DIRECTION('ref_axis',(-1.46081976924362E-16,1.,0.));
#42610=DIRECTION('center_axis',(1.,1.46081976924362E-16,0.));
#42611=DIRECTION('ref_axis',(-1.46081976924362E-16,1.,0.));
#42612=DIRECTION('',(1.,1.46081976924362E-16,0.));
#42613=DIRECTION('center_axis',(1.,1.92420077553238E-16,0.));
#42614=DIRECTION('ref_axis',(-1.92420077553238E-16,1.,0.));
#42615=DIRECTION('',(1.,1.46081976924362E-16,0.));
#42616=DIRECTION('center_axis',(1.,1.46081976924362E-16,0.));
#42617=DIRECTION('ref_axis',(-1.46081976924362E-16,1.,0.));
#42618=DIRECTION('center_axis',(1.,1.46081976924362E-16,0.));
#42619=DIRECTION('ref_axis',(-1.46081976924362E-16,1.,0.));
#42620=DIRECTION('',(1.,1.46081976924362E-16,0.));
#42621=DIRECTION('center_axis',(1.,1.92420077553238E-16,0.));
#42622=DIRECTION('ref_axis',(-1.92420077553238E-16,1.,0.));
#42623=DIRECTION('',(1.,1.46081976924362E-16,0.));
#42624=DIRECTION('center_axis',(1.,1.46081976924362E-16,0.));
#42625=DIRECTION('ref_axis',(-1.46081976924362E-16,1.,0.));
#42626=DIRECTION('center_axis',(1.,1.46081976924362E-16,0.));
#42627=DIRECTION('ref_axis',(-1.46081976924362E-16,1.,0.));
#42628=DIRECTION('',(1.,1.46081976924362E-16,0.));
#42629=DIRECTION('center_axis',(1.,1.92420077553238E-16,0.));
#42630=DIRECTION('ref_axis',(-1.92420077553238E-16,1.,0.));
#42631=DIRECTION('',(1.,1.46081976924362E-16,0.));
#42632=DIRECTION('center_axis',(1.,1.46081976924362E-16,0.));
#42633=DIRECTION('ref_axis',(-1.46081976924362E-16,1.,0.));
#42634=DIRECTION('center_axis',(1.,1.46081976924362E-16,0.));
#42635=DIRECTION('ref_axis',(-1.46081976924362E-16,1.,0.));
#42636=DIRECTION('',(1.,1.46081976924362E-16,0.));
#42637=DIRECTION('center_axis',(1.,1.92420077553238E-16,0.));
#42638=DIRECTION('ref_axis',(-1.92420077553238E-16,1.,0.));
#42639=DIRECTION('',(1.,1.46081976924362E-16,0.));
#42640=DIRECTION('center_axis',(1.,1.46081976924362E-16,0.));
#42641=DIRECTION('ref_axis',(-1.46081976924362E-16,1.,0.));
#42642=DIRECTION('center_axis',(1.,1.46081976924362E-16,0.));
#42643=DIRECTION('ref_axis',(-1.46081976924362E-16,1.,0.));
#42644=DIRECTION('',(1.,1.46081976924362E-16,0.));
#42645=DIRECTION('center_axis',(1.,1.92420077553238E-16,0.));
#42646=DIRECTION('ref_axis',(-1.92420077553238E-16,1.,0.));
#42647=DIRECTION('',(1.,1.46081976924362E-16,0.));
#42648=DIRECTION('center_axis',(1.,1.46081976924362E-16,0.));
#42649=DIRECTION('ref_axis',(-1.46081976924362E-16,1.,0.));
#42650=DIRECTION('center_axis',(1.,1.46081976924362E-16,0.));
#42651=DIRECTION('ref_axis',(-1.46081976924362E-16,1.,0.));
#42652=DIRECTION('',(1.,1.46081976924362E-16,0.));
#42653=DIRECTION('center_axis',(1.,1.92420077553238E-16,0.));
#42654=DIRECTION('ref_axis',(-1.92420077553238E-16,1.,0.));
#42655=DIRECTION('',(1.,1.46081976924362E-16,0.));
#42656=DIRECTION('center_axis',(1.,1.46081976924362E-16,0.));
#42657=DIRECTION('ref_axis',(-1.46081976924362E-16,1.,0.));
#42658=DIRECTION('center_axis',(1.,1.46081976924362E-16,0.));
#42659=DIRECTION('ref_axis',(-1.46081976924362E-16,1.,0.));
#42660=DIRECTION('',(1.,1.46081976924362E-16,0.));
#42661=DIRECTION('center_axis',(1.,1.92420077553238E-16,0.));
#42662=DIRECTION('ref_axis',(-1.92420077553238E-16,1.,0.));
#42663=DIRECTION('',(1.,1.46081976924362E-16,0.));
#42664=DIRECTION('center_axis',(1.,1.46081976924362E-16,0.));
#42665=DIRECTION('ref_axis',(-1.46081976924362E-16,1.,0.));
#42666=DIRECTION('center_axis',(-1.,-1.46081976924362E-16,0.));
#42667=DIRECTION('ref_axis',(-1.46081976924362E-16,1.,0.));
#42668=DIRECTION('',(1.,1.46081976924362E-16,0.));
#42669=DIRECTION('center_axis',(-1.,-1.92420077553238E-16,0.));
#42670=DIRECTION('ref_axis',(-1.92420077553238E-16,1.,0.));
#42671=DIRECTION('',(1.,1.46081976924362E-16,0.));
#42672=DIRECTION('center_axis',(1.,1.46081976924362E-16,0.));
#42673=DIRECTION('ref_axis',(-1.46081976924362E-16,1.,0.));
#42674=DIRECTION('center_axis',(-1.,-1.46081976924362E-16,0.));
#42675=DIRECTION('ref_axis',(-1.46081976924362E-16,1.,0.));
#42676=DIRECTION('',(1.,1.46081976924362E-16,0.));
#42677=DIRECTION('center_axis',(-1.,-1.92420077553238E-16,0.));
#42678=DIRECTION('ref_axis',(-1.92420077553238E-16,1.,0.));
#42679=DIRECTION('',(1.,1.46081976924362E-16,0.));
#42680=DIRECTION('center_axis',(1.,1.46081976924362E-16,0.));
#42681=DIRECTION('ref_axis',(-1.46081976924362E-16,1.,0.));
#42682=DIRECTION('center_axis',(-1.,-1.46081976924362E-16,0.));
#42683=DIRECTION('ref_axis',(-1.46081976924362E-16,1.,0.));
#42684=DIRECTION('',(1.,1.46081976924362E-16,0.));
#42685=DIRECTION('center_axis',(-1.,-1.92420077553238E-16,0.));
#42686=DIRECTION('ref_axis',(-1.92420077553238E-16,1.,0.));
#42687=DIRECTION('',(1.,1.46081976924362E-16,0.));
#42688=DIRECTION('center_axis',(1.,1.46081976924362E-16,0.));
#42689=DIRECTION('ref_axis',(-1.46081976924362E-16,1.,0.));
#42690=DIRECTION('center_axis',(-1.,-1.46081976924362E-16,0.));
#42691=DIRECTION('ref_axis',(-1.46081976924362E-16,1.,1.15648231731787E-15));
#42692=DIRECTION('',(1.,1.46081976924362E-16,0.));
#42693=DIRECTION('center_axis',(-1.,-1.92420077553238E-16,0.));
#42694=DIRECTION('ref_axis',(-1.92420077553238E-16,1.,0.));
#42695=DIRECTION('',(1.,1.46081976924362E-16,0.));
#42696=DIRECTION('center_axis',(1.,1.46081976924362E-16,0.));
#42697=DIRECTION('ref_axis',(-1.46081976924362E-16,1.,0.));
#42698=DIRECTION('center_axis',(1.,1.46081976924362E-16,0.));
#42699=DIRECTION('ref_axis',(-1.46081976924362E-16,1.,0.));
#42700=DIRECTION('',(1.,1.46081976924362E-16,0.));
#42701=DIRECTION('center_axis',(1.,1.92420077553238E-16,0.));
#42702=DIRECTION('ref_axis',(-1.92420077553238E-16,1.,0.));
#42703=DIRECTION('',(1.,1.46081976924362E-16,0.));
#42704=DIRECTION('center_axis',(1.,1.46081976924362E-16,0.));
#42705=DIRECTION('ref_axis',(-1.46081976924362E-16,1.,0.));
#42706=DIRECTION('center_axis',(1.,1.46081976924362E-16,0.));
#42707=DIRECTION('ref_axis',(-1.46081976924362E-16,1.,0.));
#42708=DIRECTION('',(1.,1.46081976924362E-16,0.));
#42709=DIRECTION('center_axis',(1.,1.92420077553238E-16,0.));
#42710=DIRECTION('ref_axis',(-1.92420077553238E-16,1.,0.));
#42711=DIRECTION('',(1.,1.46081976924362E-16,0.));
#42712=DIRECTION('center_axis',(1.,1.46081976924362E-16,0.));
#42713=DIRECTION('ref_axis',(-1.46081976924362E-16,1.,0.));
#42714=DIRECTION('center_axis',(-1.,-1.46081976924362E-16,0.));
#42715=DIRECTION('ref_axis',(-1.46081976924362E-16,1.,0.));
#42716=DIRECTION('',(1.,1.46081976924362E-16,0.));
#42717=DIRECTION('center_axis',(-1.,-1.92420077553238E-16,0.));
#42718=DIRECTION('ref_axis',(-1.92420077553238E-16,1.,0.));
#42719=DIRECTION('',(1.,1.46081976924362E-16,0.));
#42720=DIRECTION('center_axis',(1.,1.46081976924362E-16,0.));
#42721=DIRECTION('ref_axis',(-1.46081976924362E-16,1.,0.));
#42722=DIRECTION('center_axis',(1.,1.46081976924362E-16,0.));
#42723=DIRECTION('ref_axis',(-1.46081976924362E-16,1.,0.));
#42724=DIRECTION('',(1.,1.46081976924362E-16,0.));
#42725=DIRECTION('center_axis',(1.,1.92420077553238E-16,0.));
#42726=DIRECTION('ref_axis',(-1.92420077553238E-16,1.,0.));
#42727=DIRECTION('',(1.,1.46081976924362E-16,0.));
#42728=DIRECTION('center_axis',(1.,1.46081976924362E-16,0.));
#42729=DIRECTION('ref_axis',(-1.46081976924362E-16,1.,0.));
#42730=DIRECTION('center_axis',(-1.,-1.46081976924362E-16,0.));
#42731=DIRECTION('ref_axis',(-1.46081976924362E-16,1.,0.));
#42732=DIRECTION('',(1.,1.46081976924362E-16,0.));
#42733=DIRECTION('center_axis',(-1.,-1.92420077553238E-16,0.));
#42734=DIRECTION('ref_axis',(-1.92420077553238E-16,1.,0.));
#42735=DIRECTION('',(1.,1.46081976924362E-16,0.));
#42736=DIRECTION('center_axis',(1.,1.46081976924362E-16,0.));
#42737=DIRECTION('ref_axis',(-1.46081976924362E-16,1.,0.));
#42738=DIRECTION('center_axis',(-1.,-1.46081976924362E-16,0.));
#42739=DIRECTION('ref_axis',(-1.46081976924362E-16,1.,0.));
#42740=DIRECTION('',(1.,1.46081976924362E-16,0.));
#42741=DIRECTION('center_axis',(-1.,-1.92420077553238E-16,0.));
#42742=DIRECTION('ref_axis',(-1.92420077553238E-16,1.,0.));
#42743=DIRECTION('',(1.,1.46081976924362E-16,0.));
#42744=DIRECTION('center_axis',(1.,1.46081976924362E-16,0.));
#42745=DIRECTION('ref_axis',(-1.46081976924362E-16,1.,0.));
#42746=DIRECTION('center_axis',(1.,1.46081976924362E-16,0.));
#42747=DIRECTION('ref_axis',(-1.46081976924362E-16,1.,0.));
#42748=DIRECTION('',(1.,1.46081976924362E-16,0.));
#42749=DIRECTION('center_axis',(1.,1.92420077553238E-16,0.));
#42750=DIRECTION('ref_axis',(-1.92420077553238E-16,1.,0.));
#42751=DIRECTION('',(1.,1.46081976924362E-16,0.));
#42752=DIRECTION('center_axis',(1.,1.46081976924362E-16,0.));
#42753=DIRECTION('ref_axis',(-1.46081976924362E-16,1.,0.));
#42754=DIRECTION('center_axis',(-1.,-1.46081976924362E-16,0.));
#42755=DIRECTION('ref_axis',(-1.46081976924362E-16,1.,0.));
#42756=DIRECTION('',(1.,1.46081976924362E-16,0.));
#42757=DIRECTION('center_axis',(-1.,-1.92420077553238E-16,0.));
#42758=DIRECTION('ref_axis',(-1.92420077553238E-16,1.,0.));
#42759=DIRECTION('',(1.,1.46081976924362E-16,0.));
#42760=DIRECTION('center_axis',(1.,1.46081976924362E-16,0.));
#42761=DIRECTION('ref_axis',(-1.46081976924362E-16,1.,0.));
#42762=DIRECTION('center_axis',(1.,1.46081976924362E-16,0.));
#42763=DIRECTION('ref_axis',(-1.46081976924362E-16,1.,0.));
#42764=DIRECTION('',(1.,1.46081976924362E-16,0.));
#42765=DIRECTION('center_axis',(1.,1.92420077553238E-16,0.));
#42766=DIRECTION('ref_axis',(-1.92420077553238E-16,1.,0.));
#42767=DIRECTION('',(1.,1.46081976924362E-16,0.));
#42768=DIRECTION('center_axis',(1.,1.46081976924362E-16,0.));
#42769=DIRECTION('ref_axis',(-1.46081976924362E-16,1.,0.));
#42770=DIRECTION('center_axis',(1.,1.46081976924362E-16,0.));
#42771=DIRECTION('ref_axis',(-1.46081976924362E-16,1.,0.));
#42772=DIRECTION('',(1.,1.46081976924362E-16,0.));
#42773=DIRECTION('center_axis',(1.,1.92420077553238E-16,0.));
#42774=DIRECTION('ref_axis',(-1.92420077553238E-16,1.,0.));
#42775=DIRECTION('',(1.,1.46081976924362E-16,0.));
#42776=DIRECTION('center_axis',(1.,1.46081976924362E-16,0.));
#42777=DIRECTION('ref_axis',(-1.46081976924362E-16,1.,0.));
#42778=DIRECTION('center_axis',(1.,1.46081976924362E-16,0.));
#42779=DIRECTION('ref_axis',(-1.46081976924362E-16,1.,0.));
#42780=DIRECTION('',(1.,1.46081976924362E-16,0.));
#42781=DIRECTION('center_axis',(1.,1.92420077553238E-16,0.));
#42782=DIRECTION('ref_axis',(-1.92420077553238E-16,1.,0.));
#42783=DIRECTION('',(1.,1.46081976924362E-16,0.));
#42784=DIRECTION('center_axis',(1.,1.46081976924362E-16,0.));
#42785=DIRECTION('ref_axis',(-1.46081976924362E-16,1.,0.));
#42786=DIRECTION('center_axis',(1.,1.46081976924362E-16,0.));
#42787=DIRECTION('ref_axis',(-1.46081976924362E-16,1.,0.));
#42788=DIRECTION('',(1.,1.46081976924362E-16,0.));
#42789=DIRECTION('center_axis',(1.,1.92420077553238E-16,0.));
#42790=DIRECTION('ref_axis',(-1.92420077553238E-16,1.,0.));
#42791=DIRECTION('',(1.,1.46081976924362E-16,0.));
#42792=DIRECTION('center_axis',(1.,1.46081976924362E-16,0.));
#42793=DIRECTION('ref_axis',(-1.46081976924362E-16,1.,0.));
#42794=DIRECTION('center_axis',(1.,1.46081976924362E-16,0.));
#42795=DIRECTION('ref_axis',(-1.46081976924362E-16,1.,0.));
#42796=DIRECTION('',(1.,1.46081976924362E-16,0.));
#42797=DIRECTION('center_axis',(1.,1.92420077553238E-16,0.));
#42798=DIRECTION('ref_axis',(-1.92420077553238E-16,1.,0.));
#42799=DIRECTION('',(1.,1.46081976924362E-16,0.));
#42800=DIRECTION('center_axis',(1.,1.46081976924362E-16,0.));
#42801=DIRECTION('ref_axis',(-1.46081976924362E-16,1.,0.));
#42802=DIRECTION('center_axis',(-1.,-1.46081976924362E-16,0.));
#42803=DIRECTION('ref_axis',(-1.46081976924362E-16,1.,0.));
#42804=DIRECTION('',(1.,1.46081976924362E-16,0.));
#42805=DIRECTION('center_axis',(-1.,-1.92420077553238E-16,0.));
#42806=DIRECTION('ref_axis',(-1.92420077553238E-16,1.,0.));
#42807=DIRECTION('',(1.,1.46081976924362E-16,0.));
#42808=DIRECTION('center_axis',(1.,1.46081976924362E-16,0.));
#42809=DIRECTION('ref_axis',(-1.46081976924362E-16,1.,0.));
#42810=DIRECTION('center_axis',(-1.,-1.46081976924362E-16,0.));
#42811=DIRECTION('ref_axis',(-1.46081976924362E-16,1.,0.));
#42812=DIRECTION('',(1.,1.46081976924362E-16,0.));
#42813=DIRECTION('center_axis',(-1.,-1.92420077553238E-16,0.));
#42814=DIRECTION('ref_axis',(-1.92420077553238E-16,1.,0.));
#42815=DIRECTION('',(1.,1.46081976924362E-16,0.));
#42816=DIRECTION('center_axis',(1.,1.46081976924362E-16,0.));
#42817=DIRECTION('ref_axis',(-1.46081976924362E-16,1.,0.));
#42818=DIRECTION('center_axis',(-1.,-1.46081976924362E-16,0.));
#42819=DIRECTION('ref_axis',(-1.46081976924362E-16,1.,0.));
#42820=DIRECTION('',(1.,1.46081976924362E-16,0.));
#42821=DIRECTION('center_axis',(-1.,-1.92420077553238E-16,0.));
#42822=DIRECTION('ref_axis',(-1.92420077553238E-16,1.,0.));
#42823=DIRECTION('',(1.,1.46081976924362E-16,0.));
#42824=DIRECTION('center_axis',(1.,1.46081976924362E-16,0.));
#42825=DIRECTION('ref_axis',(-1.46081976924362E-16,1.,0.));
#42826=DIRECTION('center_axis',(-1.,-1.46081976924362E-16,0.));
#42827=DIRECTION('ref_axis',(-1.46081976924362E-16,1.,0.));
#42828=DIRECTION('',(1.,1.46081976924362E-16,0.));
#42829=DIRECTION('center_axis',(-1.,-1.92420077553238E-16,0.));
#42830=DIRECTION('ref_axis',(-1.92420077553238E-16,1.,0.));
#42831=DIRECTION('',(1.,1.46081976924362E-16,0.));
#42832=DIRECTION('center_axis',(1.,1.46081976924362E-16,0.));
#42833=DIRECTION('ref_axis',(-1.46081976924362E-16,1.,0.));
#42834=DIRECTION('center_axis',(-1.,-1.46081976924362E-16,0.));
#42835=DIRECTION('ref_axis',(-1.46081976924362E-16,1.,0.));
#42836=DIRECTION('',(1.,1.46081976924362E-16,0.));
#42837=DIRECTION('center_axis',(-1.,-1.92420077553238E-16,0.));
#42838=DIRECTION('ref_axis',(-1.92420077553238E-16,1.,0.));
#42839=DIRECTION('',(1.,1.46081976924362E-16,0.));
#42840=DIRECTION('center_axis',(1.,1.46081976924362E-16,0.));
#42841=DIRECTION('ref_axis',(-1.46081976924362E-16,1.,0.));
#42842=DIRECTION('center_axis',(-1.,-1.46081976924362E-16,0.));
#42843=DIRECTION('ref_axis',(-1.46081976924362E-16,1.,0.));
#42844=DIRECTION('',(1.,1.46081976924362E-16,0.));
#42845=DIRECTION('center_axis',(-1.,-1.92420077553238E-16,0.));
#42846=DIRECTION('ref_axis',(-1.92420077553238E-16,1.,0.));
#42847=DIRECTION('',(1.,1.46081976924362E-16,0.));
#42848=DIRECTION('center_axis',(1.,1.46081976924362E-16,0.));
#42849=DIRECTION('ref_axis',(-1.46081976924362E-16,1.,0.));
#42850=DIRECTION('center_axis',(-1.,-1.46081976924362E-16,0.));
#42851=DIRECTION('ref_axis',(-1.46081976924362E-16,1.,0.));
#42852=DIRECTION('',(1.,1.46081976924362E-16,0.));
#42853=DIRECTION('center_axis',(-1.,-1.92420077553238E-16,0.));
#42854=DIRECTION('ref_axis',(-1.92420077553238E-16,1.,0.));
#42855=DIRECTION('',(1.,1.46081976924362E-16,0.));
#42856=DIRECTION('center_axis',(1.,1.46081976924362E-16,0.));
#42857=DIRECTION('ref_axis',(-1.46081976924362E-16,1.,0.));
#42858=DIRECTION('center_axis',(1.,1.46081976924362E-16,0.));
#42859=DIRECTION('ref_axis',(-1.46081976924362E-16,1.,0.));
#42860=DIRECTION('',(1.,1.46081976924362E-16,0.));
#42861=DIRECTION('center_axis',(1.,1.92420077553238E-16,0.));
#42862=DIRECTION('ref_axis',(-1.92420077553238E-16,1.,0.));
#42863=DIRECTION('',(1.,1.46081976924362E-16,0.));
#42864=DIRECTION('center_axis',(1.,1.46081976924362E-16,0.));
#42865=DIRECTION('ref_axis',(-1.46081976924362E-16,1.,0.));
#42866=DIRECTION('center_axis',(1.,1.46081976924362E-16,0.));
#42867=DIRECTION('ref_axis',(-1.46081976924362E-16,1.,0.));
#42868=DIRECTION('',(1.,1.46081976924362E-16,0.));
#42869=DIRECTION('center_axis',(1.,1.92420077553238E-16,0.));
#42870=DIRECTION('ref_axis',(-1.92420077553238E-16,1.,0.));
#42871=DIRECTION('',(1.,1.46081976924362E-16,0.));
#42872=DIRECTION('center_axis',(1.,1.46081976924362E-16,0.));
#42873=DIRECTION('ref_axis',(-1.46081976924362E-16,1.,0.));
#42874=DIRECTION('center_axis',(1.,1.46081976924362E-16,0.));
#42875=DIRECTION('ref_axis',(-1.46081976924362E-16,1.,0.));
#42876=DIRECTION('',(1.,1.46081976924362E-16,0.));
#42877=DIRECTION('center_axis',(1.,1.92420077553238E-16,0.));
#42878=DIRECTION('ref_axis',(-1.92420077553238E-16,1.,0.));
#42879=DIRECTION('',(1.,1.46081976924362E-16,0.));
#42880=DIRECTION('center_axis',(1.,1.46081976924362E-16,0.));
#42881=DIRECTION('ref_axis',(-1.46081976924362E-16,1.,0.));
#42882=DIRECTION('center_axis',(1.,1.46081976924362E-16,0.));
#42883=DIRECTION('ref_axis',(-1.46081976924362E-16,1.,0.));
#42884=DIRECTION('',(1.,1.46081976924362E-16,0.));
#42885=DIRECTION('center_axis',(1.,1.92420077553238E-16,0.));
#42886=DIRECTION('ref_axis',(-1.92420077553238E-16,1.,0.));
#42887=DIRECTION('',(1.,1.46081976924362E-16,0.));
#42888=DIRECTION('center_axis',(1.,1.46081976924362E-16,0.));
#42889=DIRECTION('ref_axis',(-1.46081976924362E-16,1.,0.));
#42890=DIRECTION('center_axis',(-1.,-1.46081976924362E-16,0.));
#42891=DIRECTION('ref_axis',(-1.46081976924362E-16,1.,0.));
#42892=DIRECTION('',(1.,1.46081976924362E-16,0.));
#42893=DIRECTION('center_axis',(-1.,-1.92420077553238E-16,0.));
#42894=DIRECTION('ref_axis',(-1.92420077553238E-16,1.,0.));
#42895=DIRECTION('',(1.,1.46081976924362E-16,0.));
#42896=DIRECTION('center_axis',(1.,1.46081976924362E-16,0.));
#42897=DIRECTION('ref_axis',(-1.46081976924362E-16,1.,0.));
#42898=DIRECTION('center_axis',(-1.,-1.46081976924362E-16,0.));
#42899=DIRECTION('ref_axis',(-1.46081976924362E-16,1.,0.));
#42900=DIRECTION('',(1.,1.46081976924362E-16,0.));
#42901=DIRECTION('center_axis',(-1.,-1.92420077553238E-16,0.));
#42902=DIRECTION('ref_axis',(-1.92420077553238E-16,1.,0.));
#42903=DIRECTION('',(1.,1.46081976924362E-16,0.));
#42904=DIRECTION('center_axis',(1.,1.46081976924362E-16,0.));
#42905=DIRECTION('ref_axis',(-1.46081976924362E-16,1.,0.));
#42906=DIRECTION('center_axis',(1.,1.46081976924362E-16,0.));
#42907=DIRECTION('ref_axis',(-1.46081976924362E-16,1.,0.));
#42908=DIRECTION('',(1.,1.46081976924362E-16,0.));
#42909=DIRECTION('center_axis',(1.,1.92420077553238E-16,0.));
#42910=DIRECTION('ref_axis',(-1.92420077553238E-16,1.,0.));
#42911=DIRECTION('',(1.,1.46081976924362E-16,0.));
#42912=DIRECTION('center_axis',(1.,1.46081976924362E-16,0.));
#42913=DIRECTION('ref_axis',(-1.46081976924362E-16,1.,0.));
#42914=DIRECTION('center_axis',(-1.,-1.46081976924362E-16,0.));
#42915=DIRECTION('ref_axis',(-1.46081976924362E-16,1.,0.));
#42916=DIRECTION('',(1.,1.46081976924362E-16,0.));
#42917=DIRECTION('center_axis',(-1.,-1.92420077553238E-16,0.));
#42918=DIRECTION('ref_axis',(-1.92420077553238E-16,1.,0.));
#42919=DIRECTION('',(1.,1.46081976924362E-16,0.));
#42920=DIRECTION('center_axis',(1.,1.46081976924362E-16,0.));
#42921=DIRECTION('ref_axis',(-1.46081976924362E-16,1.,0.));
#42922=DIRECTION('center_axis',(1.,1.46081976924362E-16,0.));
#42923=DIRECTION('ref_axis',(-1.46081976924362E-16,1.,0.));
#42924=DIRECTION('',(1.,1.46081976924362E-16,0.));
#42925=DIRECTION('center_axis',(1.,1.92420077553238E-16,0.));
#42926=DIRECTION('ref_axis',(-1.92420077553238E-16,1.,0.));
#42927=DIRECTION('',(1.,1.46081976924362E-16,0.));
#42928=DIRECTION('center_axis',(1.,1.46081976924362E-16,0.));
#42929=DIRECTION('ref_axis',(-1.46081976924362E-16,1.,0.));
#42930=DIRECTION('center_axis',(1.,1.46081976924362E-16,0.));
#42931=DIRECTION('ref_axis',(-1.46081976924362E-16,1.,0.));
#42932=DIRECTION('',(1.,1.46081976924362E-16,0.));
#42933=DIRECTION('center_axis',(1.,1.92420077553238E-16,0.));
#42934=DIRECTION('ref_axis',(-1.92420077553238E-16,1.,0.));
#42935=DIRECTION('',(1.,1.46081976924362E-16,0.));
#42936=DIRECTION('center_axis',(1.,1.46081976924362E-16,0.));
#42937=DIRECTION('ref_axis',(-1.46081976924362E-16,1.,0.));
#42938=DIRECTION('center_axis',(-1.,-1.46081976924362E-16,0.));
#42939=DIRECTION('ref_axis',(-1.46081976924362E-16,1.,0.));
#42940=DIRECTION('',(1.,1.46081976924362E-16,0.));
#42941=DIRECTION('center_axis',(-1.,-1.92420077553238E-16,0.));
#42942=DIRECTION('ref_axis',(-1.92420077553238E-16,1.,0.));
#42943=DIRECTION('',(1.,1.46081976924362E-16,0.));
#42944=DIRECTION('center_axis',(-1.,-4.38245930773088E-16,0.));
#42945=DIRECTION('ref_axis',(4.38245930773088E-16,-1.,0.));
#42946=DIRECTION('center_axis',(-1.,-4.38245930773088E-16,0.));
#42947=DIRECTION('ref_axis',(4.38245930773088E-16,-1.,0.));
#42948=DIRECTION('',(1.,4.38245930773088E-16,0.));
#42949=DIRECTION('center_axis',(1.,4.38245930773088E-16,0.));
#42950=DIRECTION('ref_axis',(4.38245930773088E-16,-1.,-4.62592926927148E-15));
#42951=DIRECTION('',(-1.,-4.38245930773088E-16,0.));
#42952=DIRECTION('center_axis',(-1.,-4.38245930773088E-16,0.));
#42953=DIRECTION('ref_axis',(4.38245930773088E-16,-1.,0.));
#42954=DIRECTION('center_axis',(-1.,-4.38245930773088E-16,0.));
#42955=DIRECTION('ref_axis',(4.38245930773088E-16,-1.,0.));
#42956=DIRECTION('',(1.,4.38245930773088E-16,0.));
#42957=DIRECTION('center_axis',(1.,4.38245930773088E-16,0.));
#42958=DIRECTION('ref_axis',(4.38245930773088E-16,-1.,-4.62592926927148E-15));
#42959=DIRECTION('',(-1.,-4.38245930773088E-16,0.));
#42960=DIRECTION('center_axis',(-1.,-4.38245930773088E-16,0.));
#42961=DIRECTION('ref_axis',(4.38245930773088E-16,-1.,0.));
#42962=DIRECTION('center_axis',(-1.,-4.38245930773088E-16,0.));
#42963=DIRECTION('ref_axis',(4.38245930773088E-16,-1.,0.));
#42964=DIRECTION('',(1.,4.38245930773088E-16,0.));
#42965=DIRECTION('center_axis',(1.,4.38245930773088E-16,0.));
#42966=DIRECTION('ref_axis',(4.38245930773088E-16,-1.,-1.15648231731787E-14));
#42967=DIRECTION('',(-1.,-4.38245930773088E-16,0.));
#42968=DIRECTION('center_axis',(-1.,-4.38245930773088E-16,0.));
#42969=DIRECTION('ref_axis',(4.38245930773088E-16,-1.,0.));
#42970=DIRECTION('center_axis',(-1.,-4.38245930773088E-16,0.));
#42971=DIRECTION('ref_axis',(4.38245930773088E-16,-1.,0.));
#42972=DIRECTION('',(1.,4.38245930773088E-16,0.));
#42973=DIRECTION('center_axis',(1.,4.38245930773088E-16,0.));
#42974=DIRECTION('ref_axis',(4.38245930773088E-16,-1.,0.));
#42975=DIRECTION('',(-1.,-4.38245930773088E-16,0.));
#42976=DIRECTION('center_axis',(-1.,-4.38245930773088E-16,0.));
#42977=DIRECTION('ref_axis',(4.38245930773088E-16,-1.,0.));
#42978=DIRECTION('center_axis',(-1.,-4.38245930773088E-16,0.));
#42979=DIRECTION('ref_axis',(4.38245930773088E-16,-1.,0.));
#42980=DIRECTION('',(1.,4.38245930773088E-16,0.));
#42981=DIRECTION('center_axis',(1.,4.38245930773088E-16,0.));
#42982=DIRECTION('ref_axis',(4.38245930773088E-16,-1.,4.16333634234433E-14));
#42983=DIRECTION('',(-1.,-4.38245930773088E-16,-8.64002241377108E-33));
#42984=DIRECTION('center_axis',(-1.,-4.38245930773088E-16,0.));
#42985=DIRECTION('ref_axis',(4.38245930773088E-16,-1.,0.));
#42986=DIRECTION('center_axis',(-1.,-4.38245930773088E-16,0.));
#42987=DIRECTION('ref_axis',(4.38245930773088E-16,-1.,0.));
#42988=DIRECTION('',(1.,4.38245930773088E-16,0.));
#42989=DIRECTION('center_axis',(1.,4.38245930773088E-16,0.));
#42990=DIRECTION('ref_axis',(4.38245930773088E-16,-1.,-2.31296463463574E-15));
#42991=DIRECTION('',(-1.,-4.38245930773088E-16,0.));
#42992=DIRECTION('center_axis',(-1.,-4.38245930773088E-16,0.));
#42993=DIRECTION('ref_axis',(4.38245930773088E-16,-1.,0.));
#42994=DIRECTION('center_axis',(-1.,-4.38245930773088E-16,0.));
#42995=DIRECTION('ref_axis',(4.38245930773088E-16,-1.,0.));
#42996=DIRECTION('',(1.,4.38245930773088E-16,0.));
#42997=DIRECTION('center_axis',(1.,4.38245930773088E-16,0.));
#42998=DIRECTION('ref_axis',(4.38245930773088E-16,-1.,1.04083408558608E-14));
#42999=DIRECTION('',(-1.,-4.38245930773088E-16,0.));
#43000=DIRECTION('center_axis',(-1.,-4.38245930773088E-16,0.));
#43001=DIRECTION('ref_axis',(4.38245930773088E-16,-1.,0.));
#43002=DIRECTION('center_axis',(-1.,-4.38245930773088E-16,0.));
#43003=DIRECTION('ref_axis',(4.38245930773088E-16,-1.,0.));
#43004=DIRECTION('',(1.,4.38245930773088E-16,0.));
#43005=DIRECTION('center_axis',(1.,4.38245930773088E-16,0.));
#43006=DIRECTION('ref_axis',(4.38245930773088E-16,-1.,0.));
#43007=DIRECTION('',(-1.,-4.38245930773088E-16,0.));
#43008=DIRECTION('center_axis',(-1.,-4.38245930773088E-16,0.));
#43009=DIRECTION('ref_axis',(4.38245930773088E-16,-1.,0.));
#43010=DIRECTION('center_axis',(-1.,-4.38245930773088E-16,0.));
#43011=DIRECTION('ref_axis',(4.38245930773088E-16,-1.,0.));
#43012=DIRECTION('',(1.,4.38245930773088E-16,0.));
#43013=DIRECTION('center_axis',(1.,4.38245930773088E-16,0.));
#43014=DIRECTION('ref_axis',(4.38245930773088E-16,-1.,-1.61907524424502E-14));
#43015=DIRECTION('',(-1.,-4.38245930773088E-16,0.));
#43016=DIRECTION('center_axis',(-1.,-4.38245930773088E-16,0.));
#43017=DIRECTION('ref_axis',(4.38245930773088E-16,-1.,0.));
#43018=DIRECTION('center_axis',(-1.,-4.38245930773088E-16,0.));
#43019=DIRECTION('ref_axis',(4.38245930773088E-16,-1.,0.));
#43020=DIRECTION('',(1.,4.38245930773088E-16,0.));
#43021=DIRECTION('center_axis',(1.,4.38245930773088E-16,0.));
#43022=DIRECTION('ref_axis',(4.38245930773088E-16,-1.,0.));
#43023=DIRECTION('',(-1.,-4.38245930773088E-16,0.));
#43024=DIRECTION('center_axis',(-1.,-4.38245930773088E-16,0.));
#43025=DIRECTION('ref_axis',(4.38245930773088E-16,-1.,0.));
#43026=DIRECTION('center_axis',(-1.,-4.38245930773088E-16,0.));
#43027=DIRECTION('ref_axis',(4.38245930773088E-16,-1.,0.));
#43028=DIRECTION('',(1.,4.38245930773088E-16,0.));
#43029=DIRECTION('center_axis',(1.,4.38245930773088E-16,0.));
#43030=DIRECTION('ref_axis',(4.38245930773088E-16,-1.,-1.38777878078144E-14));
#43031=DIRECTION('',(-1.,-4.38245930773088E-16,-8.64002241377108E-33));
#43032=DIRECTION('center_axis',(-1.,-4.38245930773088E-16,0.));
#43033=DIRECTION('ref_axis',(4.38245930773088E-16,-1.,0.));
#43034=DIRECTION('center_axis',(-1.,-4.38245930773088E-16,0.));
#43035=DIRECTION('ref_axis',(4.38245930773088E-16,-1.,0.));
#43036=DIRECTION('',(1.,4.38245930773088E-16,0.));
#43037=DIRECTION('center_axis',(1.,4.38245930773088E-16,0.));
#43038=DIRECTION('ref_axis',(4.38245930773088E-16,-1.,1.73472347597681E-15));
#43039=DIRECTION('',(-1.,-4.38245930773088E-16,0.));
#43040=DIRECTION('center_axis',(-1.,-4.38245930773088E-16,0.));
#43041=DIRECTION('ref_axis',(4.38245930773088E-16,-1.,0.));
#43042=DIRECTION('center_axis',(-1.,-4.38245930773088E-16,0.));
#43043=DIRECTION('ref_axis',(4.38245930773088E-16,-1.,0.));
#43044=DIRECTION('',(1.,4.38245930773088E-16,0.));
#43045=DIRECTION('center_axis',(1.,4.38245930773088E-16,0.));
#43046=DIRECTION('ref_axis',(4.38245930773088E-16,-1.,-3.98986399474665E-14));
#43047=DIRECTION('',(-1.,-4.38245930773088E-16,0.));
#43048=DIRECTION('center_axis',(-1.,-4.38245930773088E-16,0.));
#43049=DIRECTION('ref_axis',(4.38245930773088E-16,-1.,0.));
#43050=DIRECTION('center_axis',(-1.,-4.38245930773088E-16,0.));
#43051=DIRECTION('ref_axis',(4.38245930773088E-16,-1.,0.));
#43052=DIRECTION('',(1.,4.38245930773088E-16,0.));
#43053=DIRECTION('center_axis',(1.,4.38245930773088E-16,0.));
#43054=DIRECTION('ref_axis',(4.38245930773088E-16,-1.,0.));
#43055=DIRECTION('',(-1.,-4.38245930773088E-16,0.));
#43056=DIRECTION('center_axis',(-1.,-4.38245930773088E-16,0.));
#43057=DIRECTION('ref_axis',(4.38245930773088E-16,-1.,0.));
#43058=DIRECTION('center_axis',(-1.,-4.38245930773088E-16,0.));
#43059=DIRECTION('ref_axis',(4.38245930773088E-16,-1.,0.));
#43060=DIRECTION('',(1.,4.38245930773088E-16,0.));
#43061=DIRECTION('center_axis',(1.,4.38245930773088E-16,0.));
#43062=DIRECTION('ref_axis',(4.38245930773088E-16,-1.,1.15648231731787E-15));
#43063=DIRECTION('',(-1.,-4.38245930773088E-16,0.));
#43064=DIRECTION('center_axis',(-1.,-4.38245930773088E-16,0.));
#43065=DIRECTION('ref_axis',(4.38245930773088E-16,-1.,0.));
#43066=DIRECTION('center_axis',(-1.,-4.38245930773088E-16,0.));
#43067=DIRECTION('ref_axis',(4.38245930773088E-16,-1.,0.));
#43068=DIRECTION('',(1.,4.38245930773088E-16,0.));
#43069=DIRECTION('center_axis',(1.,4.38245930773088E-16,0.));
#43070=DIRECTION('ref_axis',(4.38245930773088E-16,-1.,-2.31296463463574E-14));
#43071=DIRECTION('',(-1.,-4.38245930773088E-16,0.));
#43072=DIRECTION('center_axis',(-1.,-4.38245930773088E-16,0.));
#43073=DIRECTION('ref_axis',(4.38245930773088E-16,-1.,0.));
#43074=DIRECTION('center_axis',(-1.,-4.38245930773088E-16,0.));
#43075=DIRECTION('ref_axis',(4.38245930773088E-16,-1.,0.));
#43076=DIRECTION('',(1.,4.38245930773088E-16,0.));
#43077=DIRECTION('center_axis',(1.,4.38245930773088E-16,0.));
#43078=DIRECTION('ref_axis',(4.38245930773088E-16,-1.,0.));
#43079=DIRECTION('',(-1.,-4.38245930773088E-16,0.));
#43080=DIRECTION('center_axis',(-1.,-4.38245930773088E-16,0.));
#43081=DIRECTION('ref_axis',(4.38245930773088E-16,-1.,0.));
#43082=DIRECTION('center_axis',(-1.,-4.38245930773088E-16,0.));
#43083=DIRECTION('ref_axis',(4.38245930773088E-16,-1.,0.));
#43084=DIRECTION('',(1.,4.38245930773088E-16,0.));
#43085=DIRECTION('center_axis',(1.,4.38245930773088E-16,0.));
#43086=DIRECTION('ref_axis',(4.38245930773088E-16,-1.,-3.70074341541719E-14));
#43087=DIRECTION('',(-1.,-4.38245930773088E-16,-6.16297582203917E-33));
#43088=DIRECTION('',(-1.,-4.38245930773088E-16,0.));
#43089=DIRECTION('',(1.,4.38245930773088E-16,0.));
#43090=DIRECTION('',(-1.,-4.38245930773088E-16,0.));
#43091=DIRECTION('',(1.,4.38245930773088E-16,0.));
#43092=DIRECTION('',(-1.,-4.38245930773088E-16,0.));
#43093=DIRECTION('',(1.,4.38245930773088E-16,0.));
#43094=DIRECTION('',(-1.,-4.38245930773088E-16,0.));
#43095=DIRECTION('',(1.,4.38245930773088E-16,0.));
#43096=DIRECTION('',(-1.,-4.38245930773088E-16,0.));
#43097=DIRECTION('',(1.,4.38245930773088E-16,0.));
#43098=DIRECTION('center_axis',(-1.,-4.38245930773088E-16,0.));
#43099=DIRECTION('ref_axis',(4.38245930773088E-16,-1.,0.));
#43100=DIRECTION('center_axis',(1.,4.38245930773088E-16,0.));
#43101=DIRECTION('ref_axis',(4.38245930773088E-16,-1.,0.));
#43102=DIRECTION('',(-1.,-4.38245930773088E-16,0.));
#43103=DIRECTION('center_axis',(1.,4.81050193883094E-16,1.4791141972894E-31));
#43104=DIRECTION('ref_axis',(4.81050193883094E-16,-1.,7.11528171381301E-47));
#43105=DIRECTION('center_axis',(-1.,-4.38245930773088E-16,0.));
#43106=DIRECTION('ref_axis',(4.38245930773088E-16,-1.,0.));
#43107=DIRECTION('center_axis',(-1.,-4.38245930773088E-16,0.));
#43108=DIRECTION('ref_axis',(4.38245930773088E-16,-1.,0.));
#43109=DIRECTION('',(-1.,-4.38245930773088E-16,0.));
#43110=DIRECTION('center_axis',(-1.,-4.81050193883094E-16,-1.4791141972894E-31));
#43111=DIRECTION('ref_axis',(4.81050193883094E-16,-1.,7.11528171381301E-47));
#43112=DIRECTION('center_axis',(-1.,-4.38245930773088E-16,0.));
#43113=DIRECTION('ref_axis',(4.38245930773088E-16,-1.,0.));
#43114=DIRECTION('center_axis',(1.,4.38245930773088E-16,0.));
#43115=DIRECTION('ref_axis',(4.38245930773088E-16,-1.,0.));
#43116=DIRECTION('',(-1.,-4.38245930773088E-16,0.));
#43117=DIRECTION('center_axis',(1.,4.81050193883094E-16,1.4791141972894E-31));
#43118=DIRECTION('ref_axis',(4.81050193883094E-16,-1.,7.11528171381301E-47));
#43119=DIRECTION('center_axis',(-1.,-4.38245930773088E-16,0.));
#43120=DIRECTION('ref_axis',(4.38245930773088E-16,-1.,0.));
#43121=DIRECTION('center_axis',(-1.,-4.38245930773088E-16,0.));
#43122=DIRECTION('ref_axis',(4.38245930773088E-16,-1.,0.));
#43123=DIRECTION('',(-1.,-4.38245930773088E-16,0.));
#43124=DIRECTION('center_axis',(-1.,-4.81050193883094E-16,-1.4791141972894E-31));
#43125=DIRECTION('ref_axis',(4.81050193883094E-16,-1.,7.11528171381302E-47));
#43126=DIRECTION('center_axis',(-1.,-4.38245930773088E-16,0.));
#43127=DIRECTION('ref_axis',(0.,0.,1.));
#43128=DIRECTION('center_axis',(-1.,-4.38245930773088E-16,0.));
#43129=DIRECTION('ref_axis',(0.,0.,-1.));
#43130=DIRECTION('center_axis',(-4.38245930773088E-16,1.,-2.089831575765E-16));
#43131=DIRECTION('ref_axis',(0.,-2.089831575765E-16,-1.));
#43132=DIRECTION('center_axis',(-1.,-4.38245930773088E-16,0.));
#43133=DIRECTION('ref_axis',(0.,0.,1.));
#43134=DIRECTION('center_axis',(-1.,-4.38245930773088E-16,0.));
#43135=DIRECTION('ref_axis',(0.,0.,1.));
#43136=DIRECTION('center_axis',(-1.,-4.38245930773088E-16,0.));
#43137=DIRECTION('ref_axis',(4.38245930773088E-16,-1.,0.));
#43138=DIRECTION('center_axis',(-4.38245930773088E-16,1.,-1.9456480777872E-16));
#43139=DIRECTION('ref_axis',(0.,-1.9456480777872E-16,-1.));
#43140=DIRECTION('center_axis',(-1.,-4.38245930773088E-16,0.));
#43141=DIRECTION('ref_axis',(4.38245930773088E-16,-1.,0.));
#43142=DIRECTION('center_axis',(-1.,-4.38245930773088E-16,0.));
#43143=DIRECTION('ref_axis',(0.,0.,1.));
#43144=DIRECTION('center_axis',(-1.,-4.38245930773088E-16,0.));
#43145=DIRECTION('ref_axis',(4.38245930773088E-16,-1.,0.));
#43146=DIRECTION('center_axis',(4.38245930773088E-16,-1.,2.05122036882246E-16));
#43147=DIRECTION('ref_axis',(0.,-2.05122036882246E-16,-1.));
#43148=DIRECTION('center_axis',(-1.,-4.38245930773088E-16,0.));
#43149=DIRECTION('ref_axis',(0.,0.,1.));
#43150=DIRECTION('center_axis',(1.,4.38245930773088E-16,0.));
#43151=DIRECTION('ref_axis',(0.,0.,1.));
#43152=DIRECTION('center_axis',(4.38245930773088E-16,-1.,1.91213816259009E-16));
#43153=DIRECTION('ref_axis',(0.,-1.91213816259009E-16,-1.));
#43154=DIRECTION('center_axis',(0.,1.,0.));
#43155=DIRECTION('ref_axis',(0.,0.,1.));
#43156=DIRECTION('center_axis',(0.,-1.,0.));
#43157=DIRECTION('ref_axis',(0.,0.,1.));
#43158=DIRECTION('',(0.,1.,0.));
#43159=DIRECTION('center_axis',(0.,-1.,0.));
#43160=DIRECTION('ref_axis',(0.,0.,1.));
#43161=DIRECTION('center_axis',(0.,1.,0.));
#43162=DIRECTION('ref_axis',(0.,0.,1.));
#43163=DIRECTION('center_axis',(0.,-1.,0.));
#43164=DIRECTION('ref_axis',(0.,0.,1.));
#43165=DIRECTION('',(0.,1.,0.));
#43166=DIRECTION('center_axis',(0.,-1.,0.));
#43167=DIRECTION('ref_axis',(0.,0.,1.));
#43168=DIRECTION('center_axis',(0.,1.,0.));
#43169=DIRECTION('ref_axis',(0.,0.,1.));
#43170=DIRECTION('center_axis',(0.,-1.,0.));
#43171=DIRECTION('ref_axis',(0.,0.,1.));
#43172=DIRECTION('',(0.,1.,0.));
#43173=DIRECTION('center_axis',(0.,-1.,0.));
#43174=DIRECTION('ref_axis',(0.,0.,1.));
#43175=DIRECTION('center_axis',(0.,1.,0.));
#43176=DIRECTION('ref_axis',(0.,0.,1.));
#43177=DIRECTION('center_axis',(0.,-1.,0.));
#43178=DIRECTION('ref_axis',(0.,0.,1.));
#43179=DIRECTION('',(0.,1.,0.));
#43180=DIRECTION('center_axis',(0.,-1.,0.));
#43181=DIRECTION('ref_axis',(0.,0.,1.));
#43182=DIRECTION('',(-1.,-4.38245930773088E-16,0.));
#43183=DIRECTION('',(1.,4.38245930773088E-16,0.));
#43184=DIRECTION('center_axis',(0.,-1.,0.));
#43185=DIRECTION('ref_axis',(0.,0.,-1.));
#43186=DIRECTION('',(0.,-3.77113799125394E-15,1.));
#43187=DIRECTION('',(-1.,0.,0.));
#43188=DIRECTION('',(0.,0.,-1.));
#43189=DIRECTION('center_axis',(0.,1.,0.));
#43190=DIRECTION('ref_axis',(0.,0.,1.));
#43191=DIRECTION('',(0.,0.,-1.));
#43192=DIRECTION('center_axis',(0.,1.,0.));
#43193=DIRECTION('ref_axis',(0.,0.,-1.));
#43194=DIRECTION('',(0.,0.,-1.));
#43195=DIRECTION('',(-1.,0.,0.));
#43196=DIRECTION('',(0.,-1.41417674672023E-15,1.));
#43197=DIRECTION('',(-1.,0.,0.));
#43198=DIRECTION('',(0.,0.,-1.));
#43199=DIRECTION('',(-1.,0.,0.));
#43200=DIRECTION('',(0.,0.,1.));
#43201=DIRECTION('',(-1.,0.,0.));
#43202=DIRECTION('',(3.77113799125394E-15,1.41417674672023E-15,-1.));
#43203=DIRECTION('',(-1.,0.,0.));
#43204=DIRECTION('',(0.,0.,1.));
#43205=DIRECTION('center_axis',(0.,1.,0.));
#43206=DIRECTION('ref_axis',(0.,0.,1.));
#43207=DIRECTION('',(0.,0.,-1.));
#43208=DIRECTION('center_axis',(0.,1.,0.));
#43209=DIRECTION('ref_axis',(0.,0.,-1.));
#43210=DIRECTION('',(0.,0.,1.));
#43211=DIRECTION('',(-1.,0.,0.));
#43212=DIRECTION('',(-3.77113799125394E-15,3.77113799125394E-15,-1.));
#43213=DIRECTION('',(1.,0.,0.));
#43214=DIRECTION('',(0.,0.,1.));
#43215=DIRECTION('',(1.,0.,0.));
#43216=DIRECTION('',(0.,0.,-1.));
#43217=DIRECTION('',(1.,0.,0.));
#43218=DIRECTION('',(1.,0.,0.));
#43219=DIRECTION('',(-1.,0.,0.));
#43220=DIRECTION('',(1.,0.,0.));
#43221=DIRECTION('',(0.,0.,-1.));
#43222=DIRECTION('',(-1.,0.,0.));
#43223=DIRECTION('',(-1.,0.,0.));
#43224=DIRECTION('',(-1.,0.,0.));
#43225=DIRECTION('',(0.,0.,1.));
#43226=DIRECTION('',(1.,0.,0.));
#43227=DIRECTION('',(-1.,0.,0.));
#43228=DIRECTION('',(1.,0.,0.));
#43229=DIRECTION('',(0.,0.,-1.));
#43230=DIRECTION('',(-1.,0.,0.));
#43231=DIRECTION('',(-1.,0.,0.));
#43232=DIRECTION('',(-1.,0.,0.));
#43233=DIRECTION('',(0.,0.,1.));
#43234=DIRECTION('',(1.,0.,0.));
#43235=DIRECTION('',(-1.,0.,0.));
#43236=DIRECTION('',(1.,0.,0.));
#43237=DIRECTION('',(0.,0.,-1.));
#43238=DIRECTION('',(-1.,0.,0.));
#43239=DIRECTION('',(-1.,0.,0.));
#43240=DIRECTION('',(-1.,0.,0.));
#43241=DIRECTION('',(0.,0.,1.));
#43242=DIRECTION('',(1.,0.,0.));
#43243=DIRECTION('',(-1.,0.,0.));
#43244=DIRECTION('',(1.,0.,0.));
#43245=DIRECTION('',(0.,0.,-1.));
#43246=DIRECTION('',(-1.,0.,0.));
#43247=DIRECTION('',(-1.,0.,0.));
#43248=DIRECTION('',(-1.,0.,0.));
#43249=DIRECTION('',(0.,0.,1.));
#43250=DIRECTION('center_axis',(0.,-1.,0.));
#43251=DIRECTION('ref_axis',(0.,0.,-1.));
#43252=DIRECTION('',(-1.,0.,0.));
#43253=DIRECTION('',(0.,0.,1.));
#43254=DIRECTION('',(1.,0.,0.));
#43255=DIRECTION('',(0.,0.,-1.));
#43256=DIRECTION('',(1.,0.,0.));
#43257=DIRECTION('',(0.,0.,1.));
#43258=DIRECTION('',(1.,0.,0.));
#43259=DIRECTION('',(-3.77113799125394E-15,0.,-1.));
#43260=DIRECTION('',(-1.,0.,0.));
#43261=DIRECTION('',(0.,0.,-1.));
#43262=DIRECTION('center_axis',(0.,-1.,0.));
#43263=DIRECTION('ref_axis',(0.,0.,-1.));
#43264=DIRECTION('',(0.,0.,-1.));
#43265=DIRECTION('center_axis',(0.,-1.,0.));
#43266=DIRECTION('ref_axis',(0.,0.,-1.));
#43267=DIRECTION('',(0.,0.,-1.));
#43268=DIRECTION('',(-1.,0.,0.));
#43269=DIRECTION('',(3.77113799125394E-15,0.,-1.));
#43270=DIRECTION('',(-1.,0.,0.));
#43271=DIRECTION('',(0.,0.,1.));
#43272=DIRECTION('',(-1.,0.,0.));
#43273=DIRECTION('',(0.,0.,-1.));
#43274=DIRECTION('',(-1.,0.,0.));
#43275=DIRECTION('',(0.,0.,1.));
#43276=DIRECTION('',(-1.,0.,0.));
#43277=DIRECTION('',(0.,0.,1.));
#43278=DIRECTION('center_axis',(0.,-1.,0.));
#43279=DIRECTION('ref_axis',(0.,0.,-1.));
#43280=DIRECTION('',(0.,0.,-1.));
#43281=DIRECTION('center_axis',(0.,-1.,0.));
#43282=DIRECTION('ref_axis',(0.,0.,-1.));
#43283=DIRECTION('',(0.,0.,1.));
#43284=DIRECTION('',(1.,0.,0.));
#43285=DIRECTION('',(0.,0.,-1.));
#43286=DIRECTION('',(1.,0.,0.));
#43287=DIRECTION('',(0.,0.,1.));
#43288=DIRECTION('',(1.,0.,0.));
#43289=DIRECTION('',(0.,0.,-1.));
#43290=DIRECTION('',(1.,0.,0.));
#43291=DIRECTION('',(0.,0.,1.));
#43292=DIRECTION('',(1.,0.,0.));
#43293=DIRECTION('',(0.,0.,-1.));
#43294=DIRECTION('',(1.,0.,0.));
#43295=DIRECTION('',(0.,0.,1.));
#43296=DIRECTION('',(1.,0.,0.));
#43297=DIRECTION('',(0.,0.,-1.));
#43298=DIRECTION('',(1.,0.,0.));
#43299=DIRECTION('',(0.,0.,1.));
#43300=DIRECTION('center_axis',(0.,0.,-1.));
#43301=DIRECTION('ref_axis',(-1.,0.,0.));
#43302=DIRECTION('',(0.,-1.,6.12323399573677E-17));
#43303=DIRECTION('',(0.,-1.,0.));
#43304=DIRECTION('center_axis',(0.,0.,-1.));
#43305=DIRECTION('ref_axis',(-1.,0.,0.));
#43306=DIRECTION('',(0.,-1.,6.12323399573677E-17));
#43307=DIRECTION('',(0.,1.,0.));
#43308=DIRECTION('center_axis',(0.,0.,-1.));
#43309=DIRECTION('ref_axis',(-1.,0.,0.));
#43310=DIRECTION('',(-1.15648231731787E-15,1.,0.));
#43311=DIRECTION('',(1.,0.,0.));
#43312=DIRECTION('',(0.,-1.,0.));
#43313=DIRECTION('center_axis',(0.,0.,1.));
#43314=DIRECTION('ref_axis',(-1.,1.06251812903579E-14,0.));
#43315=DIRECTION('',(-1.,-3.56237856673809E-16,0.));
#43316=DIRECTION('center_axis',(0.,0.,1.));
#43317=DIRECTION('ref_axis',(-1.,8.67361737988403E-16,0.));
#43318=DIRECTION('',(0.,-1.,0.));
#43319=DIRECTION('',(1.,0.,0.));
#43320=DIRECTION('',(-1.,0.,0.));
#43321=DIRECTION('',(1.,0.,0.));
#43322=DIRECTION('',(0.,1.,0.));
#43323=DIRECTION('',(-1.,0.,0.));
#43324=DIRECTION('',(-1.,0.,0.));
#43325=DIRECTION('',(-1.,0.,0.));
#43326=DIRECTION('',(-5.8432790769745E-16,1.,0.));
#43327=DIRECTION('',(1.,5.8432790769745E-16,0.));
#43328=DIRECTION('',(-1.,-5.8432790769745E-16,0.));
#43329=DIRECTION('',(1.,5.8432790769745E-16,0.));
#43330=DIRECTION('',(5.8432790769745E-16,-1.,0.));
#43331=DIRECTION('',(-1.,-5.8432790769745E-16,0.));
#43332=DIRECTION('',(-1.,-5.8432790769745E-16,0.));
#43333=DIRECTION('',(-1.,-5.8432790769745E-16,0.));
#43334=DIRECTION('center_axis',(0.,0.,-1.));
#43335=DIRECTION('ref_axis',(-1.,0.,0.));
#43336=DIRECTION('',(-1.,0.,0.));
#43337=DIRECTION('',(-1.15648231731787E-15,1.,0.));
#43338=DIRECTION('center_axis',(0.,0.,1.));
#43339=DIRECTION('ref_axis',(-1.,8.67361737988403E-16,0.));
#43340=DIRECTION('',(-1.,-3.56237856673809E-16,0.));
#43341=DIRECTION('center_axis',(0.,0.,1.));
#43342=DIRECTION('ref_axis',(-1.,1.06251812903579E-14,0.));
#43343=DIRECTION('',(0.,-1.,0.));
#43344=DIRECTION('',(-1.,0.,0.));
#43345=DIRECTION('',(0.,1.,0.));
#43346=DIRECTION('',(-1.,0.,0.));
#43347=DIRECTION('',(0.,-1.,0.));
#43348=DIRECTION('',(-5.8432790769745E-16,1.,0.));
#43349=DIRECTION('',(1.,5.8432790769745E-16,0.));
#43350=DIRECTION('',(5.8432790769745E-16,-1.,0.));
#43351=DIRECTION('',(1.,5.8432790769745E-16,0.));
#43352=DIRECTION('center_axis',(0.,0.,1.));
#43353=DIRECTION('ref_axis',(1.,0.,0.));
#43354=DIRECTION('',(0.,-1.,6.12323399573677E-17));
#43355=DIRECTION('',(0.,-1.,0.));
#43356=DIRECTION('center_axis',(0.,0.,1.));
#43357=DIRECTION('ref_axis',(1.,0.,0.));
#43358=DIRECTION('',(0.,-1.,6.12323399573677E-17));
#43359=DIRECTION('',(0.,1.,0.));
#43360=DIRECTION('center_axis',(1.,1.46081976924362E-16,0.));
#43361=DIRECTION('ref_axis',(-1.46081976924362E-16,1.,0.));
#43362=DIRECTION('',(1.46081976924362E-16,-1.,0.));
#43363=DIRECTION('',(-1.03295556492353E-16,0.707106781186547,0.707106781186547));
#43364=DIRECTION('',(0.,0.,-1.));
#43365=DIRECTION('',(1.03295556492353E-16,-0.707106781186547,0.707106781186547));
#43366=DIRECTION('',(1.46081976924362E-16,-1.,0.));
#43367=DIRECTION('',(0.,0.,1.));
#43368=DIRECTION('center_axis',(1.,1.46081976924362E-16,0.));
#43369=DIRECTION('ref_axis',(-1.46081976924362E-16,1.,0.));
#43370=DIRECTION('',(0.,0.,-1.));
#43371=DIRECTION('center_axis',(1.,1.46081976924362E-16,0.));
#43372=DIRECTION('ref_axis',(-1.46081976924362E-16,1.,0.));
#43373=DIRECTION('',(0.,0.,1.));
#43374=DIRECTION('',(-1.92420077553238E-16,1.,0.));
#43375=DIRECTION('',(-1.92420077553238E-16,1.,0.));
#43376=DIRECTION('center_axis',(-1.,-1.92420077553238E-16,0.));
#43377=DIRECTION('ref_axis',(-1.92420077553238E-16,1.,0.));
#43378=DIRECTION('',(-1.92420077553238E-16,1.,0.));
#43379=DIRECTION('',(-1.92420077553238E-16,1.,0.));
#43380=DIRECTION('center_axis',(-1.,-1.92420077553238E-16,0.));
#43381=DIRECTION('ref_axis',(-1.92420077553238E-16,1.,0.));
#43382=DIRECTION('',(-1.92420077553238E-16,1.,0.));
#43383=DIRECTION('',(-1.92420077553238E-16,1.,0.));
#43384=DIRECTION('center_axis',(-1.,-1.92420077553238E-16,0.));
#43385=DIRECTION('ref_axis',(-1.92420077553238E-16,1.,0.));
#43386=DIRECTION('',(-1.92420077553238E-16,1.,0.));
#43387=DIRECTION('',(-1.92420077553238E-16,1.,0.));
#43388=DIRECTION('center_axis',(-1.,-1.92420077553238E-16,0.));
#43389=DIRECTION('ref_axis',(-1.92420077553238E-16,1.,0.));
#43390=DIRECTION('',(-1.92420077553238E-16,1.,0.));
#43391=DIRECTION('',(-1.92420077553238E-16,1.,0.));
#43392=DIRECTION('center_axis',(-1.,-1.92420077553238E-16,0.));
#43393=DIRECTION('ref_axis',(-1.92420077553238E-16,1.,0.));
#43394=DIRECTION('',(-1.92420077553238E-16,1.,0.));
#43395=DIRECTION('',(-1.92420077553238E-16,1.,0.));
#43396=DIRECTION('center_axis',(-1.,-1.92420077553238E-16,0.));
#43397=DIRECTION('ref_axis',(-1.92420077553238E-16,1.,0.));
#43398=DIRECTION('',(-1.92420077553238E-16,1.,0.));
#43399=DIRECTION('',(-1.92420077553238E-16,1.,0.));
#43400=DIRECTION('center_axis',(-1.,-1.92420077553238E-16,0.));
#43401=DIRECTION('ref_axis',(-1.92420077553238E-16,1.,0.));
#43402=DIRECTION('',(-1.92420077553238E-16,1.,0.));
#43403=DIRECTION('',(-1.92420077553238E-16,1.,0.));
#43404=DIRECTION('center_axis',(-1.,-1.92420077553238E-16,0.));
#43405=DIRECTION('ref_axis',(-1.92420077553238E-16,1.,0.));
#43406=DIRECTION('',(-1.92420077553238E-16,1.,0.));
#43407=DIRECTION('',(-1.92420077553238E-16,1.,0.));
#43408=DIRECTION('center_axis',(-1.,-1.92420077553238E-16,0.));
#43409=DIRECTION('ref_axis',(-1.92420077553238E-16,1.,0.));
#43410=DIRECTION('',(-1.92420077553238E-16,1.,0.));
#43411=DIRECTION('',(-1.92420077553238E-16,1.,0.));
#43412=DIRECTION('center_axis',(-1.,-1.92420077553238E-16,0.));
#43413=DIRECTION('ref_axis',(-1.92420077553238E-16,1.,0.));
#43414=DIRECTION('',(-1.92420077553238E-16,1.,0.));
#43415=DIRECTION('',(-1.92420077553238E-16,1.,0.));
#43416=DIRECTION('center_axis',(-1.,-1.92420077553238E-16,0.));
#43417=DIRECTION('ref_axis',(-1.92420077553238E-16,1.,0.));
#43418=DIRECTION('',(-1.92420077553238E-16,1.,0.));
#43419=DIRECTION('',(-1.92420077553238E-16,1.,0.));
#43420=DIRECTION('center_axis',(-1.,-1.92420077553238E-16,0.));
#43421=DIRECTION('ref_axis',(-1.92420077553238E-16,1.,0.));
#43422=DIRECTION('',(1.92420077553238E-16,-1.,0.));
#43423=DIRECTION('center_axis',(-1.,-1.92420077553238E-16,0.));
#43424=DIRECTION('ref_axis',(-1.92420077553238E-16,1.,0.));
#43425=DIRECTION('',(1.92420077553238E-16,-1.,0.));
#43426=DIRECTION('',(1.92420077553238E-16,-1.,0.));
#43427=DIRECTION('center_axis',(-1.,-1.92420077553238E-16,0.));
#43428=DIRECTION('ref_axis',(-1.92420077553238E-16,1.,0.));
#43429=DIRECTION('',(1.92420077553238E-16,-1.,0.));
#43430=DIRECTION('',(1.92420077553238E-16,-1.,0.));
#43431=DIRECTION('center_axis',(-1.,-1.92420077553238E-16,0.));
#43432=DIRECTION('ref_axis',(-1.92420077553238E-16,1.,0.));
#43433=DIRECTION('',(1.92420077553238E-16,-1.,0.));
#43434=DIRECTION('',(1.92420077553238E-16,-1.,0.));
#43435=DIRECTION('center_axis',(-1.,-1.92420077553238E-16,0.));
#43436=DIRECTION('ref_axis',(-1.92420077553238E-16,1.,0.));
#43437=DIRECTION('',(1.92420077553238E-16,-1.,0.));
#43438=DIRECTION('',(1.92420077553238E-16,-1.,0.));
#43439=DIRECTION('center_axis',(-1.,-1.92420077553238E-16,0.));
#43440=DIRECTION('ref_axis',(-1.92420077553238E-16,1.,0.));
#43441=DIRECTION('',(1.92420077553238E-16,-1.,0.));
#43442=DIRECTION('',(1.92420077553238E-16,-1.,0.));
#43443=DIRECTION('center_axis',(-1.,-1.92420077553238E-16,0.));
#43444=DIRECTION('ref_axis',(-1.92420077553238E-16,1.,0.));
#43445=DIRECTION('',(1.92420077553238E-16,-1.,0.));
#43446=DIRECTION('',(1.92420077553238E-16,-1.,0.));
#43447=DIRECTION('center_axis',(-1.,-1.92420077553238E-16,0.));
#43448=DIRECTION('ref_axis',(-1.92420077553238E-16,1.,0.));
#43449=DIRECTION('',(1.92420077553238E-16,-1.,0.));
#43450=DIRECTION('',(1.92420077553238E-16,-1.,0.));
#43451=DIRECTION('center_axis',(-1.,-1.92420077553238E-16,0.));
#43452=DIRECTION('ref_axis',(-1.92420077553238E-16,1.,0.));
#43453=DIRECTION('',(1.92420077553238E-16,-1.,0.));
#43454=DIRECTION('',(1.92420077553238E-16,-1.,0.));
#43455=DIRECTION('center_axis',(-1.,-1.92420077553238E-16,0.));
#43456=DIRECTION('ref_axis',(-1.92420077553238E-16,1.,0.));
#43457=DIRECTION('',(1.92420077553238E-16,-1.,0.));
#43458=DIRECTION('',(1.92420077553238E-16,-1.,0.));
#43459=DIRECTION('center_axis',(-1.,-1.92420077553238E-16,0.));
#43460=DIRECTION('ref_axis',(-1.92420077553238E-16,1.,0.));
#43461=DIRECTION('',(1.92420077553238E-16,-1.,0.));
#43462=DIRECTION('',(1.92420077553238E-16,-1.,0.));
#43463=DIRECTION('center_axis',(-1.,-1.92420077553238E-16,0.));
#43464=DIRECTION('ref_axis',(-1.92420077553238E-16,1.,0.));
#43465=DIRECTION('',(1.92420077553238E-16,-1.,0.));
#43466=DIRECTION('',(1.92420077553238E-16,-1.,0.));
#43467=DIRECTION('center_axis',(-1.,-1.92420077553238E-16,0.));
#43468=DIRECTION('ref_axis',(-1.92420077553238E-16,1.,0.));
#43469=DIRECTION('',(1.92420077553238E-16,-1.,0.));
#43470=DIRECTION('',(-1.92420077553238E-16,1.,0.));
#43471=DIRECTION('center_axis',(1.,1.92420077553238E-16,0.));
#43472=DIRECTION('ref_axis',(-1.92420077553238E-16,1.,0.));
#43473=DIRECTION('',(-1.92420077553238E-16,1.,0.));
#43474=DIRECTION('',(-1.92420077553238E-16,1.,0.));
#43475=DIRECTION('center_axis',(1.,1.92420077553238E-16,0.));
#43476=DIRECTION('ref_axis',(-1.92420077553238E-16,1.,0.));
#43477=DIRECTION('',(-1.92420077553238E-16,1.,0.));
#43478=DIRECTION('',(-1.92420077553238E-16,1.,0.));
#43479=DIRECTION('center_axis',(1.,1.92420077553238E-16,0.));
#43480=DIRECTION('ref_axis',(-1.92420077553238E-16,1.,0.));
#43481=DIRECTION('',(-1.92420077553238E-16,1.,0.));
#43482=DIRECTION('',(-1.92420077553238E-16,1.,0.));
#43483=DIRECTION('center_axis',(1.,1.92420077553238E-16,0.));
#43484=DIRECTION('ref_axis',(-1.92420077553238E-16,1.,0.));
#43485=DIRECTION('',(-1.92420077553238E-16,1.,0.));
#43486=DIRECTION('',(-1.92420077553238E-16,1.,0.));
#43487=DIRECTION('center_axis',(1.,1.92420077553238E-16,0.));
#43488=DIRECTION('ref_axis',(-1.92420077553238E-16,1.,0.));
#43489=DIRECTION('',(-1.92420077553238E-16,1.,0.));
#43490=DIRECTION('',(-1.92420077553238E-16,1.,0.));
#43491=DIRECTION('center_axis',(1.,1.92420077553238E-16,0.));
#43492=DIRECTION('ref_axis',(-1.92420077553238E-16,1.,0.));
#43493=DIRECTION('',(-1.92420077553238E-16,1.,0.));
#43494=DIRECTION('',(-1.92420077553238E-16,1.,0.));
#43495=DIRECTION('center_axis',(1.,1.92420077553238E-16,0.));
#43496=DIRECTION('ref_axis',(-1.92420077553238E-16,1.,0.));
#43497=DIRECTION('',(-1.92420077553238E-16,1.,0.));
#43498=DIRECTION('',(-1.92420077553238E-16,1.,0.));
#43499=DIRECTION('center_axis',(1.,1.92420077553238E-16,0.));
#43500=DIRECTION('ref_axis',(-1.92420077553238E-16,1.,0.));
#43501=DIRECTION('',(-1.92420077553238E-16,1.,0.));
#43502=DIRECTION('',(-1.92420077553238E-16,1.,0.));
#43503=DIRECTION('center_axis',(1.,1.92420077553238E-16,0.));
#43504=DIRECTION('ref_axis',(-1.92420077553238E-16,1.,0.));
#43505=DIRECTION('',(-1.92420077553238E-16,1.,0.));
#43506=DIRECTION('',(-1.92420077553238E-16,1.,0.));
#43507=DIRECTION('center_axis',(1.,1.92420077553238E-16,0.));
#43508=DIRECTION('ref_axis',(-1.92420077553238E-16,1.,0.));
#43509=DIRECTION('',(-1.92420077553238E-16,1.,0.));
#43510=DIRECTION('',(-1.92420077553238E-16,1.,0.));
#43511=DIRECTION('center_axis',(1.,1.92420077553238E-16,0.));
#43512=DIRECTION('ref_axis',(-1.92420077553238E-16,1.,0.));
#43513=DIRECTION('',(-1.92420077553238E-16,1.,0.));
#43514=DIRECTION('',(-1.92420077553238E-16,1.,0.));
#43515=DIRECTION('center_axis',(1.,1.92420077553238E-16,0.));
#43516=DIRECTION('ref_axis',(-1.92420077553238E-16,1.,0.));
#43517=DIRECTION('',(-1.92420077553238E-16,1.,0.));
#43518=DIRECTION('',(1.92420077553238E-16,-1.,0.));
#43519=DIRECTION('',(1.92420077553238E-16,-1.,0.));
#43520=DIRECTION('center_axis',(1.,1.92420077553238E-16,0.));
#43521=DIRECTION('ref_axis',(-1.92420077553238E-16,1.,0.));
#43522=DIRECTION('',(1.92420077553238E-16,-1.,0.));
#43523=DIRECTION('',(1.92420077553238E-16,-1.,0.));
#43524=DIRECTION('center_axis',(1.,1.92420077553238E-16,0.));
#43525=DIRECTION('ref_axis',(-1.92420077553238E-16,1.,0.));
#43526=DIRECTION('',(1.92420077553238E-16,-1.,0.));
#43527=DIRECTION('',(1.92420077553238E-16,-1.,0.));
#43528=DIRECTION('center_axis',(1.,1.92420077553238E-16,0.));
#43529=DIRECTION('ref_axis',(-1.92420077553238E-16,1.,0.));
#43530=DIRECTION('',(1.92420077553238E-16,-1.,0.));
#43531=DIRECTION('',(1.92420077553238E-16,-1.,0.));
#43532=DIRECTION('center_axis',(1.,1.92420077553238E-16,0.));
#43533=DIRECTION('ref_axis',(-1.92420077553238E-16,1.,0.));
#43534=DIRECTION('',(1.92420077553238E-16,-1.,0.));
#43535=DIRECTION('',(1.92420077553238E-16,-1.,0.));
#43536=DIRECTION('center_axis',(1.,1.92420077553238E-16,0.));
#43537=DIRECTION('ref_axis',(-1.92420077553238E-16,1.,0.));
#43538=DIRECTION('',(1.92420077553238E-16,-1.,0.));
#43539=DIRECTION('',(1.92420077553238E-16,-1.,0.));
#43540=DIRECTION('center_axis',(1.,1.92420077553238E-16,0.));
#43541=DIRECTION('ref_axis',(-1.92420077553238E-16,1.,0.));
#43542=DIRECTION('',(1.92420077553238E-16,-1.,0.));
#43543=DIRECTION('',(1.92420077553238E-16,-1.,0.));
#43544=DIRECTION('center_axis',(1.,1.92420077553238E-16,0.));
#43545=DIRECTION('ref_axis',(-1.92420077553238E-16,1.,0.));
#43546=DIRECTION('',(1.92420077553238E-16,-1.,0.));
#43547=DIRECTION('',(1.92420077553238E-16,-1.,0.));
#43548=DIRECTION('center_axis',(1.,1.92420077553238E-16,0.));
#43549=DIRECTION('ref_axis',(-1.92420077553238E-16,1.,0.));
#43550=DIRECTION('',(1.92420077553238E-16,-1.,0.));
#43551=DIRECTION('',(1.92420077553238E-16,-1.,0.));
#43552=DIRECTION('center_axis',(1.,1.92420077553238E-16,0.));
#43553=DIRECTION('ref_axis',(-1.92420077553238E-16,1.,0.));
#43554=DIRECTION('',(1.92420077553238E-16,-1.,0.));
#43555=DIRECTION('',(1.92420077553238E-16,-1.,0.));
#43556=DIRECTION('center_axis',(1.,1.92420077553238E-16,0.));
#43557=DIRECTION('ref_axis',(-1.92420077553238E-16,1.,0.));
#43558=DIRECTION('',(1.92420077553238E-16,-1.,0.));
#43559=DIRECTION('',(1.92420077553238E-16,-1.,0.));
#43560=DIRECTION('center_axis',(1.,1.92420077553238E-16,0.));
#43561=DIRECTION('ref_axis',(-1.92420077553238E-16,1.,0.));
#43562=DIRECTION('',(1.92420077553238E-16,-1.,0.));
#43563=DIRECTION('',(1.92420077553238E-16,-1.,0.));
#43564=DIRECTION('center_axis',(1.,1.92420077553238E-16,0.));
#43565=DIRECTION('ref_axis',(-1.92420077553238E-16,1.,0.));
#43566=DIRECTION('center_axis',(1.,1.46081976924362E-16,0.));
#43567=DIRECTION('ref_axis',(-1.46081976924362E-16,1.,0.));
#43568=DIRECTION('',(0.,0.,-1.));
#43569=DIRECTION('',(1.03295556492353E-16,-0.707106781186547,-0.707106781186547));
#43570=DIRECTION('',(1.46081976924362E-16,-1.,0.));
#43571=DIRECTION('',(0.,0.,-1.));
#43572=DIRECTION('center_axis',(1.,1.46081976924362E-16,0.));
#43573=DIRECTION('ref_axis',(-1.46081976924362E-16,1.,0.));
#43574=DIRECTION('',(0.,0.,-1.));
#43575=DIRECTION('center_axis',(-1.,-8.82055185704388E-15,0.));
#43576=DIRECTION('ref_axis',(0.,0.,1.));
#43577=DIRECTION('',(0.,0.,-1.));
#43578=DIRECTION('',(1.46081976924362E-16,-1.,0.));
#43579=DIRECTION('',(-1.03295556492353E-16,0.707106781186547,-0.707106781186547));
#43580=DIRECTION('',(1.46081976924362E-16,-1.,0.));
#43581=DIRECTION('center_axis',(1.,1.46081976924362E-16,0.));
#43582=DIRECTION('ref_axis',(-1.46081976924362E-16,1.,0.));
#43583=DIRECTION('',(1.46081976924362E-16,-1.,0.));
#43584=DIRECTION('',(1.46081976924362E-16,-1.,0.));
#43585=DIRECTION('center_axis',(1.,1.46081976924362E-16,0.));
#43586=DIRECTION('ref_axis',(-1.46081976924362E-16,1.,0.));
#43587=DIRECTION('',(1.46081976924362E-16,-1.,0.));
#43588=DIRECTION('',(-1.46081976924362E-16,1.,0.));
#43589=DIRECTION('center_axis',(-1.,-1.46081976924362E-16,0.));
#43590=DIRECTION('ref_axis',(-1.46081976924362E-16,1.,0.));
#43591=DIRECTION('',(-1.46081976924362E-16,1.,0.));
#43592=DIRECTION('',(-1.46081976924362E-16,1.,0.));
#43593=DIRECTION('center_axis',(-1.,-1.46081976924362E-16,0.));
#43594=DIRECTION('ref_axis',(-1.46081976924362E-16,1.,0.));
#43595=DIRECTION('',(-1.46081976924362E-16,1.,0.));
#43596=DIRECTION('',(-1.46081976924362E-16,1.,0.));
#43597=DIRECTION('center_axis',(-1.,-1.46081976924362E-16,0.));
#43598=DIRECTION('ref_axis',(-1.46081976924362E-16,1.,0.));
#43599=DIRECTION('',(-1.46081976924362E-16,1.,0.));
#43600=DIRECTION('',(-1.46081976924362E-16,1.,0.));
#43601=DIRECTION('center_axis',(-1.,-1.46081976924362E-16,0.));
#43602=DIRECTION('ref_axis',(-1.46081976924362E-16,1.,0.));
#43603=DIRECTION('',(-1.46081976924362E-16,1.,0.));
#43604=DIRECTION('',(-1.46081976924362E-16,1.,0.));
#43605=DIRECTION('center_axis',(-1.,-1.46081976924362E-16,0.));
#43606=DIRECTION('ref_axis',(-1.46081976924362E-16,1.,0.));
#43607=DIRECTION('',(-1.46081976924362E-16,1.,0.));
#43608=DIRECTION('',(1.46081976924362E-16,-1.,0.));
#43609=DIRECTION('center_axis',(1.,1.46081976924362E-16,0.));
#43610=DIRECTION('ref_axis',(-1.46081976924362E-16,1.,0.));
#43611=DIRECTION('',(1.46081976924362E-16,-1.,0.));
#43612=DIRECTION('',(1.46081976924362E-16,-1.,0.));
#43613=DIRECTION('center_axis',(1.,1.46081976924362E-16,0.));
#43614=DIRECTION('ref_axis',(-1.46081976924362E-16,1.,0.));
#43615=DIRECTION('',(1.46081976924362E-16,-1.,0.));
#43616=DIRECTION('',(1.46081976924362E-16,-1.,0.));
#43617=DIRECTION('center_axis',(1.,1.46081976924362E-16,0.));
#43618=DIRECTION('ref_axis',(-1.46081976924362E-16,1.,0.));
#43619=DIRECTION('',(1.46081976924362E-16,-1.,0.));
#43620=DIRECTION('',(1.46081976924362E-16,-1.,0.));
#43621=DIRECTION('center_axis',(1.,1.46081976924362E-16,0.));
#43622=DIRECTION('ref_axis',(-1.46081976924362E-16,1.,0.));
#43623=DIRECTION('',(1.46081976924362E-16,-1.,0.));
#43624=DIRECTION('',(1.46081976924362E-16,-1.,0.));
#43625=DIRECTION('center_axis',(1.,1.46081976924362E-16,0.));
#43626=DIRECTION('ref_axis',(-1.46081976924362E-16,1.,0.));
#43627=DIRECTION('',(1.46081976924362E-16,-1.,0.));
#43628=DIRECTION('',(-1.46081976924362E-16,1.,0.));
#43629=DIRECTION('center_axis',(-1.,-1.46081976924362E-16,0.));
#43630=DIRECTION('ref_axis',(-1.46081976924362E-16,1.,0.));
#43631=DIRECTION('',(-1.46081976924362E-16,1.,0.));
#43632=DIRECTION('',(1.46081976924362E-16,-1.,0.));
#43633=DIRECTION('',(1.46081976924362E-16,-1.,0.));
#43634=DIRECTION('center_axis',(-1.,-1.46081976924362E-16,0.));
#43635=DIRECTION('ref_axis',(-1.46081976924362E-16,1.,0.));
#43636=DIRECTION('',(-1.46081976924362E-16,1.,0.));
#43637=DIRECTION('',(-1.46081976924362E-16,1.,0.));
#43638=DIRECTION('center_axis',(1.,1.46081976924362E-16,0.));
#43639=DIRECTION('ref_axis',(-1.46081976924362E-16,1.,0.));
#43640=DIRECTION('',(-1.46081976924362E-16,1.,0.));
#43641=DIRECTION('',(-1.46081976924362E-16,1.,0.));
#43642=DIRECTION('center_axis',(1.,1.46081976924362E-16,0.));
#43643=DIRECTION('ref_axis',(-1.46081976924362E-16,1.,0.));
#43644=DIRECTION('',(1.46081976924362E-16,-1.,0.));
#43645=DIRECTION('',(1.46081976924362E-16,-1.,0.));
#43646=DIRECTION('center_axis',(-1.,-1.46081976924362E-16,0.));
#43647=DIRECTION('ref_axis',(-1.46081976924362E-16,1.,0.));
#43648=DIRECTION('',(1.46081976924362E-16,-1.,0.));
#43649=DIRECTION('',(1.46081976924362E-16,-1.,0.));
#43650=DIRECTION('center_axis',(-1.,-1.46081976924362E-16,0.));
#43651=DIRECTION('ref_axis',(-1.46081976924362E-16,1.,0.));
#43652=DIRECTION('',(-1.46081976924362E-16,1.,0.));
#43653=DIRECTION('',(-1.46081976924362E-16,1.,0.));
#43654=DIRECTION('center_axis',(1.,1.46081976924362E-16,0.));
#43655=DIRECTION('ref_axis',(-1.46081976924362E-16,1.,0.));
#43656=DIRECTION('',(-1.46081976924362E-16,1.,0.));
#43657=DIRECTION('',(-1.46081976924362E-16,1.,0.));
#43658=DIRECTION('center_axis',(1.,1.46081976924362E-16,0.));
#43659=DIRECTION('ref_axis',(-1.46081976924362E-16,1.,0.));
#43660=DIRECTION('',(-1.46081976924362E-16,1.,0.));
#43661=DIRECTION('',(-1.46081976924362E-16,1.,0.));
#43662=DIRECTION('center_axis',(1.,1.46081976924362E-16,0.));
#43663=DIRECTION('ref_axis',(-1.46081976924362E-16,1.,0.));
#43664=DIRECTION('',(-1.46081976924362E-16,1.,0.));
#43665=DIRECTION('',(-1.46081976924362E-16,1.,0.));
#43666=DIRECTION('center_axis',(1.,1.46081976924362E-16,0.));
#43667=DIRECTION('ref_axis',(-1.46081976924362E-16,1.,0.));
#43668=DIRECTION('',(-1.46081976924362E-16,1.,0.));
#43669=DIRECTION('',(-1.46081976924362E-16,1.,0.));
#43670=DIRECTION('center_axis',(1.,1.46081976924362E-16,0.));
#43671=DIRECTION('ref_axis',(-1.46081976924362E-16,1.,0.));
#43672=DIRECTION('',(-1.46081976924362E-16,1.,0.));
#43673=DIRECTION('',(-1.46081976924362E-16,1.,0.));
#43674=DIRECTION('center_axis',(1.,1.46081976924362E-16,0.));
#43675=DIRECTION('ref_axis',(-1.46081976924362E-16,1.,0.));
#43676=DIRECTION('',(-1.46081976924362E-16,1.,0.));
#43677=DIRECTION('',(-1.46081976924362E-16,1.,0.));
#43678=DIRECTION('center_axis',(1.,1.46081976924362E-16,0.));
#43679=DIRECTION('ref_axis',(-1.46081976924362E-16,1.,0.));
#43680=DIRECTION('',(1.46081976924362E-16,-1.,0.));
#43681=DIRECTION('',(1.46081976924362E-16,-1.,0.));
#43682=DIRECTION('center_axis',(-1.,-1.46081976924362E-16,0.));
#43683=DIRECTION('ref_axis',(-1.46081976924362E-16,1.,0.));
#43684=DIRECTION('',(1.46081976924362E-16,-1.,0.));
#43685=DIRECTION('',(1.46081976924362E-16,-1.,0.));
#43686=DIRECTION('center_axis',(-1.,-1.46081976924362E-16,0.));
#43687=DIRECTION('ref_axis',(-1.46081976924362E-16,1.,0.));
#43688=DIRECTION('',(1.46081976924362E-16,-1.,0.));
#43689=DIRECTION('',(1.46081976924362E-16,-1.,0.));
#43690=DIRECTION('center_axis',(-1.,-1.46081976924362E-16,0.));
#43691=DIRECTION('ref_axis',(-1.46081976924362E-16,1.,0.));
#43692=DIRECTION('',(-1.46081976924362E-16,1.,0.));
#43693=DIRECTION('',(-1.46081976924362E-16,1.,0.));
#43694=DIRECTION('center_axis',(1.,1.46081976924362E-16,0.));
#43695=DIRECTION('ref_axis',(-1.46081976924362E-16,1.,0.));
#43696=DIRECTION('',(1.46081976924362E-16,-1.,0.));
#43697=DIRECTION('',(1.46081976924362E-16,-1.,0.));
#43698=DIRECTION('center_axis',(-1.,-1.46081976924362E-16,0.));
#43699=DIRECTION('ref_axis',(-1.46081976924362E-16,1.,0.));
#43700=DIRECTION('',(1.46081976924362E-16,-1.,0.));
#43701=DIRECTION('',(1.46081976924362E-16,-1.,0.));
#43702=DIRECTION('center_axis',(-1.,-1.46081976924362E-16,0.));
#43703=DIRECTION('ref_axis',(-1.46081976924362E-16,1.,0.));
#43704=DIRECTION('',(1.46081976924362E-16,-1.,0.));
#43705=DIRECTION('',(1.46081976924362E-16,-1.,0.));
#43706=DIRECTION('center_axis',(-1.,-1.46081976924362E-16,0.));
#43707=DIRECTION('ref_axis',(-1.46081976924362E-16,1.,0.));
#43708=DIRECTION('',(1.46081976924362E-16,-1.,0.));
#43709=DIRECTION('',(1.46081976924362E-16,-1.,0.));
#43710=DIRECTION('center_axis',(-1.,-1.46081976924362E-16,0.));
#43711=DIRECTION('ref_axis',(-1.46081976924362E-16,1.,0.));
#43712=DIRECTION('',(1.46081976924362E-16,-1.,0.));
#43713=DIRECTION('',(1.46081976924362E-16,-1.,0.));
#43714=DIRECTION('center_axis',(-1.,-1.46081976924362E-16,0.));
#43715=DIRECTION('ref_axis',(-1.46081976924362E-16,1.,0.));
#43716=DIRECTION('',(-1.46081976924362E-16,1.,0.));
#43717=DIRECTION('',(-1.46081976924362E-16,1.,0.));
#43718=DIRECTION('center_axis',(1.,1.46081976924362E-16,0.));
#43719=DIRECTION('ref_axis',(-1.46081976924362E-16,1.,0.));
#43720=DIRECTION('',(1.46081976924362E-16,-1.,0.));
#43721=DIRECTION('',(1.46081976924362E-16,-1.,0.));
#43722=DIRECTION('center_axis',(-1.,-1.46081976924362E-16,0.));
#43723=DIRECTION('ref_axis',(-1.46081976924362E-16,1.,0.));
#43724=DIRECTION('',(-1.46081976924362E-16,1.,0.));
#43725=DIRECTION('',(-1.46081976924362E-16,1.,0.));
#43726=DIRECTION('center_axis',(1.,1.46081976924362E-16,0.));
#43727=DIRECTION('ref_axis',(-1.46081976924362E-16,1.,0.));
#43728=DIRECTION('',(-1.46081976924362E-16,1.,0.));
#43729=DIRECTION('center_axis',(-1.,-1.46081976924362E-16,0.));
#43730=DIRECTION('ref_axis',(-1.46081976924362E-16,1.,0.));
#43731=DIRECTION('',(-1.46081976924362E-16,1.,0.));
#43732=DIRECTION('',(-1.46081976924362E-16,1.,0.));
#43733=DIRECTION('center_axis',(-1.,-1.46081976924362E-16,0.));
#43734=DIRECTION('ref_axis',(-1.46081976924362E-16,1.,0.));
#43735=DIRECTION('',(-1.46081976924362E-16,1.,0.));
#43736=DIRECTION('',(-1.46081976924362E-16,1.,0.));
#43737=DIRECTION('center_axis',(-1.,-1.46081976924362E-16,0.));
#43738=DIRECTION('ref_axis',(-1.46081976924362E-16,1.,0.));
#43739=DIRECTION('',(-1.46081976924362E-16,1.,0.));
#43740=DIRECTION('',(-1.46081976924362E-16,1.,0.));
#43741=DIRECTION('center_axis',(-1.,-1.46081976924362E-16,0.));
#43742=DIRECTION('ref_axis',(-1.46081976924362E-16,1.,0.));
#43743=DIRECTION('',(-1.46081976924362E-16,1.,0.));
#43744=DIRECTION('',(1.46081976924362E-16,-1.,0.));
#43745=DIRECTION('center_axis',(1.,1.46081976924362E-16,0.));
#43746=DIRECTION('ref_axis',(-1.46081976924362E-16,1.,0.));
#43747=DIRECTION('',(1.46081976924362E-16,-1.,0.));
#43748=DIRECTION('',(1.46081976924362E-16,-1.,0.));
#43749=DIRECTION('center_axis',(1.,1.46081976924362E-16,0.));
#43750=DIRECTION('ref_axis',(-1.46081976924362E-16,1.,0.));
#43751=DIRECTION('',(1.46081976924362E-16,-1.,0.));
#43752=DIRECTION('',(1.46081976924362E-16,-1.,0.));
#43753=DIRECTION('center_axis',(1.,1.46081976924362E-16,0.));
#43754=DIRECTION('ref_axis',(-1.46081976924362E-16,1.,0.));
#43755=DIRECTION('',(1.46081976924362E-16,-1.,0.));
#43756=DIRECTION('',(1.46081976924362E-16,-1.,0.));
#43757=DIRECTION('center_axis',(1.,1.46081976924362E-16,0.));
#43758=DIRECTION('ref_axis',(-1.46081976924362E-16,1.,0.));
#43759=DIRECTION('',(1.46081976924362E-16,-1.,0.));
#43760=DIRECTION('',(-1.46081976924362E-16,1.,0.));
#43761=DIRECTION('center_axis',(-1.,-1.46081976924362E-16,0.));
#43762=DIRECTION('ref_axis',(-1.46081976924362E-16,1.,0.));
#43763=DIRECTION('',(-1.46081976924362E-16,1.,0.));
#43764=DIRECTION('',(1.46081976924362E-16,-1.,0.));
#43765=DIRECTION('center_axis',(1.,1.46081976924362E-16,0.));
#43766=DIRECTION('ref_axis',(-1.46081976924362E-16,1.,0.));
#43767=DIRECTION('',(1.46081976924362E-16,-1.,0.));
#43768=DIRECTION('',(-1.46081976924362E-16,1.,0.));
#43769=DIRECTION('center_axis',(-1.,-1.46081976924362E-16,0.));
#43770=DIRECTION('ref_axis',(-1.46081976924362E-16,1.,0.));
#43771=DIRECTION('',(-1.46081976924362E-16,1.,0.));
#43772=DIRECTION('center_axis',(-3.79532109154651E-16,0.866025403784439,
0.499999999999999));
#43773=DIRECTION('ref_axis',(-7.94699513894569E-33,-0.499999999999999,0.866025403784439));
#43774=DIRECTION('',(-3.46944695195361E-16,0.499999999999999,-0.866025403784439));
#43775=DIRECTION('',(2.19122965386544E-16,-0.499999999999999,0.866025403784439));
#43776=DIRECTION('',(-1.,-4.38245930773088E-16,0.));
#43777=DIRECTION('center_axis',(-3.79532109154651E-16,0.866025403784439,
0.499999999999999));
#43778=DIRECTION('ref_axis',(-7.94699513894569E-33,-0.499999999999999,0.866025403784439));
#43779=DIRECTION('',(2.19122965386544E-16,-0.499999999999999,0.866025403784439));
#43780=DIRECTION('',(-1.,-4.38245930773088E-16,0.));
#43781=DIRECTION('',(-3.46944695195361E-16,0.499999999999999,-0.866025403784439));
#43782=DIRECTION('center_axis',(3.79532109154651E-16,-0.866025403784439,
-0.499999999999999));
#43783=DIRECTION('ref_axis',(1.5326347767966E-32,0.499999999999999,-0.866025403784439));
#43784=DIRECTION('',(3.46944695195362E-16,-0.499999999999999,0.866025403784439));
#43785=DIRECTION('',(1.,4.38245930773088E-16,0.));
#43786=DIRECTION('',(-2.19122965386544E-16,0.499999999999999,-0.866025403784439));
#43787=DIRECTION('',(-1.,-4.38245930773088E-16,0.));
#43788=DIRECTION('center_axis',(-3.79532109154651E-16,0.866025403784438,
-0.5));
#43789=DIRECTION('ref_axis',(1.94620289117031E-33,0.5,0.866025403784438));
#43790=DIRECTION('',(-2.19122965386544E-16,0.5,0.866025403784438));
#43791=DIRECTION('',(0.,-0.5,-0.866025403784438));
#43792=DIRECTION('',(1.,4.38245930773088E-16,8.64002241377108E-33));
#43793=DIRECTION('center_axis',(3.79532109154651E-16,-0.866025403784438,
0.5));
#43794=DIRECTION('ref_axis',(-1.94620289117031E-33,-0.5,-0.866025403784438));
#43795=DIRECTION('',(0.,0.5,0.866025403784438));
#43796=DIRECTION('',(1.,4.38245930773088E-16,8.64002241377108E-33));
#43797=DIRECTION('',(2.19122965386544E-16,-0.5,-0.866025403784438));
#43798=DIRECTION('',(-1.,-4.38245930773088E-16,-8.64002241377108E-33));
#43799=DIRECTION('center_axis',(0.,0.,-1.));
#43800=DIRECTION('ref_axis',(-1.,0.,0.));
#43801=DIRECTION('',(-4.38245930773088E-16,1.,0.));
#43802=DIRECTION('',(4.38245930773088E-16,-1.,0.));
#43803=DIRECTION('',(1.,4.38245930773088E-16,0.));
#43804=DIRECTION('center_axis',(0.,0.,1.));
#43805=DIRECTION('ref_axis',(1.,0.,0.));
#43806=DIRECTION('',(-4.38245930773088E-16,1.,0.));
#43807=DIRECTION('',(4.38245930773088E-16,-1.,0.));
#43808=DIRECTION('',(-1.,-4.38245930773088E-16,0.));
#43809=DIRECTION('center_axis',(3.79532109154651E-16,-0.866025403784439,
-0.5));
#43810=DIRECTION('ref_axis',(-8.35245407460559E-33,0.5,-0.866025403784439));
#43811=DIRECTION('',(-2.19122965386544E-16,0.5,-0.866025403784439));
#43812=DIRECTION('',(-1.,-4.38245930773088E-16,0.));
#43813=DIRECTION('',(0.,-0.5,0.866025403784439));
#43814=DIRECTION('',(1.,4.38245930773088E-16,0.));
#43815=DIRECTION('center_axis',(3.79532109154651E-16,-0.866025403784438,
0.5));
#43816=DIRECTION('ref_axis',(2.27057003969863E-32,-0.5,-0.866025403784438));
#43817=DIRECTION('',(2.19122965386544E-16,-0.5,-0.866025403784438));
#43818=DIRECTION('',(-1.,-4.38245930773088E-16,0.));
#43819=DIRECTION('',(-3.46944695195361E-16,0.5,0.866025403784438));
#43820=DIRECTION('',(1.,4.38245930773088E-16,0.));
#43821=DIRECTION('center_axis',(-3.79532109154651E-16,0.866025403784439,
-0.5));
#43822=DIRECTION('ref_axis',(-1.08662994757006E-32,0.5,0.866025403784439));
#43823=DIRECTION('',(3.46944695195361E-16,-0.5,-0.866025403784438));
#43824=DIRECTION('',(1.,4.38245930773088E-16,0.));
#43825=DIRECTION('',(-2.19122965386544E-16,0.5,0.866025403784438));
#43826=DIRECTION('center_axis',(0.,0.,1.));
#43827=DIRECTION('ref_axis',(1.,0.,0.));
#43828=DIRECTION('',(4.38245930773088E-16,-1.,0.));
#43829=DIRECTION('',(-1.,-4.38245930773088E-16,0.));
#43830=DIRECTION('',(-4.38245930773088E-16,1.,0.));
#43831=DIRECTION('',(1.,4.38245930773088E-16,0.));
#43832=DIRECTION('center_axis',(0.,0.,-1.));
#43833=DIRECTION('ref_axis',(-1.,0.,0.));
#43834=DIRECTION('',(-4.38245930773088E-16,1.,0.));
#43835=DIRECTION('',(-1.,-4.38245930773088E-16,0.));
#43836=DIRECTION('',(4.38245930773088E-16,-1.,0.));
#43837=DIRECTION('',(1.,4.38245930773088E-16,0.));
#43838=DIRECTION('center_axis',(-3.79532109154651E-16,0.866025403784439,
0.499999999999999));
#43839=DIRECTION('ref_axis',(-7.94699513894569E-33,-0.499999999999999,0.866025403784439));
#43840=DIRECTION('',(-3.46944695195361E-16,0.499999999999999,-0.866025403784439));
#43841=DIRECTION('',(2.19122965386544E-16,-0.499999999999999,0.866025403784439));
#43842=DIRECTION('',(-1.,-4.38245930773088E-16,0.));
#43843=DIRECTION('center_axis',(-3.79532109154651E-16,0.866025403784439,
0.499999999999999));
#43844=DIRECTION('ref_axis',(-7.94699513894569E-33,-0.499999999999999,0.866025403784439));
#43845=DIRECTION('',(2.19122965386544E-16,-0.499999999999999,0.866025403784439));
#43846=DIRECTION('',(-1.,-4.38245930773088E-16,0.));
#43847=DIRECTION('',(-3.46944695195361E-16,0.499999999999999,-0.866025403784439));
#43848=DIRECTION('center_axis',(3.79532109154651E-16,-0.866025403784439,
-0.499999999999999));
#43849=DIRECTION('ref_axis',(1.5326347767966E-32,0.499999999999999,-0.866025403784439));
#43850=DIRECTION('',(3.46944695195362E-16,-0.499999999999999,0.866025403784439));
#43851=DIRECTION('',(1.,4.38245930773088E-16,0.));
#43852=DIRECTION('',(-2.19122965386544E-16,0.499999999999999,-0.866025403784439));
#43853=DIRECTION('',(-1.,-4.38245930773088E-16,0.));
#43854=DIRECTION('center_axis',(-3.79532109154651E-16,0.866025403784438,
-0.5));
#43855=DIRECTION('ref_axis',(1.94620289117031E-33,0.5,0.866025403784438));
#43856=DIRECTION('',(-2.19122965386544E-16,0.5,0.866025403784438));
#43857=DIRECTION('',(0.,-0.5,-0.866025403784438));
#43858=DIRECTION('',(1.,4.38245930773088E-16,8.64002241377108E-33));
#43859=DIRECTION('center_axis',(3.79532109154651E-16,-0.866025403784438,
0.5));
#43860=DIRECTION('ref_axis',(-1.94620289117031E-33,-0.5,-0.866025403784438));
#43861=DIRECTION('',(0.,0.5,0.866025403784438));
#43862=DIRECTION('',(1.,4.38245930773088E-16,6.16297582203917E-33));
#43863=DIRECTION('',(2.19122965386544E-16,-0.5,-0.866025403784438));
#43864=DIRECTION('',(-1.,-4.38245930773088E-16,-8.64002241377108E-33));
#43865=DIRECTION('center_axis',(0.,0.,-1.));
#43866=DIRECTION('ref_axis',(-1.,0.,0.));
#43867=DIRECTION('',(-4.38245930773088E-16,1.,0.));
#43868=DIRECTION('',(4.38245930773088E-16,-1.,0.));
#43869=DIRECTION('',(1.,4.38245930773088E-16,0.));
#43870=DIRECTION('center_axis',(0.,0.,1.));
#43871=DIRECTION('ref_axis',(1.,0.,0.));
#43872=DIRECTION('',(-4.38245930773088E-16,1.,0.));
#43873=DIRECTION('',(4.38245930773088E-16,-1.,0.));
#43874=DIRECTION('',(-1.,-4.38245930773088E-16,0.));
#43875=DIRECTION('center_axis',(3.79532109154651E-16,-0.866025403784439,
-0.5));
#43876=DIRECTION('ref_axis',(-8.35245407460559E-33,0.5,-0.866025403784439));
#43877=DIRECTION('',(-2.19122965386544E-16,0.5,-0.866025403784439));
#43878=DIRECTION('',(-1.,-4.38245930773088E-16,0.));
#43879=DIRECTION('',(0.,-0.5,0.866025403784439));
#43880=DIRECTION('',(1.,4.38245930773088E-16,0.));
#43881=DIRECTION('center_axis',(3.79532109154651E-16,-0.866025403784438,
0.5));
#43882=DIRECTION('ref_axis',(2.27057003969863E-32,-0.5,-0.866025403784438));
#43883=DIRECTION('',(2.19122965386544E-16,-0.5,-0.866025403784438));
#43884=DIRECTION('',(-1.,-4.38245930773088E-16,0.));
#43885=DIRECTION('',(-3.46944695195361E-16,0.5,0.866025403784438));
#43886=DIRECTION('',(1.,4.38245930773088E-16,0.));
#43887=DIRECTION('center_axis',(-3.79532109154651E-16,0.866025403784439,
-0.5));
#43888=DIRECTION('ref_axis',(-1.08662994757006E-32,0.5,0.866025403784439));
#43889=DIRECTION('',(3.46944695195361E-16,-0.5,-0.866025403784438));
#43890=DIRECTION('',(1.,4.38245930773088E-16,0.));
#43891=DIRECTION('',(-2.19122965386544E-16,0.5,0.866025403784438));
#43892=DIRECTION('center_axis',(0.,0.,1.));
#43893=DIRECTION('ref_axis',(1.,0.,0.));
#43894=DIRECTION('',(4.38245930773088E-16,-1.,0.));
#43895=DIRECTION('',(-1.,-4.38245930773088E-16,0.));
#43896=DIRECTION('',(-4.38245930773088E-16,1.,0.));
#43897=DIRECTION('',(1.,4.38245930773088E-16,0.));
#43898=DIRECTION('center_axis',(0.,0.,-1.));
#43899=DIRECTION('ref_axis',(-1.,0.,0.));
#43900=DIRECTION('',(-4.38245930773088E-16,1.,0.));
#43901=DIRECTION('',(-1.,-4.38245930773088E-16,0.));
#43902=DIRECTION('',(4.38245930773088E-16,-1.,0.));
#43903=DIRECTION('',(1.,4.38245930773088E-16,0.));
#43904=DIRECTION('',(-1.,-4.38245930773088E-16,0.));
#43905=DIRECTION('',(1.,4.38245930773088E-16,0.));
#43906=DIRECTION('center_axis',(-1.,-4.38245930773088E-16,0.));
#43907=DIRECTION('ref_axis',(0.,0.,1.));
#43908=DIRECTION('center_axis',(-1.,-4.38245930773088E-16,0.));
#43909=DIRECTION('ref_axis',(4.38245930773088E-16,-1.,0.));
#43910=DIRECTION('center_axis',(-1.,-4.38245930773088E-16,0.));
#43911=DIRECTION('ref_axis',(4.38245930773088E-16,-1.,0.));
#43912=DIRECTION('center_axis',(-1.,-4.38245930773088E-16,0.));
#43913=DIRECTION('ref_axis',(4.38245930773088E-16,-1.,0.));
#43914=DIRECTION('center_axis',(-1.,-4.38245930773088E-16,0.));
#43915=DIRECTION('ref_axis',(4.38245930773088E-16,-1.,0.));
#43916=DIRECTION('',(2.19122965386544E-16,-0.5,-0.866025403784438));
#43917=DIRECTION('center_axis',(-1.,-4.38245930773088E-16,0.));
#43918=DIRECTION('ref_axis',(4.38245930773088E-16,-1.,0.));
#43919=DIRECTION('center_axis',(-1.,-4.38245930773088E-16,0.));
#43920=DIRECTION('ref_axis',(4.38245930773088E-16,-1.,0.));
#43921=DIRECTION('',(2.19122965386544E-16,-0.499999999999999,0.866025403784439));
#43922=DIRECTION('',(4.38245930773088E-16,-1.,0.));
#43923=DIRECTION('center_axis',(-1.,-4.38245930773088E-16,0.));
#43924=DIRECTION('ref_axis',(4.38245930773088E-16,-1.,0.));
#43925=DIRECTION('',(-2.19122965386544E-16,0.5,0.866025403784438));
#43926=DIRECTION('center_axis',(-1.,-4.38245930773088E-16,0.));
#43927=DIRECTION('ref_axis',(4.38245930773088E-16,-1.,0.));
#43928=DIRECTION('center_axis',(-1.,-4.38245930773088E-16,0.));
#43929=DIRECTION('ref_axis',(4.38245930773088E-16,-1.,0.));
#43930=DIRECTION('',(2.19122965386544E-16,-0.499999999999999,0.866025403784439));
#43931=DIRECTION('center_axis',(-1.,-4.38245930773088E-16,0.));
#43932=DIRECTION('ref_axis',(4.38245930773088E-16,-1.,0.));
#43933=DIRECTION('',(-4.38245930773088E-16,1.,0.));
#43934=DIRECTION('center_axis',(-1.,-4.38245930773088E-16,0.));
#43935=DIRECTION('ref_axis',(4.38245930773088E-16,-1.,0.));
#43936=DIRECTION('center_axis',(-1.,-4.38245930773088E-16,0.));
#43937=DIRECTION('ref_axis',(4.38245930773088E-16,-1.,0.));
#43938=DIRECTION('',(-2.19122965386544E-16,0.5,0.866025403784438));
#43939=DIRECTION('center_axis',(-1.,-4.38245930773088E-16,0.));
#43940=DIRECTION('ref_axis',(4.38245930773088E-16,-1.,0.));
#43941=DIRECTION('center_axis',(-1.,-4.38245930773088E-16,0.));
#43942=DIRECTION('ref_axis',(4.38245930773088E-16,-1.,0.));
#43943=DIRECTION('',(-2.19122965386544E-16,0.499999999999999,-0.866025403784439));
#43944=DIRECTION('center_axis',(-1.,-4.38245930773088E-16,0.));
#43945=DIRECTION('ref_axis',(4.38245930773088E-16,-1.,0.));
#43946=DIRECTION('',(-4.38245930773088E-16,1.,0.));
#43947=DIRECTION('center_axis',(-1.,-4.38245930773088E-16,0.));
#43948=DIRECTION('ref_axis',(4.38245930773088E-16,-1.,0.));
#43949=DIRECTION('center_axis',(-1.,-4.38245930773088E-16,0.));
#43950=DIRECTION('ref_axis',(4.38245930773088E-16,-1.,0.));
#43951=DIRECTION('',(2.19122965386544E-16,-0.5,-0.866025403784438));
#43952=DIRECTION('center_axis',(-1.,-4.38245930773088E-16,0.));
#43953=DIRECTION('ref_axis',(4.38245930773088E-16,-1.,0.));
#43954=DIRECTION('',(-2.19122965386544E-16,0.5,-0.866025403784439));
#43955=DIRECTION('center_axis',(-1.,-4.38245930773088E-16,0.));
#43956=DIRECTION('ref_axis',(4.38245930773088E-16,-1.,0.));
#43957=DIRECTION('center_axis',(-1.,-4.38245930773088E-16,0.));
#43958=DIRECTION('ref_axis',(4.38245930773088E-16,-1.,0.));
#43959=DIRECTION('',(4.38245930773088E-16,-1.,0.));
#43960=DIRECTION('center_axis',(-1.,-4.38245930773088E-16,0.));
#43961=DIRECTION('ref_axis',(4.38245930773088E-16,-1.,0.));
#43962=DIRECTION('center_axis',(-1.,-4.38245930773088E-16,0.));
#43963=DIRECTION('ref_axis',(4.38245930773088E-16,-1.,0.));
#43964=DIRECTION('center_axis',(-1.,-4.38245930773088E-16,0.));
#43965=DIRECTION('ref_axis',(4.38245930773088E-16,-1.,0.));
#43966=DIRECTION('center_axis',(-1.,-4.38245930773088E-16,0.));
#43967=DIRECTION('ref_axis',(4.38245930773088E-16,-1.,0.));
#43968=DIRECTION('center_axis',(-1.,-4.38245930773088E-16,0.));
#43969=DIRECTION('ref_axis',(4.38245930773088E-16,-1.,0.));
#43970=DIRECTION('center_axis',(-1.,-4.38245930773088E-16,0.));
#43971=DIRECTION('ref_axis',(4.38245930773088E-16,-1.,0.));
#43972=DIRECTION('center_axis',(-1.,-4.38245930773088E-16,0.));
#43973=DIRECTION('ref_axis',(4.38245930773088E-16,-1.,0.));
#43974=DIRECTION('center_axis',(-1.,-4.38245930773088E-16,0.));
#43975=DIRECTION('ref_axis',(4.38245930773088E-16,-1.,0.));
#43976=DIRECTION('center_axis',(-1.,-4.38245930773088E-16,0.));
#43977=DIRECTION('ref_axis',(4.38245930773088E-16,-1.,0.));
#43978=DIRECTION('center_axis',(-1.,-4.38245930773088E-16,0.));
#43979=DIRECTION('ref_axis',(4.38245930773088E-16,-1.,0.));
#43980=DIRECTION('center_axis',(-1.,-4.38245930773088E-16,0.));
#43981=DIRECTION('ref_axis',(4.38245930773088E-16,-1.,0.));
#43982=DIRECTION('center_axis',(-1.,-4.38245930773088E-16,0.));
#43983=DIRECTION('ref_axis',(4.38245930773088E-16,-1.,0.));
#43984=DIRECTION('center_axis',(-1.,-4.38245930773088E-16,0.));
#43985=DIRECTION('ref_axis',(4.38245930773088E-16,-1.,0.));
#43986=DIRECTION('center_axis',(-1.,-4.38245930773088E-16,0.));
#43987=DIRECTION('ref_axis',(4.38245930773088E-16,-1.,0.));
#43988=DIRECTION('center_axis',(-1.,-4.38245930773088E-16,0.));
#43989=DIRECTION('ref_axis',(4.38245930773088E-16,-1.,0.));
#43990=DIRECTION('center_axis',(-1.,-4.38245930773088E-16,0.));
#43991=DIRECTION('ref_axis',(4.38245930773088E-16,-1.,0.));
#43992=DIRECTION('center_axis',(-1.,-4.38245930773088E-16,0.));
#43993=DIRECTION('ref_axis',(4.38245930773088E-16,-1.,0.));
#43994=DIRECTION('center_axis',(-1.,-4.38245930773088E-16,0.));
#43995=DIRECTION('ref_axis',(4.38245930773088E-16,-1.,0.));
#43996=DIRECTION('center_axis',(-1.,-4.38245930773088E-16,0.));
#43997=DIRECTION('ref_axis',(4.38245930773088E-16,-1.,0.));
#43998=DIRECTION('center_axis',(-1.,-4.38245930773088E-16,0.));
#43999=DIRECTION('ref_axis',(4.38245930773088E-16,-1.,0.));
#44000=DIRECTION('center_axis',(-1.,-4.38245930773088E-16,0.));
#44001=DIRECTION('ref_axis',(4.38245930773088E-16,-1.,0.));
#44002=DIRECTION('center_axis',(-1.,-4.38245930773088E-16,0.));
#44003=DIRECTION('ref_axis',(4.38245930773088E-16,-1.,0.));
#44004=DIRECTION('center_axis',(-1.,-4.38245930773088E-16,0.));
#44005=DIRECTION('ref_axis',(4.38245930773088E-16,-1.,0.));
#44006=DIRECTION('center_axis',(-1.,-4.38245930773088E-16,0.));
#44007=DIRECTION('ref_axis',(4.38245930773088E-16,-1.,0.));
#44008=DIRECTION('center_axis',(-1.,-4.38245930773088E-16,0.));
#44009=DIRECTION('ref_axis',(4.38245930773088E-16,-1.,0.));
#44010=DIRECTION('center_axis',(-1.,-4.38245930773088E-16,0.));
#44011=DIRECTION('ref_axis',(4.38245930773088E-16,-1.,0.));
#44012=DIRECTION('center_axis',(-1.,-4.38245930773088E-16,0.));
#44013=DIRECTION('ref_axis',(4.38245930773088E-16,-1.,0.));
#44014=DIRECTION('center_axis',(-1.,-4.38245930773088E-16,0.));
#44015=DIRECTION('ref_axis',(4.38245930773088E-16,-1.,0.));
#44016=DIRECTION('center_axis',(-1.,-4.38245930773088E-16,0.));
#44017=DIRECTION('ref_axis',(4.38245930773088E-16,-1.,0.));
#44018=DIRECTION('center_axis',(-1.,-4.38245930773088E-16,0.));
#44019=DIRECTION('ref_axis',(4.38245930773088E-16,-1.,0.));
#44020=DIRECTION('center_axis',(-1.,-4.38245930773088E-16,0.));
#44021=DIRECTION('ref_axis',(4.38245930773088E-16,-1.,0.));
#44022=DIRECTION('center_axis',(-1.,-4.38245930773088E-16,0.));
#44023=DIRECTION('ref_axis',(4.38245930773088E-16,-1.,0.));
#44024=DIRECTION('center_axis',(-1.,-4.38245930773088E-16,0.));
#44025=DIRECTION('ref_axis',(4.38245930773088E-16,-1.,0.));
#44026=DIRECTION('center_axis',(-1.,-4.38245930773088E-16,0.));
#44027=DIRECTION('ref_axis',(4.38245930773088E-16,-1.,0.));
#44028=DIRECTION('center_axis',(-3.79532109154651E-16,0.866025403784439,
0.499999999999999));
#44029=DIRECTION('ref_axis',(-7.94699513894569E-33,-0.499999999999999,0.866025403784439));
#44030=DIRECTION('',(-3.46944695195361E-16,0.499999999999999,-0.866025403784439));
#44031=DIRECTION('',(-1.,-4.38245930773088E-16,0.));
#44032=DIRECTION('',(1.,4.38245930773088E-16,0.));
#44033=DIRECTION('',(-1.,-4.38245930773088E-16,0.));
#44034=DIRECTION('',(-1.,-4.38245930773088E-16,0.));
#44035=DIRECTION('center_axis',(-1.,-4.38245930773088E-16,0.));
#44036=DIRECTION('ref_axis',(4.38245930773088E-16,-1.,0.));
#44037=DIRECTION('',(0.,0.,-1.));
#44038=DIRECTION('',(3.09886669477061E-16,-0.707106781186547,-0.707106781186547));
#44039=DIRECTION('',(-4.38245930773088E-16,1.,0.));
#44040=DIRECTION('',(0.,0.,-1.));
#44041=DIRECTION('center_axis',(-1.,-4.38245930773088E-16,0.));
#44042=DIRECTION('ref_axis',(4.38245930773088E-16,-1.,0.));
#44043=DIRECTION('',(0.,0.,-1.));
#44044=DIRECTION('center_axis',(-1.,-4.38245930773088E-16,0.));
#44045=DIRECTION('ref_axis',(4.38245930773088E-16,-1.,0.));
#44046=DIRECTION('',(0.,0.,-1.));
#44047=DIRECTION('',(-4.38245930773088E-16,1.,0.));
#44048=DIRECTION('',(-3.09886669477061E-16,0.707106781186547,-0.707106781186547));
#44049=DIRECTION('',(0.,2.77555756156289E-15,1.));
#44050=DIRECTION('',(0.,-1.,0.));
#44051=DIRECTION('',(0.,-4.16333634234433E-15,-1.));
#44052=DIRECTION('',(0.,1.,0.));
#44053=DIRECTION('center_axis',(-1.,-4.38245930773088E-16,0.));
#44054=DIRECTION('ref_axis',(4.38245930773088E-16,-1.,0.));
#44055=DIRECTION('',(0.,1.,0.));
#44056=DIRECTION('center_axis',(-1.,-4.38245930773088E-16,0.));
#44057=DIRECTION('ref_axis',(4.38245930773088E-16,-1.,0.));
#44058=DIRECTION('',(0.,0.707106781186552,0.707106781186543));
#44059=DIRECTION('center_axis',(-1.,-4.38245930773088E-16,0.));
#44060=DIRECTION('ref_axis',(4.38245930773088E-16,-1.,0.));
#44061=DIRECTION('',(0.,1.8333618114597E-15,1.));
#44062=DIRECTION('center_axis',(-1.,-4.38245930773088E-16,0.));
#44063=DIRECTION('ref_axis',(4.38245930773088E-16,-1.,0.));
#44064=DIRECTION('',(0.,-0.707106781186551,0.707106781186544));
#44065=DIRECTION('center_axis',(-1.,-4.38245930773088E-16,0.));
#44066=DIRECTION('ref_axis',(4.38245930773088E-16,-1.,0.));
#44067=DIRECTION('',(0.,-1.,-1.3325595315168E-15));
#44068=DIRECTION('center_axis',(-1.,-4.38245930773088E-16,0.));
#44069=DIRECTION('ref_axis',(4.38245930773088E-16,-1.,0.));
#44070=DIRECTION('',(0.,0.,-1.));
#44071=DIRECTION('center_axis',(-1.,-4.38245930773088E-16,0.));
#44072=DIRECTION('ref_axis',(4.38245930773088E-16,-1.,0.));
#44073=DIRECTION('',(-4.38245930773088E-16,1.,0.));
#44074=DIRECTION('',(-3.09886669477061E-16,0.707106781186547,0.707106781186547));
#44075=DIRECTION('',(0.,0.,-1.));
#44076=DIRECTION('',(3.09886669477061E-16,-0.707106781186547,0.707106781186547));
#44077=DIRECTION('',(-4.38245930773088E-16,1.,0.));
#44078=DIRECTION('',(0.,0.,1.));
#44079=DIRECTION('center_axis',(-1.,-4.38245930773088E-16,0.));
#44080=DIRECTION('ref_axis',(4.38245930773088E-16,-1.,0.));
#44081=DIRECTION('',(0.,0.,-1.));
#44082=DIRECTION('center_axis',(1.,6.12323399573677E-17,0.));
#44083=DIRECTION('ref_axis',(0.,0.,1.));
#44084=DIRECTION('',(0.,0.,1.));
#44085=DIRECTION('',(4.38245930773088E-16,-1.,0.));
#44086=DIRECTION('',(-1.21637680698141E-30,2.77555756156289E-15,1.));
#44087=DIRECTION('',(-4.38245930773088E-16,1.,0.));
#44088=DIRECTION('',(1.82456521047212E-30,-4.16333634234433E-15,-1.));
#44089=DIRECTION('',(-4.38245930773088E-16,1.,0.));
#44090=DIRECTION('center_axis',(-1.,-4.38245930773088E-16,0.));
#44091=DIRECTION('ref_axis',(4.38245930773088E-16,-1.,0.));
#44092=DIRECTION('',(0.,0.,-1.));
#44093=DIRECTION('center_axis',(-1.,-4.38245930773088E-16,0.));
#44094=DIRECTION('ref_axis',(4.38245930773088E-16,-1.,0.));
#44095=DIRECTION('',(4.38245930773088E-16,-1.,-1.3325595315168E-15));
#44096=DIRECTION('center_axis',(-1.,-4.38245930773088E-16,0.));
#44097=DIRECTION('ref_axis',(4.38245930773088E-16,-1.,0.));
#44098=DIRECTION('',(3.09886669477062E-16,-0.707106781186551,0.707106781186544));
#44099=DIRECTION('center_axis',(-1.,-4.38245930773088E-16,0.));
#44100=DIRECTION('ref_axis',(4.38245930773088E-16,-1.,0.));
#44101=DIRECTION('',(-8.03463353506993E-31,1.8333618114597E-15,1.));
#44102=DIRECTION('center_axis',(-1.,-4.38245930773088E-16,0.));
#44103=DIRECTION('ref_axis',(4.38245930773088E-16,-1.,0.));
#44104=DIRECTION('',(-3.09886669477063E-16,0.707106781186552,0.707106781186543));
#44105=DIRECTION('center_axis',(-1.,-4.38245930773088E-16,0.));
#44106=DIRECTION('ref_axis',(4.38245930773088E-16,-1.,0.));
#44107=DIRECTION('center_axis',(0.,1.,0.));
#44108=DIRECTION('ref_axis',(0.,0.,1.));
#44109=DIRECTION('',(0.,-1.,-1.11022302462516E-14));
#44110=DIRECTION('',(0.,1.,0.));
#44111=DIRECTION('',(0.,-1.,-1.11022302462516E-14));
#44112=DIRECTION('center_axis',(-1.,0.,0.));
#44113=DIRECTION('ref_axis',(0.,0.,1.));
#44114=DIRECTION('center_axis',(0.,1.,0.));
#44115=DIRECTION('ref_axis',(0.,0.,1.));
#44116=DIRECTION('',(0.,1.,0.));
#44117=DIRECTION('',(0.,1.,0.));
#44118=DIRECTION('',(0.,1.,0.));
#44119=DIRECTION('center_axis',(-1.,0.,0.));
#44120=DIRECTION('ref_axis',(0.,0.,1.));
#44121=DIRECTION('center_axis',(0.,1.,0.));
#44122=DIRECTION('ref_axis',(0.,0.,1.));
#44123=DIRECTION('',(-2.22044604925031E-14,-1.,-2.22044604925031E-14));
#44124=DIRECTION('',(0.,1.,0.));
#44125=DIRECTION('',(-2.22044604925031E-14,-1.,-2.22044604925031E-14));
#44126=DIRECTION('center_axis',(1.,0.,0.));
#44127=DIRECTION('ref_axis',(0.,0.,-1.));
#44128=DIRECTION('center_axis',(0.,1.,0.));
#44129=DIRECTION('ref_axis',(0.,0.,1.));
#44130=DIRECTION('',(0.,1.,0.));
#44131=DIRECTION('',(0.,1.,0.));
#44132=DIRECTION('',(0.,1.,0.));
#44133=DIRECTION('center_axis',(1.,0.,0.));
#44134=DIRECTION('ref_axis',(0.,0.,-1.));
#44135=DIRECTION('',(-1.,0.,0.));
#44136=DIRECTION('',(-1.,0.,0.));
#44137=DIRECTION('',(1.,-1.42247325030098E-14,4.44089209850062E-14));
#44138=DIRECTION('',(1.,-1.42247325030098E-14,4.44089209850062E-14));
#44139=DIRECTION('center_axis',(0.,0.,-1.));
#44140=DIRECTION('ref_axis',(-1.,0.,0.));
#44141=DIRECTION('center_axis',(0.,0.,-1.));
#44142=DIRECTION('ref_axis',(-1.,0.,0.));
#44143=DIRECTION('center_axis',(-6.12323399573677E-17,1.,0.));
#44144=DIRECTION('ref_axis',(0.,0.,1.));
#44145=DIRECTION('',(1.,6.12323399573677E-17,0.));
#44146=DIRECTION('',(1.,6.12323399573677E-17,0.));
#44147=DIRECTION('center_axis',(0.,0.,-1.));
#44148=DIRECTION('ref_axis',(-1.,0.,0.));
#44149=DIRECTION('',(1.,0.,0.));
#44150=DIRECTION('center_axis',(0.,1.,0.));
#44151=DIRECTION('ref_axis',(0.,0.,1.));
#44152=DIRECTION('',(-1.,0.,0.));
#44153=DIRECTION('',(1.,0.,0.));
#44154=DIRECTION('center_axis',(0.,0.,1.));
#44155=DIRECTION('ref_axis',(1.,0.,0.));
#44156=DIRECTION('',(-1.,0.,0.));
#44157=DIRECTION('',(-1.,-6.12323399573677E-17,0.));
#44158=DIRECTION('center_axis',(-6.12323399573677E-17,1.,0.));
#44159=DIRECTION('ref_axis',(0.,0.,1.));
#44160=DIRECTION('',(1.,6.12323399573677E-17,0.));
#44161=DIRECTION('center_axis',(1.,6.12323399573677E-17,0.));
#44162=DIRECTION('ref_axis',(0.,0.,1.));
#44163=DIRECTION('center_axis',(1.,6.12323399573677E-17,0.));
#44164=DIRECTION('ref_axis',(0.,0.,1.));
#44165=DIRECTION('',(-1.,0.,1.11022302462514E-14));
#44166=DIRECTION('',(-1.,0.,1.11022302462514E-14));
#44167=DIRECTION('',(1.,-1.73472347597679E-15,1.11022302462514E-14));
#44168=DIRECTION('',(1.,-1.73472347597679E-15,1.11022302462514E-14));
#44169=DIRECTION('center_axis',(0.,0.,1.));
#44170=DIRECTION('ref_axis',(1.,0.,0.));
#44171=DIRECTION('center_axis',(0.,0.,1.));
#44172=DIRECTION('ref_axis',(1.,0.,0.));
#44173=DIRECTION('center_axis',(-8.82055185704388E-15,1.,0.));
#44174=DIRECTION('ref_axis',(0.,0.,-1.));
#44175=DIRECTION('',(1.,8.82055185704388E-15,0.));
#44176=DIRECTION('',(-1.,-8.82055185704388E-15,0.));
#44177=DIRECTION('center_axis',(0.,0.,-1.));
#44178=DIRECTION('ref_axis',(-1.,0.,0.));
#44179=DIRECTION('',(-1.,0.,0.));
#44180=DIRECTION('center_axis',(0.,1.,0.));
#44181=DIRECTION('ref_axis',(0.,0.,1.));
#44182=DIRECTION('',(-1.,0.,0.));
#44183=DIRECTION('',(1.,0.,0.));
#44184=DIRECTION('center_axis',(0.,0.,-1.));
#44185=DIRECTION('ref_axis',(-1.,0.,0.));
#44186=DIRECTION('',(1.,0.,0.));
#44187=DIRECTION('',(1.,8.82055185704388E-15,0.));
#44188=DIRECTION('center_axis',(-8.82055185704388E-15,1.,0.));
#44189=DIRECTION('ref_axis',(0.,0.,-1.));
#44190=DIRECTION('',(-1.,-8.82055185704388E-15,0.));
#44191=DIRECTION('center_axis',(-1.,-8.82055185704388E-15,0.));
#44192=DIRECTION('ref_axis',(0.,0.,1.));
#44193=DIRECTION('center_axis',(-1.,-8.82055185704388E-15,0.));
#44194=DIRECTION('ref_axis',(0.,0.,1.));
#44195=DIRECTION('center_axis',(0.,0.,1.));
#44196=DIRECTION('ref_axis',(1.,0.,0.));
#44197=DIRECTION('center_axis',(0.,0.,1.));
#44198=DIRECTION('ref_axis',(1.,0.,0.));
#44199=DIRECTION('center_axis',(0.,0.,1.));
#44200=DIRECTION('ref_axis',(1.,0.,0.));
#44201=DIRECTION('center_axis',(0.,0.,1.));
#44202=DIRECTION('ref_axis',(1.,0.,0.));
#44203=DIRECTION('center_axis',(0.,0.,-1.));
#44204=DIRECTION('ref_axis',(1.,-8.67361737988403E-16,0.));
#44205=DIRECTION('center_axis',(0.,0.,-1.));
#44206=DIRECTION('ref_axis',(1.,8.67361737988403E-16,0.));
#44207=DIRECTION('center_axis',(0.,0.,1.));
#44208=DIRECTION('ref_axis',(1.,0.,0.));
#44209=DIRECTION('center_axis',(0.,0.,1.));
#44210=DIRECTION('ref_axis',(1.,0.,0.));
#44211=DIRECTION('',(0.,0.,1.));
#44212=DIRECTION('center_axis',(0.,0.,-1.));
#44213=DIRECTION('ref_axis',(1.,8.67361737988403E-16,0.));
#44214=DIRECTION('center_axis',(0.,0.,1.));
#44215=DIRECTION('ref_axis',(1.,0.,0.));
#44216=DIRECTION('center_axis',(0.,0.,-1.));
#44217=DIRECTION('ref_axis',(1.,-3.18755438710738E-14,0.));
#44218=DIRECTION('',(0.,0.,-1.));
#44219=DIRECTION('center_axis',(0.,0.,1.));
#44220=DIRECTION('ref_axis',(1.,0.,0.));
#44221=DIRECTION('center_axis',(0.,0.,-1.));
#44222=DIRECTION('ref_axis',(-1.,0.,0.));
#44223=DIRECTION('center_axis',(0.,0.,-1.));
#44224=DIRECTION('ref_axis',(1.,-7.2280144832367E-16,0.));
#44225=DIRECTION('',(-0.42443387623072,-0.905458935958868,0.));
#44226=DIRECTION('center_axis',(0.,0.,1.));
#44227=DIRECTION('ref_axis',(1.,0.,0.));
#44228=DIRECTION('',(-1.,0.,0.));
#44229=DIRECTION('center_axis',(0.,0.,1.));
#44230=DIRECTION('ref_axis',(1.,0.,0.));
#44231=DIRECTION('',(-0.42443387623072,0.905458935958868,0.));
#44232=DIRECTION('center_axis',(0.,0.,-1.));
#44233=DIRECTION('ref_axis',(1.,-3.61400724161833E-15,0.));
#44234=DIRECTION('',(-0.424433876230721,0.905458935958868,0.));
#44235=DIRECTION('center_axis',(0.,0.,1.));
#44236=DIRECTION('ref_axis',(1.,0.,0.));
#44237=DIRECTION('',(-1.,0.,0.));
#44238=DIRECTION('center_axis',(0.,0.,1.));
#44239=DIRECTION('ref_axis',(1.,0.,0.));
#44240=DIRECTION('',(-0.424433876230721,-0.905458935958868,0.));
#44241=DIRECTION('center_axis',(0.,0.,-1.));
#44242=DIRECTION('ref_axis',(-0.42443387623072,-0.905458935958868,0.));
#44243=DIRECTION('center_axis',(0.,0.,1.));
#44244=DIRECTION('ref_axis',(1.,0.,0.));
#44245=DIRECTION('',(-0.42443387623072,0.905458935958868,0.));
#44246=DIRECTION('center_axis',(0.,0.,-1.));
#44247=DIRECTION('ref_axis',(1.,1.15648231731787E-14,0.));
#44248=DIRECTION('',(-1.,0.,0.));
#44249=DIRECTION('center_axis',(0.,0.,-1.));
#44250=DIRECTION('ref_axis',(1.,-1.73472347597681E-15,0.));
#44251=DIRECTION('',(-0.42443387623072,-0.905458935958868,0.));
#44252=DIRECTION('center_axis',(0.,0.,1.));
#44253=DIRECTION('ref_axis',(1.,0.,0.));
#44254=DIRECTION('',(-0.424433876230721,-0.905458935958868,0.));
#44255=DIRECTION('center_axis',(0.,0.,-1.));
#44256=DIRECTION('ref_axis',(1.,0.,0.));
#44257=DIRECTION('',(-1.,0.,0.));
#44258=DIRECTION('center_axis',(0.,0.,-1.));
#44259=DIRECTION('ref_axis',(1.,1.69701209606427E-15,0.));
#44260=DIRECTION('',(-0.42443387623072,0.905458935958868,0.));
#44261=DIRECTION('center_axis',(0.,0.,1.));
#44262=DIRECTION('ref_axis',(1.,0.,0.));
#44263=DIRECTION('',(0.,0.,1.));
#44264=DIRECTION('',(0.,0.,-1.));
#44265=DIRECTION('center_axis',(0.,0.,1.));
#44266=DIRECTION('ref_axis',(1.,0.,0.));
#44267=DIRECTION('',(0.,0.,1.));
#44268=DIRECTION('',(0.,0.,-1.));
#44269=DIRECTION('center_axis',(-0.905458935958868,0.42443387623072,0.));
#44270=DIRECTION('ref_axis',(-0.42443387623072,-0.905458935958868,0.));
#44271=DIRECTION('center_axis',(0.905458935958868,0.42443387623072,0.));
#44272=DIRECTION('ref_axis',(-0.42443387623072,0.905458935958868,0.));
#44273=DIRECTION('center_axis',(0.,1.,0.));
#44274=DIRECTION('ref_axis',(0.,0.,1.));
#44275=DIRECTION('center_axis',(0.,0.,1.));
#44276=DIRECTION('ref_axis',(1.,0.,0.));
#44277=DIRECTION('',(0.,0.,-1.));
#44278=DIRECTION('',(0.,0.,1.));
#44279=DIRECTION('center_axis',(0.,0.,1.));
#44280=DIRECTION('ref_axis',(1.,0.,0.));
#44281=DIRECTION('',(0.,0.,-1.));
#44282=DIRECTION('',(0.,0.,1.));
#44283=DIRECTION('center_axis',(0.,0.,1.));
#44284=DIRECTION('ref_axis',(1.,0.,0.));
#44285=DIRECTION('',(0.,0.,-1.));
#44286=DIRECTION('center_axis',(0.,0.,1.));
#44287=DIRECTION('ref_axis',(1.,0.,0.));
#44288=DIRECTION('',(0.,0.,1.));
#44289=DIRECTION('center_axis',(-0.905458935958868,0.42443387623072,0.));
#44290=DIRECTION('ref_axis',(-0.42443387623072,-0.905458935958868,0.));
#44291=DIRECTION('center_axis',(0.905458935958868,0.42443387623072,0.));
#44292=DIRECTION('ref_axis',(-0.42443387623072,0.905458935958868,0.));
#44293=DIRECTION('center_axis',(0.,1.,0.));
#44294=DIRECTION('ref_axis',(0.,0.,1.));
#44295=DIRECTION('center_axis',(0.,0.,1.));
#44296=DIRECTION('ref_axis',(1.,0.,0.));
#44297=DIRECTION('center_axis',(0.,0.,1.));
#44298=DIRECTION('ref_axis',(1.,0.,0.));
#44299=DIRECTION('center_axis',(0.,0.,1.));
#44300=DIRECTION('ref_axis',(1.,0.,0.));
#44301=DIRECTION('center_axis',(0.,0.,1.));
#44302=DIRECTION('ref_axis',(1.,0.,0.));
#44303=DIRECTION('center_axis',(0.,0.,-1.));
#44304=DIRECTION('ref_axis',(1.,-8.67361737988403E-16,0.));
#44305=DIRECTION('center_axis',(0.,0.,-1.));
#44306=DIRECTION('ref_axis',(1.,8.67361737988403E-16,0.));
#44307=DIRECTION('center_axis',(0.,0.,1.));
#44308=DIRECTION('ref_axis',(1.,0.,0.));
#44309=DIRECTION('center_axis',(0.,0.,1.));
#44310=DIRECTION('ref_axis',(1.,0.,0.));
#44311=DIRECTION('',(0.,0.,1.));
#44312=DIRECTION('center_axis',(0.,0.,-1.));
#44313=DIRECTION('ref_axis',(1.,8.67361737988403E-16,0.));
#44314=DIRECTION('center_axis',(0.,0.,1.));
#44315=DIRECTION('ref_axis',(1.,0.,0.));
#44316=DIRECTION('center_axis',(0.,0.,-1.));
#44317=DIRECTION('ref_axis',(1.,-3.18755438710738E-14,0.));
#44318=DIRECTION('',(0.,0.,-1.));
#44319=DIRECTION('center_axis',(0.,0.,1.));
#44320=DIRECTION('ref_axis',(1.,0.,0.));
#44321=DIRECTION('center_axis',(0.,0.,-1.));
#44322=DIRECTION('ref_axis',(-1.,0.,0.));
#44323=DIRECTION('center_axis',(0.,0.,-1.));
#44324=DIRECTION('ref_axis',(1.,-7.2280144832367E-16,0.));
#44325=DIRECTION('',(-0.42443387623072,-0.905458935958868,0.));
#44326=DIRECTION('center_axis',(0.,0.,1.));
#44327=DIRECTION('ref_axis',(1.,0.,0.));
#44328=DIRECTION('',(-1.,0.,0.));
#44329=DIRECTION('center_axis',(0.,0.,1.));
#44330=DIRECTION('ref_axis',(1.,0.,0.));
#44331=DIRECTION('',(-0.42443387623072,0.905458935958868,0.));
#44332=DIRECTION('center_axis',(0.,0.,-1.));
#44333=DIRECTION('ref_axis',(1.,-3.61400724161833E-15,0.));
#44334=DIRECTION('',(-0.424433876230721,0.905458935958868,0.));
#44335=DIRECTION('center_axis',(0.,0.,1.));
#44336=DIRECTION('ref_axis',(1.,0.,0.));
#44337=DIRECTION('',(-1.,0.,0.));
#44338=DIRECTION('center_axis',(0.,0.,1.));
#44339=DIRECTION('ref_axis',(1.,0.,0.));
#44340=DIRECTION('',(-0.424433876230721,-0.905458935958868,0.));
#44341=DIRECTION('center_axis',(0.,0.,-1.));
#44342=DIRECTION('ref_axis',(-0.42443387623072,-0.905458935958868,0.));
#44343=DIRECTION('center_axis',(0.,0.,1.));
#44344=DIRECTION('ref_axis',(1.,0.,0.));
#44345=DIRECTION('',(-0.42443387623072,0.905458935958868,0.));
#44346=DIRECTION('center_axis',(0.,0.,-1.));
#44347=DIRECTION('ref_axis',(1.,1.15648231731787E-14,0.));
#44348=DIRECTION('',(-1.,0.,0.));
#44349=DIRECTION('center_axis',(0.,0.,-1.));
#44350=DIRECTION('ref_axis',(1.,-1.73472347597681E-15,0.));
#44351=DIRECTION('',(-0.42443387623072,-0.905458935958868,0.));
#44352=DIRECTION('center_axis',(0.,0.,1.));
#44353=DIRECTION('ref_axis',(1.,0.,0.));
#44354=DIRECTION('',(-0.424433876230721,-0.905458935958868,0.));
#44355=DIRECTION('center_axis',(0.,0.,-1.));
#44356=DIRECTION('ref_axis',(1.,0.,0.));
#44357=DIRECTION('',(-1.,0.,0.));
#44358=DIRECTION('center_axis',(0.,0.,-1.));
#44359=DIRECTION('ref_axis',(1.,1.69701209606427E-15,0.));
#44360=DIRECTION('',(-0.42443387623072,0.905458935958868,0.));
#44361=DIRECTION('center_axis',(0.,0.,1.));
#44362=DIRECTION('ref_axis',(1.,0.,0.));
#44363=DIRECTION('',(0.,0.,1.));
#44364=DIRECTION('',(0.,0.,-1.));
#44365=DIRECTION('center_axis',(0.,0.,1.));
#44366=DIRECTION('ref_axis',(1.,0.,0.));
#44367=DIRECTION('',(0.,0.,1.));
#44368=DIRECTION('',(0.,0.,-1.));
#44369=DIRECTION('center_axis',(-0.905458935958868,0.42443387623072,0.));
#44370=DIRECTION('ref_axis',(-0.42443387623072,-0.905458935958868,0.));
#44371=DIRECTION('center_axis',(0.905458935958868,0.42443387623072,0.));
#44372=DIRECTION('ref_axis',(-0.42443387623072,0.905458935958868,0.));
#44373=DIRECTION('center_axis',(0.,1.,0.));
#44374=DIRECTION('ref_axis',(0.,0.,1.));
#44375=DIRECTION('center_axis',(0.,0.,1.));
#44376=DIRECTION('ref_axis',(1.,0.,0.));
#44377=DIRECTION('',(0.,0.,-1.));
#44378=DIRECTION('',(0.,0.,1.));
#44379=DIRECTION('center_axis',(0.,0.,1.));
#44380=DIRECTION('ref_axis',(1.,0.,0.));
#44381=DIRECTION('',(0.,0.,-1.));
#44382=DIRECTION('',(0.,0.,1.));
#44383=DIRECTION('center_axis',(0.,0.,1.));
#44384=DIRECTION('ref_axis',(1.,0.,0.));
#44385=DIRECTION('',(0.,0.,-1.));
#44386=DIRECTION('center_axis',(0.,0.,1.));
#44387=DIRECTION('ref_axis',(1.,0.,0.));
#44388=DIRECTION('',(0.,0.,1.));
#44389=DIRECTION('center_axis',(-0.905458935958868,0.42443387623072,0.));
#44390=DIRECTION('ref_axis',(-0.42443387623072,-0.905458935958868,0.));
#44391=DIRECTION('center_axis',(0.905458935958868,0.42443387623072,0.));
#44392=DIRECTION('ref_axis',(-0.42443387623072,0.905458935958868,0.));
#44393=DIRECTION('center_axis',(0.,1.,0.));
#44394=DIRECTION('ref_axis',(0.,0.,1.));
#44395=DIRECTION('center_axis',(0.,0.,1.));
#44396=DIRECTION('ref_axis',(1.,0.,0.));
#44397=DIRECTION('center_axis',(0.,0.,1.));
#44398=DIRECTION('ref_axis',(1.,0.,0.));
#44399=DIRECTION('center_axis',(0.,0.,1.));
#44400=DIRECTION('ref_axis',(1.,0.,0.));
#44401=DIRECTION('center_axis',(0.,0.,1.));
#44402=DIRECTION('ref_axis',(1.,0.,0.));
#44403=DIRECTION('center_axis',(0.,0.,-1.));
#44404=DIRECTION('ref_axis',(1.,0.,0.));
#44405=DIRECTION('center_axis',(0.,0.,-1.));
#44406=DIRECTION('ref_axis',(1.,8.67361737988403E-16,0.));
#44407=DIRECTION('center_axis',(0.,0.,1.));
#44408=DIRECTION('ref_axis',(1.,0.,0.));
#44409=DIRECTION('center_axis',(0.,0.,1.));
#44410=DIRECTION('ref_axis',(1.,0.,0.));
#44411=DIRECTION('',(0.,0.,1.));
#44412=DIRECTION('center_axis',(0.,0.,-1.));
#44413=DIRECTION('ref_axis',(1.,8.67361737988403E-16,0.));
#44414=DIRECTION('center_axis',(0.,0.,1.));
#44415=DIRECTION('ref_axis',(1.,0.,0.));
#44416=DIRECTION('center_axis',(0.,0.,-1.));
#44417=DIRECTION('ref_axis',(1.,0.,0.));
#44418=DIRECTION('',(0.,0.,-1.));
#44419=DIRECTION('center_axis',(0.,0.,1.));
#44420=DIRECTION('ref_axis',(1.,0.,0.));
#44421=DIRECTION('center_axis',(0.,0.,-1.));
#44422=DIRECTION('ref_axis',(-1.,0.,0.));
#44423=DIRECTION('center_axis',(0.,0.,-1.));
#44424=DIRECTION('ref_axis',(1.,-7.2280144832367E-16,0.));
#44425=DIRECTION('',(-0.42443387623072,-0.905458935958868,0.));
#44426=DIRECTION('center_axis',(0.,0.,1.));
#44427=DIRECTION('ref_axis',(1.,0.,0.));
#44428=DIRECTION('',(-1.,0.,0.));
#44429=DIRECTION('center_axis',(0.,0.,1.));
#44430=DIRECTION('ref_axis',(1.,0.,0.));
#44431=DIRECTION('',(-0.42443387623072,0.905458935958868,0.));
#44432=DIRECTION('center_axis',(0.,0.,-1.));
#44433=DIRECTION('ref_axis',(1.,-7.2280144832367E-16,0.));
#44434=DIRECTION('',(-0.424433876230721,0.905458935958868,0.));
#44435=DIRECTION('center_axis',(0.,0.,1.));
#44436=DIRECTION('ref_axis',(1.,0.,0.));
#44437=DIRECTION('',(-1.,0.,0.));
#44438=DIRECTION('center_axis',(0.,0.,1.));
#44439=DIRECTION('ref_axis',(1.,0.,0.));
#44440=DIRECTION('',(-0.424433876230721,-0.905458935958868,0.));
#44441=DIRECTION('center_axis',(0.,0.,-1.));
#44442=DIRECTION('ref_axis',(-0.42443387623072,-0.905458935958868,0.));
#44443=DIRECTION('center_axis',(0.,0.,1.));
#44444=DIRECTION('ref_axis',(1.,0.,0.));
#44445=DIRECTION('',(-0.42443387623072,0.905458935958868,0.));
#44446=DIRECTION('center_axis',(0.,0.,-1.));
#44447=DIRECTION('ref_axis',(1.,0.,0.));
#44448=DIRECTION('',(-1.,0.,0.));
#44449=DIRECTION('center_axis',(0.,0.,-1.));
#44450=DIRECTION('ref_axis',(1.,-1.73472347597681E-15,0.));
#44451=DIRECTION('',(-0.42443387623072,-0.905458935958868,0.));
#44452=DIRECTION('center_axis',(0.,0.,1.));
#44453=DIRECTION('ref_axis',(1.,0.,0.));
#44454=DIRECTION('',(-0.424433876230721,-0.905458935958868,0.));
#44455=DIRECTION('center_axis',(0.,0.,-1.));
#44456=DIRECTION('ref_axis',(1.,0.,0.));
#44457=DIRECTION('',(-1.,0.,0.));
#44458=DIRECTION('center_axis',(0.,0.,-1.));
#44459=DIRECTION('ref_axis',(1.,1.69701209606427E-15,0.));
#44460=DIRECTION('',(-0.424433876230721,0.905458935958868,0.));
#44461=DIRECTION('center_axis',(0.,0.,1.));
#44462=DIRECTION('ref_axis',(1.,0.,0.));
#44463=DIRECTION('',(0.,0.,1.));
#44464=DIRECTION('',(0.,0.,-1.));
#44465=DIRECTION('center_axis',(0.,0.,1.));
#44466=DIRECTION('ref_axis',(1.,0.,0.));
#44467=DIRECTION('',(0.,0.,1.));
#44468=DIRECTION('',(0.,0.,-1.));
#44469=DIRECTION('center_axis',(-0.905458935958868,0.42443387623072,0.));
#44470=DIRECTION('ref_axis',(-0.42443387623072,-0.905458935958868,0.));
#44471=DIRECTION('center_axis',(0.905458935958868,0.42443387623072,0.));
#44472=DIRECTION('ref_axis',(-0.42443387623072,0.905458935958868,0.));
#44473=DIRECTION('center_axis',(0.,1.,0.));
#44474=DIRECTION('ref_axis',(0.,0.,1.));
#44475=DIRECTION('center_axis',(0.,0.,1.));
#44476=DIRECTION('ref_axis',(1.,0.,0.));
#44477=DIRECTION('',(0.,0.,-1.));
#44478=DIRECTION('',(0.,0.,1.));
#44479=DIRECTION('center_axis',(0.,0.,1.));
#44480=DIRECTION('ref_axis',(1.,0.,0.));
#44481=DIRECTION('',(0.,0.,-1.));
#44482=DIRECTION('',(0.,0.,1.));
#44483=DIRECTION('center_axis',(0.,0.,1.));
#44484=DIRECTION('ref_axis',(1.,0.,0.));
#44485=DIRECTION('',(0.,0.,-1.));
#44486=DIRECTION('center_axis',(0.,0.,1.));
#44487=DIRECTION('ref_axis',(1.,0.,0.));
#44488=DIRECTION('',(0.,0.,1.));
#44489=DIRECTION('center_axis',(-0.905458935958868,0.42443387623072,0.));
#44490=DIRECTION('ref_axis',(-0.42443387623072,-0.905458935958868,0.));
#44491=DIRECTION('center_axis',(0.905458935958868,0.42443387623072,0.));
#44492=DIRECTION('ref_axis',(-0.42443387623072,0.905458935958868,0.));
#44493=DIRECTION('center_axis',(0.,1.,0.));
#44494=DIRECTION('ref_axis',(0.,0.,1.));
#44495=DIRECTION('center_axis',(0.,0.,1.));
#44496=DIRECTION('ref_axis',(1.,0.,0.));
#44497=DIRECTION('center_axis',(0.,0.,1.));
#44498=DIRECTION('ref_axis',(1.,0.,0.));
#44499=DIRECTION('center_axis',(0.,0.,1.));
#44500=DIRECTION('ref_axis',(1.,0.,0.));
#44501=DIRECTION('center_axis',(0.,0.,1.));
#44502=DIRECTION('ref_axis',(1.,0.,0.));
#44503=DIRECTION('center_axis',(0.,0.,-1.));
#44504=DIRECTION('ref_axis',(1.,0.,0.));
#44505=DIRECTION('center_axis',(0.,0.,-1.));
#44506=DIRECTION('ref_axis',(1.,8.67361737988403E-16,0.));
#44507=DIRECTION('center_axis',(0.,0.,1.));
#44508=DIRECTION('ref_axis',(1.,0.,0.));
#44509=DIRECTION('center_axis',(0.,0.,1.));
#44510=DIRECTION('ref_axis',(1.,0.,0.));
#44511=DIRECTION('',(0.,0.,1.));
#44512=DIRECTION('center_axis',(0.,0.,-1.));
#44513=DIRECTION('ref_axis',(1.,8.67361737988403E-16,0.));
#44514=DIRECTION('center_axis',(0.,0.,1.));
#44515=DIRECTION('ref_axis',(1.,0.,0.));
#44516=DIRECTION('center_axis',(0.,0.,-1.));
#44517=DIRECTION('ref_axis',(1.,0.,0.));
#44518=DIRECTION('',(0.,0.,-1.));
#44519=DIRECTION('center_axis',(0.,0.,1.));
#44520=DIRECTION('ref_axis',(1.,0.,0.));
#44521=DIRECTION('center_axis',(0.,0.,-1.));
#44522=DIRECTION('ref_axis',(-1.,0.,0.));
#44523=DIRECTION('center_axis',(0.,0.,-1.));
#44524=DIRECTION('ref_axis',(1.,-7.2280144832367E-16,0.));
#44525=DIRECTION('',(-0.42443387623072,-0.905458935958868,0.));
#44526=DIRECTION('center_axis',(0.,0.,1.));
#44527=DIRECTION('ref_axis',(1.,0.,0.));
#44528=DIRECTION('',(-1.,0.,0.));
#44529=DIRECTION('center_axis',(0.,0.,1.));
#44530=DIRECTION('ref_axis',(1.,0.,0.));
#44531=DIRECTION('',(-0.42443387623072,0.905458935958868,0.));
#44532=DIRECTION('center_axis',(0.,0.,-1.));
#44533=DIRECTION('ref_axis',(1.,-7.2280144832367E-16,0.));
#44534=DIRECTION('',(-0.42443387623072,0.905458935958868,0.));
#44535=DIRECTION('center_axis',(0.,0.,1.));
#44536=DIRECTION('ref_axis',(1.,0.,0.));
#44537=DIRECTION('',(-1.,0.,0.));
#44538=DIRECTION('center_axis',(0.,0.,1.));
#44539=DIRECTION('ref_axis',(1.,0.,0.));
#44540=DIRECTION('',(-0.42443387623072,-0.905458935958868,0.));
#44541=DIRECTION('center_axis',(0.,0.,-1.));
#44542=DIRECTION('ref_axis',(-0.42443387623072,-0.905458935958868,0.));
#44543=DIRECTION('center_axis',(0.,0.,1.));
#44544=DIRECTION('ref_axis',(1.,0.,0.));
#44545=DIRECTION('',(-0.42443387623072,0.905458935958868,0.));
#44546=DIRECTION('center_axis',(0.,0.,-1.));
#44547=DIRECTION('ref_axis',(1.,0.,0.));
#44548=DIRECTION('',(-1.,0.,0.));
#44549=DIRECTION('center_axis',(0.,0.,-1.));
#44550=DIRECTION('ref_axis',(1.,-1.73472347597681E-15,0.));
#44551=DIRECTION('',(-0.42443387623072,-0.905458935958868,0.));
#44552=DIRECTION('center_axis',(0.,0.,1.));
#44553=DIRECTION('ref_axis',(1.,0.,0.));
#44554=DIRECTION('',(-0.42443387623072,-0.905458935958868,0.));
#44555=DIRECTION('center_axis',(0.,0.,-1.));
#44556=DIRECTION('ref_axis',(1.,0.,0.));
#44557=DIRECTION('',(-1.,0.,0.));
#44558=DIRECTION('center_axis',(0.,0.,-1.));
#44559=DIRECTION('ref_axis',(1.,1.69701209606427E-15,0.));
#44560=DIRECTION('',(-0.42443387623072,0.905458935958868,0.));
#44561=DIRECTION('center_axis',(0.,0.,1.));
#44562=DIRECTION('ref_axis',(1.,0.,0.));
#44563=DIRECTION('',(0.,0.,1.));
#44564=DIRECTION('',(0.,0.,-1.));
#44565=DIRECTION('center_axis',(0.,0.,1.));
#44566=DIRECTION('ref_axis',(1.,0.,0.));
#44567=DIRECTION('',(0.,0.,1.));
#44568=DIRECTION('',(0.,0.,-1.));
#44569=DIRECTION('center_axis',(-0.905458935958868,0.42443387623072,0.));
#44570=DIRECTION('ref_axis',(-0.42443387623072,-0.905458935958868,0.));
#44571=DIRECTION('center_axis',(0.905458935958868,0.42443387623072,0.));
#44572=DIRECTION('ref_axis',(-0.42443387623072,0.905458935958868,0.));
#44573=DIRECTION('center_axis',(0.,1.,0.));
#44574=DIRECTION('ref_axis',(0.,0.,1.));
#44575=DIRECTION('center_axis',(0.,0.,1.));
#44576=DIRECTION('ref_axis',(1.,0.,0.));
#44577=DIRECTION('',(0.,0.,-1.));
#44578=DIRECTION('',(0.,0.,1.));
#44579=DIRECTION('center_axis',(0.,0.,1.));
#44580=DIRECTION('ref_axis',(1.,0.,0.));
#44581=DIRECTION('',(0.,0.,-1.));
#44582=DIRECTION('',(0.,0.,1.));
#44583=DIRECTION('center_axis',(0.,0.,1.));
#44584=DIRECTION('ref_axis',(1.,0.,0.));
#44585=DIRECTION('',(0.,0.,-1.));
#44586=DIRECTION('center_axis',(0.,0.,1.));
#44587=DIRECTION('ref_axis',(1.,0.,0.));
#44588=DIRECTION('',(0.,0.,1.));
#44589=DIRECTION('center_axis',(-0.905458935958868,0.42443387623072,0.));
#44590=DIRECTION('ref_axis',(-0.42443387623072,-0.905458935958868,0.));
#44591=DIRECTION('center_axis',(0.905458935958868,0.42443387623072,0.));
#44592=DIRECTION('ref_axis',(-0.42443387623072,0.905458935958868,0.));
#44593=DIRECTION('center_axis',(0.,1.,0.));
#44594=DIRECTION('ref_axis',(0.,0.,1.));
#44595=DIRECTION('center_axis',(-1.,-4.38245930773088E-16,0.));
#44596=DIRECTION('ref_axis',(0.,0.,1.));
#44597=DIRECTION('center_axis',(1.,4.38245930773088E-16,0.));
#44598=DIRECTION('ref_axis',(4.38245930773088E-16,-1.,0.));
#44599=DIRECTION('center_axis',(1.,4.38245930773088E-16,0.));
#44600=DIRECTION('ref_axis',(4.38245930773088E-16,-1.,0.));
#44601=DIRECTION('',(-3.46944695195361E-16,0.5,0.866025403784438));
#44602=DIRECTION('center_axis',(1.,4.38245930773088E-16,0.));
#44603=DIRECTION('ref_axis',(4.38245930773088E-16,-1.,2.31296463463574E-15));
#44604=DIRECTION('center_axis',(1.,4.38245930773088E-16,0.));
#44605=DIRECTION('ref_axis',(4.38245930773088E-16,-1.,2.31296463463574E-15));
#44606=DIRECTION('',(3.46944695195361E-16,-0.5,-0.866025403784438));
#44607=DIRECTION('center_axis',(1.,4.38245930773088E-16,0.));
#44608=DIRECTION('ref_axis',(4.38245930773088E-16,-1.,0.));
#44609=DIRECTION('',(-4.38245930773088E-16,1.,0.));
#44610=DIRECTION('center_axis',(1.,4.38245930773088E-16,0.));
#44611=DIRECTION('ref_axis',(4.38245930773088E-16,-1.,0.));
#44612=DIRECTION('center_axis',(1.,4.38245930773088E-16,0.));
#44613=DIRECTION('ref_axis',(4.38245930773088E-16,-1.,0.));
#44614=DIRECTION('',(4.38245930773088E-16,-1.,0.));
#44615=DIRECTION('center_axis',(1.,4.38245930773088E-16,0.));
#44616=DIRECTION('ref_axis',(4.38245930773088E-16,-1.,0.));
#44617=DIRECTION('',(-3.46944695195361E-16,0.499999999999999,-0.866025403784439));
#44618=DIRECTION('center_axis',(1.,4.38245930773088E-16,0.));
#44619=DIRECTION('ref_axis',(4.38245930773088E-16,-1.,0.));
#44620=DIRECTION('center_axis',(1.,4.38245930773088E-16,0.));
#44621=DIRECTION('ref_axis',(4.38245930773088E-16,-1.,0.));
#44622=DIRECTION('',(3.46944695195362E-16,-0.499999999999999,0.866025403784439));
#44623=DIRECTION('center_axis',(1.,4.38245930773088E-16,0.));
#44624=DIRECTION('ref_axis',(4.38245930773088E-16,-1.,4.62592926927148E-15));
#44625=DIRECTION('center_axis',(1.,4.38245930773088E-16,0.));
#44626=DIRECTION('ref_axis',(4.38245930773088E-16,-1.,-9.25185853854296E-15));
#44627=DIRECTION('',(0.,-0.5,-0.866025403784438));
#44628=DIRECTION('center_axis',(1.,4.38245930773088E-16,0.));
#44629=DIRECTION('ref_axis',(4.38245930773088E-16,-1.,0.));
#44630=DIRECTION('',(0.,0.5,0.866025403784438));
#44631=DIRECTION('center_axis',(1.,4.38245930773088E-16,0.));
#44632=DIRECTION('ref_axis',(4.38245930773088E-16,-1.,4.62592926927148E-15));
#44633=DIRECTION('center_axis',(1.,4.38245930773088E-16,0.));
#44634=DIRECTION('ref_axis',(4.38245930773088E-16,-1.,0.));
#44635=DIRECTION('',(4.38245930773088E-16,-1.,0.));
#44636=DIRECTION('',(-4.38245930773088E-16,1.,0.));
#44637=DIRECTION('center_axis',(1.,4.38245930773088E-16,0.));
#44638=DIRECTION('ref_axis',(4.38245930773088E-16,-1.,0.));
#44639=DIRECTION('center_axis',(1.,4.38245930773088E-16,0.));
#44640=DIRECTION('ref_axis',(4.38245930773088E-16,-1.,0.));
#44641=DIRECTION('',(0.,-0.5,0.866025403784439));
#44642=DIRECTION('center_axis',(1.,4.38245930773088E-16,0.));
#44643=DIRECTION('ref_axis',(4.38245930773088E-16,-1.,0.));
#44644=DIRECTION('center_axis',(1.,4.38245930773088E-16,0.));
#44645=DIRECTION('ref_axis',(4.38245930773088E-16,-1.,0.));
#44646=DIRECTION('center_axis',(1.,4.38245930773088E-16,0.));
#44647=DIRECTION('ref_axis',(4.38245930773088E-16,-1.,0.));
#44648=DIRECTION('center_axis',(1.,4.38245930773088E-16,0.));
#44649=DIRECTION('ref_axis',(4.38245930773088E-16,-1.,2.89120579329468E-15));
#44650=DIRECTION('center_axis',(1.,4.38245930773088E-16,0.));
#44651=DIRECTION('ref_axis',(4.38245930773088E-16,-1.,1.73472347597681E-15));
#44652=DIRECTION('center_axis',(1.,4.38245930773088E-16,0.));
#44653=DIRECTION('ref_axis',(4.38245930773088E-16,-1.,0.));
#44654=DIRECTION('center_axis',(1.,4.38245930773088E-16,0.));
#44655=DIRECTION('ref_axis',(4.38245930773088E-16,-1.,0.));
#44656=DIRECTION('center_axis',(1.,4.38245930773088E-16,0.));
#44657=DIRECTION('ref_axis',(4.38245930773088E-16,-1.,0.));
#44658=DIRECTION('center_axis',(1.,4.38245930773088E-16,0.));
#44659=DIRECTION('ref_axis',(4.38245930773088E-16,-1.,0.));
#44660=DIRECTION('center_axis',(1.,4.38245930773088E-16,0.));
#44661=DIRECTION('ref_axis',(4.38245930773088E-16,-1.,4.62592926927148E-15));
#44662=DIRECTION('center_axis',(1.,4.38245930773088E-16,0.));
#44663=DIRECTION('ref_axis',(4.38245930773088E-16,-1.,-4.62592926927148E-15));
#44664=DIRECTION('center_axis',(1.,4.38245930773088E-16,0.));
#44665=DIRECTION('ref_axis',(4.38245930773088E-16,-1.,0.));
#44666=DIRECTION('center_axis',(1.,4.38245930773088E-16,0.));
#44667=DIRECTION('ref_axis',(4.38245930773088E-16,-1.,-4.62592926927148E-15));
#44668=DIRECTION('center_axis',(1.,4.38245930773088E-16,0.));
#44669=DIRECTION('ref_axis',(4.38245930773088E-16,-1.,0.));
#44670=DIRECTION('center_axis',(1.,4.38245930773088E-16,0.));
#44671=DIRECTION('ref_axis',(4.38245930773088E-16,-1.,9.25185853854296E-15));
#44672=DIRECTION('center_axis',(1.,4.38245930773088E-16,0.));
#44673=DIRECTION('ref_axis',(4.38245930773088E-16,-1.,0.));
#44674=DIRECTION('center_axis',(1.,4.38245930773088E-16,0.));
#44675=DIRECTION('ref_axis',(4.38245930773088E-16,-1.,0.));
#44676=DIRECTION('center_axis',(1.,4.38245930773088E-16,0.));
#44677=DIRECTION('ref_axis',(4.38245930773088E-16,-1.,1.15648231731787E-15));
#44678=DIRECTION('center_axis',(1.,4.38245930773088E-16,0.));
#44679=DIRECTION('ref_axis',(4.38245930773088E-16,-1.,1.15648231731787E-15));
#44680=DIRECTION('center_axis',(1.,4.38245930773088E-16,0.));
#44681=DIRECTION('ref_axis',(4.38245930773088E-16,-1.,1.80700362080917E-15));
#44682=DIRECTION('center_axis',(1.,4.38245930773088E-16,0.));
#44683=DIRECTION('ref_axis',(4.38245930773088E-16,-1.,-8.67361737988403E-16));
#44684=DIRECTION('center_axis',(1.,4.38245930773088E-16,0.));
#44685=DIRECTION('ref_axis',(4.38245930773088E-16,-1.,6.36065274524829E-15));
#44686=DIRECTION('center_axis',(1.,4.38245930773088E-16,0.));
#44687=DIRECTION('ref_axis',(4.38245930773088E-16,-1.,8.67361737988403E-16));
#44688=DIRECTION('center_axis',(1.,4.38245930773088E-16,0.));
#44689=DIRECTION('ref_axis',(4.38245930773088E-16,-1.,0.));
#44690=DIRECTION('center_axis',(1.,4.38245930773088E-16,0.));
#44691=DIRECTION('ref_axis',(4.38245930773088E-16,-1.,0.));
#44692=DIRECTION('center_axis',(1.,4.38245930773088E-16,0.));
#44693=DIRECTION('ref_axis',(4.38245930773088E-16,-1.,0.));
#44694=DIRECTION('center_axis',(1.,4.38245930773088E-16,0.));
#44695=DIRECTION('ref_axis',(4.38245930773088E-16,-1.,0.));
#44696=DIRECTION('center_axis',(1.,4.38245930773088E-16,0.));
#44697=DIRECTION('ref_axis',(4.38245930773088E-16,-1.,4.62592926927148E-15));
#44698=DIRECTION('center_axis',(1.,4.38245930773088E-16,0.));
#44699=DIRECTION('ref_axis',(4.38245930773088E-16,-1.,0.));
#44700=DIRECTION('center_axis',(1.,4.38245930773088E-16,0.));
#44701=DIRECTION('ref_axis',(4.38245930773088E-16,-1.,4.62592926927148E-15));
#44702=DIRECTION('center_axis',(1.,4.38245930773088E-16,0.));
#44703=DIRECTION('ref_axis',(4.38245930773088E-16,-1.,9.25185853854296E-15));
#44704=DIRECTION('center_axis',(1.,4.38245930773088E-16,0.));
#44705=DIRECTION('ref_axis',(4.38245930773088E-16,-1.,-4.62592926927148E-15));
#44706=DIRECTION('center_axis',(1.,4.38245930773088E-16,0.));
#44707=DIRECTION('ref_axis',(4.38245930773088E-16,-1.,4.62592926927148E-15));
#44708=DIRECTION('center_axis',(1.,4.38245930773088E-16,0.));
#44709=DIRECTION('ref_axis',(4.38245930773088E-16,-1.,0.));
#44710=DIRECTION('center_axis',(1.,4.38245930773088E-16,0.));
#44711=DIRECTION('ref_axis',(4.38245930773088E-16,-1.,0.));
#44712=DIRECTION('center_axis',(1.,4.38245930773088E-16,0.));
#44713=DIRECTION('ref_axis',(4.38245930773088E-16,-1.,-1.73472347597681E-15));
#44714=DIRECTION('center_axis',(1.,4.38245930773088E-16,0.));
#44715=DIRECTION('ref_axis',(4.38245930773088E-16,-1.,-1.73472347597681E-15));
#44716=DIRECTION('',(1.,4.38245930773088E-16,0.));
#44717=DIRECTION('',(-1.,-4.38245930773088E-16,0.));
#44718=DIRECTION('center_axis',(-3.79532109154651E-16,0.866025403784439,
0.499999999999999));
#44719=DIRECTION('ref_axis',(-7.94699513894569E-33,-0.499999999999999,0.866025403784439));
#44720=DIRECTION('',(-1.,-4.38245930773088E-16,0.));
#44721=DIRECTION('center_axis',(3.79532109154651E-16,-0.866025403784439,
-0.499999999999999));
#44722=DIRECTION('ref_axis',(1.5326347767966E-32,0.499999999999999,-0.866025403784439));
#44723=DIRECTION('',(1.,4.38245930773088E-16,0.));
#44724=DIRECTION('',(-1.,-4.38245930773088E-16,0.));
#44725=DIRECTION('center_axis',(-3.79532109154651E-16,0.866025403784438,
-0.5));
#44726=DIRECTION('ref_axis',(1.94620289117031E-33,0.5,0.866025403784438));
#44727=DIRECTION('',(1.,4.38245930773088E-16,8.64002241377108E-33));
#44728=DIRECTION('center_axis',(3.79532109154651E-16,-0.866025403784438,
0.5));
#44729=DIRECTION('ref_axis',(-1.94620289117031E-33,-0.5,-0.866025403784438));
#44730=DIRECTION('',(1.,4.38245930773088E-16,8.64002241377108E-33));
#44731=DIRECTION('',(-1.,-4.38245930773088E-16,-8.64002241377108E-33));
#44732=DIRECTION('center_axis',(0.,0.,-1.));
#44733=DIRECTION('ref_axis',(-1.,0.,0.));
#44734=DIRECTION('',(1.,4.38245930773088E-16,0.));
#44735=DIRECTION('center_axis',(0.,0.,1.));
#44736=DIRECTION('ref_axis',(1.,0.,0.));
#44737=DIRECTION('',(-1.,-4.38245930773088E-16,0.));
#44738=DIRECTION('center_axis',(3.79532109154651E-16,-0.866025403784439,
-0.5));
#44739=DIRECTION('ref_axis',(-8.35245407460559E-33,0.5,-0.866025403784439));
#44740=DIRECTION('',(-1.,-4.38245930773088E-16,0.));
#44741=DIRECTION('',(1.,4.38245930773088E-16,0.));
#44742=DIRECTION('center_axis',(3.79532109154651E-16,-0.866025403784438,
0.5));
#44743=DIRECTION('ref_axis',(2.27057003969863E-32,-0.5,-0.866025403784438));
#44744=DIRECTION('',(-1.,-4.38245930773088E-16,0.));
#44745=DIRECTION('',(1.,4.38245930773088E-16,0.));
#44746=DIRECTION('center_axis',(-3.79532109154651E-16,0.866025403784439,
-0.5));
#44747=DIRECTION('ref_axis',(-1.08662994757006E-32,0.5,0.866025403784439));
#44748=DIRECTION('',(1.,4.38245930773088E-16,0.));
#44749=DIRECTION('center_axis',(0.,0.,1.));
#44750=DIRECTION('ref_axis',(1.,0.,0.));
#44751=DIRECTION('',(-1.,-4.38245930773088E-16,0.));
#44752=DIRECTION('',(1.,4.38245930773088E-16,0.));
#44753=DIRECTION('center_axis',(0.,0.,-1.));
#44754=DIRECTION('ref_axis',(-1.,0.,0.));
#44755=DIRECTION('',(-1.,-4.38245930773088E-16,0.));
#44756=DIRECTION('',(1.,4.38245930773088E-16,0.));
#44757=DIRECTION('',(-1.,-4.38245930773088E-16,0.));
#44758=DIRECTION('',(1.,4.38245930773088E-16,0.));
#44759=DIRECTION('',(1.,4.38245930773088E-16,0.));
#44760=DIRECTION('',(-1.,-4.38245930773088E-16,0.));
#44761=DIRECTION('',(1.,4.38245930773088E-16,0.));
#44762=DIRECTION('',(-1.,-4.38245930773088E-16,0.));
#44763=DIRECTION('',(-1.,-4.38245930773088E-16,0.));
#44764=DIRECTION('',(1.,4.38245930773088E-16,0.));
#44765=DIRECTION('',(1.,4.38245930773088E-16,0.));
#44766=DIRECTION('',(-1.,-4.38245930773088E-16,0.));
#44767=DIRECTION('',(-1.,-4.38245930773088E-16,0.));
#44768=DIRECTION('',(1.,4.38245930773088E-16,0.));
#44769=DIRECTION('',(-1.,-4.38245930773088E-16,0.));
#44770=DIRECTION('',(1.,4.38245930773088E-16,0.));
#44771=DIRECTION('',(-1.,-4.38245930773088E-16,0.));
#44772=DIRECTION('',(-1.,-4.38245930773088E-16,0.));
#44773=DIRECTION('',(-1.,-4.38245930773088E-16,0.));
#44774=DIRECTION('',(1.,4.38245930773088E-16,0.));
#44775=DIRECTION('',(1.,4.38245930773088E-16,0.));
#44776=DIRECTION('',(-1.,-4.38245930773088E-16,0.));
#44777=DIRECTION('',(1.,4.38245930773088E-16,0.));
#44778=DIRECTION('',(-1.,-4.38245930773088E-16,0.));
#44779=DIRECTION('',(-1.,-4.38245930773088E-16,0.));
#44780=DIRECTION('',(1.,4.38245930773088E-16,0.));
#44781=DIRECTION('',(1.,4.38245930773088E-16,0.));
#44782=DIRECTION('',(-1.,-4.38245930773088E-16,0.));
#44783=DIRECTION('',(-1.,-4.38245930773088E-16,0.));
#44784=DIRECTION('',(1.,4.38245930773088E-16,0.));
#44785=DIRECTION('',(-1.,-4.38245930773088E-16,0.));
#44786=DIRECTION('',(1.,4.38245930773088E-16,0.));
#44787=DIRECTION('',(-1.,-4.38245930773088E-16,0.));
#44788=DIRECTION('',(-1.,-4.38245930773088E-16,0.));
#44789=DIRECTION('',(1.,4.38245930773088E-16,0.));
#44790=DIRECTION('',(-1.,-4.38245930773088E-16,0.));
#44791=DIRECTION('',(-1.,-4.38245930773088E-16,0.));
#44792=DIRECTION('',(1.,4.38245930773088E-16,0.));
#44793=DIRECTION('',(-1.,-4.38245930773088E-16,0.));
#44794=DIRECTION('',(1.,4.38245930773088E-16,0.));
#44795=DIRECTION('',(-1.,-4.38245930773088E-16,0.));
#44796=DIRECTION('',(1.,4.38245930773088E-16,0.));
#44797=DIRECTION('',(-1.,-4.38245930773088E-16,0.));
#44798=DIRECTION('center_axis',(-1.,-4.38245930773088E-16,0.));
#44799=DIRECTION('ref_axis',(4.38245930773088E-16,-1.,0.));
#44800=DIRECTION('center_axis',(-1.,-4.38245930773088E-16,0.));
#44801=DIRECTION('ref_axis',(4.38245930773088E-16,-1.,0.));
#44802=DIRECTION('center_axis',(-1.,-4.38245930773088E-16,0.));
#44803=DIRECTION('ref_axis',(-3.3768778812357E-16,0.770544035692177,0.637386765676236));
#44804=DIRECTION('center_axis',(-1.,-4.38245930773088E-16,0.));
#44805=DIRECTION('ref_axis',(4.38245930773088E-16,-1.,0.));
#44806=DIRECTION('center_axis',(-1.,-4.38245930773088E-16,0.));
#44807=DIRECTION('ref_axis',(-3.26063191989391E-16,0.744018755437613,0.668158732306228));
#44808=DIRECTION('center_axis',(-1.,-4.38245930773088E-16,0.));
#44809=DIRECTION('ref_axis',(4.38245930773088E-16,-1.,0.));
#44810=DIRECTION('center_axis',(-1.,-4.38245930773088E-16,0.));
#44811=DIRECTION('ref_axis',(-4.18556581656484E-16,0.955072374358683,-0.296372670360928));
#44812=DIRECTION('center_axis',(-1.,-4.38245930773088E-16,0.));
#44813=DIRECTION('ref_axis',(4.38245930773088E-16,-1.,0.));
#44814=DIRECTION('center_axis',(-1.,-4.38245930773088E-16,0.));
#44815=DIRECTION('ref_axis',(4.38245930773088E-16,-1.,0.));
#44816=DIRECTION('center_axis',(-1.,-4.38245930773088E-16,0.));
#44817=DIRECTION('ref_axis',(-4.18556584246465E-16,0.955072380268563,0.296372651316112));
#44818=DIRECTION('center_axis',(-1.,-4.38245930773088E-16,0.));
#44819=DIRECTION('ref_axis',(4.38245930773088E-16,-1.,0.));
#44820=DIRECTION('center_axis',(-1.,-4.38245930773088E-16,0.));
#44821=DIRECTION('ref_axis',(-3.21714447165222E-16,0.734095685948987,-0.679046039581328));
#44822=DIRECTION('center_axis',(-1.,-4.38245930773088E-16,0.));
#44823=DIRECTION('ref_axis',(-3.21714455957828E-16,0.734095706012164,0.679046017891647));
#44824=DIRECTION('center_axis',(-1.,-4.38245930773088E-16,0.));
#44825=DIRECTION('ref_axis',(4.38245930773088E-16,-1.,0.));
#44826=DIRECTION('center_axis',(-1.,-4.38245930773088E-16,0.));
#44827=DIRECTION('ref_axis',(4.38245930773088E-16,-1.,0.));
#44828=DIRECTION('center_axis',(-1.,-4.38245930773088E-16,0.));
#44829=DIRECTION('ref_axis',(4.38245930773088E-16,-1.,0.));
#44830=DIRECTION('center_axis',(-1.,-4.38245930773088E-16,0.));
#44831=DIRECTION('ref_axis',(-4.27911362366366E-16,0.976418335731055,0.215887085413176));
#44832=DIRECTION('center_axis',(-1.,-4.38245930773088E-16,0.));
#44833=DIRECTION('ref_axis',(4.38245930773088E-16,-1.,0.));
#44834=DIRECTION('center_axis',(-1.,-4.38245930773088E-16,0.));
#44835=DIRECTION('ref_axis',(4.38245930773088E-16,-1.,0.));
#44836=DIRECTION('center_axis',(-1.,-4.38245930773088E-16,0.));
#44837=DIRECTION('ref_axis',(-4.27911362366367E-16,0.976418335731058,-0.215887085413164));
#44838=DIRECTION('center_axis',(-1.,-4.38245930773088E-16,0.));
#44839=DIRECTION('ref_axis',(4.38245930773088E-16,-1.,0.));
#44840=DIRECTION('center_axis',(-1.,-4.38245930773088E-16,0.));
#44841=DIRECTION('ref_axis',(4.38245930773088E-16,-1.,0.));
#44842=DIRECTION('center_axis',(-1.,-4.38245930773088E-16,0.));
#44843=DIRECTION('ref_axis',(4.38245930773088E-16,-1.,0.));
#44844=DIRECTION('center_axis',(-1.,-4.38245930773088E-16,0.));
#44845=DIRECTION('ref_axis',(-4.16621911423142E-16,0.950657797753421,-0.310241440769309));
#44846=DIRECTION('center_axis',(-1.,-4.38245930773088E-16,0.));
#44847=DIRECTION('ref_axis',(4.38245930773088E-16,-1.,0.));
#44848=DIRECTION('center_axis',(-1.,-4.38245930773088E-16,0.));
#44849=DIRECTION('ref_axis',(4.38245930773088E-16,-1.,0.));
#44850=DIRECTION('center_axis',(-1.,-4.38245930773088E-16,0.));
#44851=DIRECTION('ref_axis',(-4.16621911423141E-16,0.950657797753419,0.310241440769313));
#44852=DIRECTION('center_axis',(-1.,-4.38245930773088E-16,0.));
#44853=DIRECTION('ref_axis',(4.38245930773088E-16,-1.,0.));
#44854=DIRECTION('center_axis',(-1.,-4.38245930773088E-16,0.));
#44855=DIRECTION('ref_axis',(-3.26063191989868E-16,0.7440187554387,-0.668158732305017));
#44856=DIRECTION('center_axis',(-1.,-4.38245930773088E-16,0.));
#44857=DIRECTION('ref_axis',(4.38245930773088E-16,-1.,0.));
#44858=DIRECTION('center_axis',(-1.,-4.38245930773088E-16,0.));
#44859=DIRECTION('ref_axis',(4.38245930773088E-16,-1.,0.));
#44860=DIRECTION('center_axis',(-1.,-4.38245930773088E-16,0.));
#44861=DIRECTION('ref_axis',(4.38245930773088E-16,-1.,0.));
#44862=DIRECTION('center_axis',(-1.,-4.38245930773088E-16,0.));
#44863=DIRECTION('ref_axis',(-4.30076690142246E-16,0.981359232209114,0.192182354439575));
#44864=DIRECTION('center_axis',(-1.,-4.38245930773088E-16,0.));
#44865=DIRECTION('ref_axis',(4.38245930773088E-16,-1.,0.));
#44866=DIRECTION('center_axis',(-1.,-4.38245930773088E-16,0.));
#44867=DIRECTION('ref_axis',(4.38245930773088E-16,-1.,0.));
#44868=DIRECTION('center_axis',(-1.,-4.38245930773088E-16,0.));
#44869=DIRECTION('ref_axis',(-4.30076690142246E-16,0.981359232209114,-0.192182354439576));
#44870=DIRECTION('center_axis',(-1.,-4.38245930773088E-16,0.));
#44871=DIRECTION('ref_axis',(4.38245930773088E-16,-1.,0.));
#44872=DIRECTION('center_axis',(-1.,-4.38245930773088E-16,0.));
#44873=DIRECTION('ref_axis',(4.38245930773088E-16,-1.,0.));
#44874=DIRECTION('center_axis',(-1.,-4.38245930773088E-16,0.));
#44875=DIRECTION('ref_axis',(4.38245930773088E-16,-1.,0.));
#44876=DIRECTION('center_axis',(-1.,-4.38245930773088E-16,0.));
#44877=DIRECTION('ref_axis',(-4.10746190391092E-16,0.937250437594515,-0.348656876067132));
#44878=DIRECTION('center_axis',(-1.,-4.38245930773088E-16,0.));
#44879=DIRECTION('ref_axis',(4.38245930773088E-16,-1.,0.));
#44880=DIRECTION('center_axis',(-1.,-4.38245930773088E-16,0.));
#44881=DIRECTION('ref_axis',(4.38245930773088E-16,-1.,0.));
#44882=DIRECTION('center_axis',(-1.,-4.38245930773088E-16,0.));
#44883=DIRECTION('ref_axis',(-4.10746190391092E-16,0.937250437594514,0.348656876067132));
#44884=DIRECTION('center_axis',(-1.,-4.38245930773088E-16,0.));
#44885=DIRECTION('ref_axis',(4.38245930773088E-16,-1.,0.));
#44886=DIRECTION('center_axis',(-1.,-4.38245930773088E-16,0.));
#44887=DIRECTION('ref_axis',(-3.3768778811311E-16,0.770544035668309,-0.637386765705091));
#44888=DIRECTION('center_axis',(-1.,-4.38245930773088E-16,0.));
#44889=DIRECTION('ref_axis',(4.38245930773088E-16,-1.,0.));
#44890=DIRECTION('center_axis',(-1.,-4.38245930773088E-16,0.));
#44891=DIRECTION('ref_axis',(4.38245930773088E-16,-1.,0.));
#44892=DIRECTION('center_axis',(-1.,-4.38245930773088E-16,0.));
#44893=DIRECTION('ref_axis',(4.38245930773088E-16,-1.,0.));
#44894=DIRECTION('center_axis',(-1.,-4.38245930773088E-16,0.));
#44895=DIRECTION('ref_axis',(-4.36006704245932E-16,0.994890479591663,0.100960059517961));
#44896=DIRECTION('center_axis',(-1.,-4.38245930773088E-16,0.));
#44897=DIRECTION('ref_axis',(4.38245930773088E-16,-1.,0.));
#44898=DIRECTION('center_axis',(-1.,-4.38245930773088E-16,0.));
#44899=DIRECTION('ref_axis',(4.38245930773088E-16,-1.,0.));
#44900=DIRECTION('center_axis',(-1.,-4.38245930773088E-16,0.));
#44901=DIRECTION('ref_axis',(-4.36006704245932E-16,0.994890479591662,-0.100960059517976));
#44902=DIRECTION('center_axis',(-1.,-4.38245930773088E-16,0.));
#44903=DIRECTION('ref_axis',(4.38245930773088E-16,-1.,0.));
#44904=DIRECTION('center_axis',(-1.,-4.38245930773088E-16,0.));
#44905=DIRECTION('ref_axis',(4.38245930773088E-16,-1.,0.));
#44906=DIRECTION('center_axis',(-1.,-4.38245930773088E-16,0.));
#44907=DIRECTION('ref_axis',(4.38245930773088E-16,-1.,0.));
#44908=DIRECTION('',(-1.,-4.38245930773088E-16,0.));
#44909=DIRECTION('',(-1.,-4.38245930773088E-16,0.));
#44910=DIRECTION('center_axis',(0.,0.,1.));
#44911=DIRECTION('ref_axis',(1.,0.,0.));
#44912=DIRECTION('',(-1.,-4.38245930773088E-16,0.));
#44913=DIRECTION('center_axis',(-1.,-4.38245930773088E-16,0.));
#44914=DIRECTION('ref_axis',(4.38245930773088E-16,-1.,0.));
#44915=DIRECTION('',(-1.,-4.38245930773088E-16,0.));
#44916=DIRECTION('center_axis',(3.09886669477059E-16,-0.707106781186543,
0.707106781186552));
#44917=DIRECTION('ref_axis',(-1.02926399073076E-32,-0.707106781186552,-0.707106781186543));
#44918=DIRECTION('',(-1.,-4.38245930773088E-16,0.));
#44919=DIRECTION('center_axis',(-1.,-4.38245930773088E-16,0.));
#44920=DIRECTION('ref_axis',(4.38245930773088E-16,-1.,0.));
#44921=DIRECTION('',(-1.,-4.38245930773088E-16,0.));
#44922=DIRECTION('center_axis',(4.38245930773088E-16,-1.,1.8333618114597E-15));
#44923=DIRECTION('ref_axis',(1.09941607071732E-47,-1.8333618114597E-15,
-1.));
#44924=DIRECTION('',(-1.,-4.38245930773088E-16,0.));
#44925=DIRECTION('center_axis',(-1.,-4.38245930773088E-16,0.));
#44926=DIRECTION('ref_axis',(4.38245930773088E-16,-1.,0.));
#44927=DIRECTION('',(-1.,-4.38245930773088E-16,0.));
#44928=DIRECTION('center_axis',(3.09886669477059E-16,-0.707106781186544,
-0.707106781186551));
#44929=DIRECTION('ref_axis',(8.09901984815823E-33,0.707106781186551,-0.707106781186544));
#44930=DIRECTION('',(-1.,-4.38245930773088E-16,0.));
#44931=DIRECTION('center_axis',(-1.,-4.38245930773088E-16,0.));
#44932=DIRECTION('ref_axis',(4.38245930773088E-16,-1.,0.));
#44933=DIRECTION('',(-1.,-4.38245930773088E-16,0.));
#44934=DIRECTION('center_axis',(-5.83988792200131E-31,1.3325595315168E-15,
-1.));
#44935=DIRECTION('ref_axis',(0.,1.,1.3325595315168E-15));
#44936=DIRECTION('',(-1.,-4.38245930773088E-16,0.));
#44937=DIRECTION('center_axis',(-1.,-4.38245930773088E-16,0.));
#44938=DIRECTION('ref_axis',(4.38245930773088E-16,-1.,0.));
#44939=DIRECTION('',(-1.,-4.38245930773088E-16,0.));
#44940=DIRECTION('center_axis',(-4.38245930773088E-16,1.,0.));
#44941=DIRECTION('ref_axis',(-1.,-4.38245930773088E-16,0.));
#44942=DIRECTION('center_axis',(4.38245930773088E-16,-1.,2.77555756156289E-15));
#44943=DIRECTION('ref_axis',(1.03714524497726E-47,-2.77555756156289E-15,
-1.));
#44944=DIRECTION('',(-1.,-4.38245930773088E-16,0.));
#44945=DIRECTION('',(-1.,-4.38245930773088E-16,0.));
#44946=DIRECTION('center_axis',(0.,0.,-1.));
#44947=DIRECTION('ref_axis',(-1.,0.,0.));
#44948=DIRECTION('',(-1.,-4.38245930773088E-16,0.));
#44949=DIRECTION('center_axis',(-4.38245930773088E-16,1.,-4.16333634234433E-15));
#44950=DIRECTION('ref_axis',(3.63000835742038E-47,4.16333634234433E-15,
1.));
#44951=DIRECTION('',(-1.,-4.38245930773088E-16,0.));
#44952=DIRECTION('center_axis',(0.,0.,1.));
#44953=DIRECTION('ref_axis',(1.,0.,0.));
#44954=DIRECTION('center_axis',(0.,-0.707106781186548,-0.707106781186548));
#44955=DIRECTION('ref_axis',(1.,0.,0.));
#44956=DIRECTION('center_axis',(0.,0.707106781186548,0.707106781186548));
#44957=DIRECTION('ref_axis',(-1.,0.,0.));
#44958=DIRECTION('center_axis',(0.,-0.707106781186548,0.707106781186548));
#44959=DIRECTION('ref_axis',(1.,0.,0.));
#44960=DIRECTION('center_axis',(0.,-0.707106781186548,0.707106781186548));
#44961=DIRECTION('ref_axis',(1.,0.,0.));
#44962=DIRECTION('center_axis',(0.,0.,-1.));
#44963=DIRECTION('ref_axis',(-1.,0.,0.));
#44964=DIRECTION('',(1.,1.46081976924362E-16,0.));
#44965=DIRECTION('center_axis',(1.,1.46081976924362E-16,0.));
#44966=DIRECTION('ref_axis',(1.46081976924362E-16,-1.,1.22464679914735E-16));
#44967=DIRECTION('',(1.,1.46081976924362E-16,0.));
#44968=DIRECTION('center_axis',(0.,0.,-1.));
#44969=DIRECTION('ref_axis',(-1.,0.,0.));
#44970=DIRECTION('center_axis',(0.,0.,1.));
#44971=DIRECTION('ref_axis',(1.,0.,0.));
#44972=DIRECTION('',(1.,1.46081976924362E-16,0.));
#44973=DIRECTION('center_axis',(0.,0.,1.));
#44974=DIRECTION('ref_axis',(1.,0.,0.));
#44975=DIRECTION('',(1.,1.46081976924362E-16,0.));
#44976=DIRECTION('center_axis',(1.,1.46081976924362E-16,0.));
#44977=DIRECTION('ref_axis',(1.46081976924362E-16,-1.,1.22464679914735E-16));
#44978=DIRECTION('center_axis',(0.,0.,1.));
#44979=DIRECTION('ref_axis',(1.,0.,0.));
#44980=DIRECTION('',(1.,1.46081976924362E-16,0.));
#44981=DIRECTION('center_axis',(0.,0.,1.));
#44982=DIRECTION('ref_axis',(1.,0.,0.));
#44983=DIRECTION('',(1.,1.46081976924362E-16,0.));
#44984=DIRECTION('center_axis',(1.,1.46081976924362E-16,0.));
#44985=DIRECTION('ref_axis',(1.46081976924362E-16,-1.,1.22464679914735E-16));
#44986=DIRECTION('center_axis',(0.,0.,-1.));
#44987=DIRECTION('ref_axis',(-1.,0.,0.));
#44988=DIRECTION('',(1.,1.46081976924362E-16,0.));
#44989=DIRECTION('center_axis',(1.,1.46081976924362E-16,0.));
#44990=DIRECTION('ref_axis',(1.46081976924362E-16,-1.,1.22464679914735E-16));
#44991=DIRECTION('',(1.,1.46081976924362E-16,0.));
#44992=DIRECTION('center_axis',(0.,0.,-1.));
#44993=DIRECTION('ref_axis',(-1.,0.,0.));
#44994=DIRECTION('center_axis',(0.,0.,1.));
#44995=DIRECTION('ref_axis',(1.,0.,0.));
#44996=DIRECTION('',(1.,1.46081976924362E-16,0.));
#44997=DIRECTION('center_axis',(0.,0.,1.));
#44998=DIRECTION('ref_axis',(1.,0.,0.));
#44999=DIRECTION('',(1.,1.46081976924362E-16,0.));
#45000=DIRECTION('center_axis',(1.,1.46081976924362E-16,0.));
#45001=DIRECTION('ref_axis',(1.46081976924362E-16,-1.,1.22464679914735E-16));
#45002=DIRECTION('center_axis',(0.,0.,-1.));
#45003=DIRECTION('ref_axis',(-1.,0.,0.));
#45004=DIRECTION('',(1.,1.46081976924362E-16,0.));
#45005=DIRECTION('center_axis',(1.,1.46081976924362E-16,0.));
#45006=DIRECTION('ref_axis',(1.46081976924362E-16,-1.,1.22464679914735E-16));
#45007=DIRECTION('',(1.,1.46081976924362E-16,0.));
#45008=DIRECTION('center_axis',(0.,0.,-1.));
#45009=DIRECTION('ref_axis',(-1.,0.,0.));
#45010=DIRECTION('center_axis',(0.,0.,-1.));
#45011=DIRECTION('ref_axis',(-1.,0.,0.));
#45012=DIRECTION('',(1.,1.46081976924362E-16,0.));
#45013=DIRECTION('center_axis',(1.,1.46081976924362E-16,0.));
#45014=DIRECTION('ref_axis',(1.46081976924362E-16,-1.,1.22464679914735E-16));
#45015=DIRECTION('',(1.,1.46081976924362E-16,0.));
#45016=DIRECTION('center_axis',(0.,0.,-1.));
#45017=DIRECTION('ref_axis',(-1.,0.,0.));
#45018=DIRECTION('center_axis',(0.,0.,1.));
#45019=DIRECTION('ref_axis',(1.,0.,0.));
#45020=DIRECTION('',(1.,1.46081976924362E-16,0.));
#45021=DIRECTION('center_axis',(0.,0.,1.));
#45022=DIRECTION('ref_axis',(1.,0.,0.));
#45023=DIRECTION('',(1.,1.46081976924362E-16,0.));
#45024=DIRECTION('center_axis',(1.,1.46081976924362E-16,0.));
#45025=DIRECTION('ref_axis',(1.46081976924362E-16,-1.,1.22464679914735E-16));
#45026=DIRECTION('center_axis',(0.,0.,1.));
#45027=DIRECTION('ref_axis',(1.,0.,0.));
#45028=DIRECTION('',(1.,1.46081976924362E-16,0.));
#45029=DIRECTION('center_axis',(0.,0.,1.));
#45030=DIRECTION('ref_axis',(1.,0.,0.));
#45031=DIRECTION('',(1.,1.46081976924362E-16,0.));
#45032=DIRECTION('center_axis',(1.,1.46081976924362E-16,0.));
#45033=DIRECTION('ref_axis',(1.46081976924362E-16,-1.,1.22464679914735E-16));
#45034=DIRECTION('center_axis',(0.,0.,1.));
#45035=DIRECTION('ref_axis',(1.,0.,0.));
#45036=DIRECTION('',(1.,1.46081976924362E-16,0.));
#45037=DIRECTION('center_axis',(0.,0.,1.));
#45038=DIRECTION('ref_axis',(1.,0.,0.));
#45039=DIRECTION('',(1.,1.46081976924362E-16,0.));
#45040=DIRECTION('center_axis',(1.,1.46081976924362E-16,0.));
#45041=DIRECTION('ref_axis',(1.46081976924362E-16,-1.,1.22464679914735E-16));
#45042=DIRECTION('center_axis',(0.,0.,1.));
#45043=DIRECTION('ref_axis',(1.,0.,0.));
#45044=DIRECTION('',(1.,1.46081976924362E-16,0.));
#45045=DIRECTION('center_axis',(0.,0.,1.));
#45046=DIRECTION('ref_axis',(1.,0.,0.));
#45047=DIRECTION('',(1.,1.46081976924362E-16,0.));
#45048=DIRECTION('center_axis',(1.,1.46081976924362E-16,0.));
#45049=DIRECTION('ref_axis',(1.46081976924362E-16,-1.,1.22464679914735E-16));
#45050=DIRECTION('center_axis',(0.,0.,-1.));
#45051=DIRECTION('ref_axis',(-1.,0.,0.));
#45052=DIRECTION('',(1.,1.46081976924362E-16,0.));
#45053=DIRECTION('center_axis',(1.,1.46081976924362E-16,0.));
#45054=DIRECTION('ref_axis',(1.46081976924362E-16,-1.,1.22464679914735E-16));
#45055=DIRECTION('',(1.,1.46081976924362E-16,0.));
#45056=DIRECTION('center_axis',(0.,0.,-1.));
#45057=DIRECTION('ref_axis',(-1.,0.,0.));
#45058=DIRECTION('center_axis',(0.,0.,-1.));
#45059=DIRECTION('ref_axis',(-1.,0.,0.));
#45060=DIRECTION('',(1.,1.46081976924362E-16,0.));
#45061=DIRECTION('center_axis',(1.,1.46081976924362E-16,0.));
#45062=DIRECTION('ref_axis',(1.46081976924362E-16,-1.,1.22464679914735E-16));
#45063=DIRECTION('',(1.,1.46081976924362E-16,0.));
#45064=DIRECTION('center_axis',(0.,0.,-1.));
#45065=DIRECTION('ref_axis',(-1.,0.,0.));
#45066=DIRECTION('center_axis',(0.,0.,-1.));
#45067=DIRECTION('ref_axis',(-1.,0.,0.));
#45068=DIRECTION('',(1.,1.46081976924362E-16,0.));
#45069=DIRECTION('center_axis',(1.,1.46081976924362E-16,0.));
#45070=DIRECTION('ref_axis',(1.46081976924362E-16,-1.,1.22464679914735E-16));
#45071=DIRECTION('',(1.,1.46081976924362E-16,0.));
#45072=DIRECTION('center_axis',(0.,0.,-1.));
#45073=DIRECTION('ref_axis',(-1.,0.,0.));
#45074=DIRECTION('center_axis',(0.,0.,-1.));
#45075=DIRECTION('ref_axis',(-1.,0.,0.));
#45076=DIRECTION('',(1.,1.46081976924362E-16,0.));
#45077=DIRECTION('center_axis',(1.,1.46081976924362E-16,0.));
#45078=DIRECTION('ref_axis',(1.46081976924362E-16,-1.,1.22464679914735E-16));
#45079=DIRECTION('',(1.,1.46081976924362E-16,0.));
#45080=DIRECTION('center_axis',(0.,0.,-1.));
#45081=DIRECTION('ref_axis',(-1.,0.,0.));
#45082=DIRECTION('center_axis',(0.,0.,-1.));
#45083=DIRECTION('ref_axis',(-1.,0.,0.));
#45084=DIRECTION('',(1.,1.46081976924362E-16,0.));
#45085=DIRECTION('center_axis',(1.,1.46081976924362E-16,0.));
#45086=DIRECTION('ref_axis',(1.46081976924362E-16,-1.,1.22464679914735E-16));
#45087=DIRECTION('',(1.,1.46081976924362E-16,0.));
#45088=DIRECTION('center_axis',(0.,0.,-1.));
#45089=DIRECTION('ref_axis',(-1.,0.,0.));
#45090=DIRECTION('center_axis',(0.,0.,-1.));
#45091=DIRECTION('ref_axis',(-1.,0.,0.));
#45092=DIRECTION('',(1.,1.46081976924362E-16,0.));
#45093=DIRECTION('center_axis',(1.,1.46081976924362E-16,0.));
#45094=DIRECTION('ref_axis',(1.46081976924362E-16,-1.,1.22464679914735E-16));
#45095=DIRECTION('',(1.,1.46081976924362E-16,0.));
#45096=DIRECTION('center_axis',(0.,0.,-1.));
#45097=DIRECTION('ref_axis',(-1.,0.,0.));
#45098=DIRECTION('center_axis',(0.,0.,-1.));
#45099=DIRECTION('ref_axis',(-1.,0.,0.));
#45100=DIRECTION('',(1.,1.46081976924362E-16,0.));
#45101=DIRECTION('center_axis',(1.,1.46081976924362E-16,0.));
#45102=DIRECTION('ref_axis',(1.46081976924362E-16,-1.,1.22464679914735E-16));
#45103=DIRECTION('',(1.,1.46081976924362E-16,0.));
#45104=DIRECTION('center_axis',(0.,0.,-1.));
#45105=DIRECTION('ref_axis',(-1.,0.,0.));
#45106=DIRECTION('center_axis',(0.,0.,1.));
#45107=DIRECTION('ref_axis',(1.,0.,0.));
#45108=DIRECTION('',(1.,1.46081976924362E-16,0.));
#45109=DIRECTION('center_axis',(0.,0.,1.));
#45110=DIRECTION('ref_axis',(1.,0.,0.));
#45111=DIRECTION('',(1.,1.46081976924362E-16,0.));
#45112=DIRECTION('center_axis',(1.,1.46081976924362E-16,0.));
#45113=DIRECTION('ref_axis',(1.46081976924362E-16,-1.,1.22464679914735E-16));
#45114=DIRECTION('center_axis',(0.,0.,1.));
#45115=DIRECTION('ref_axis',(1.,0.,0.));
#45116=DIRECTION('',(1.,1.46081976924362E-16,0.));
#45117=DIRECTION('center_axis',(0.,0.,1.));
#45118=DIRECTION('ref_axis',(1.,0.,0.));
#45119=DIRECTION('',(1.,1.46081976924362E-16,0.));
#45120=DIRECTION('center_axis',(1.,1.46081976924362E-16,0.));
#45121=DIRECTION('ref_axis',(1.46081976924362E-16,-1.,1.22464679914735E-16));
#45122=DIRECTION('center_axis',(0.,0.,1.));
#45123=DIRECTION('ref_axis',(1.,0.,0.));
#45124=DIRECTION('',(1.,1.46081976924362E-16,0.));
#45125=DIRECTION('center_axis',(0.,0.,1.));
#45126=DIRECTION('ref_axis',(1.,0.,0.));
#45127=DIRECTION('',(1.,1.46081976924362E-16,0.));
#45128=DIRECTION('center_axis',(1.,1.46081976924362E-16,0.));
#45129=DIRECTION('ref_axis',(1.46081976924362E-16,-1.,1.22464679914735E-16));
#45130=DIRECTION('center_axis',(0.,0.,1.));
#45131=DIRECTION('ref_axis',(1.,0.,0.));
#45132=DIRECTION('',(1.,1.46081976924362E-16,0.));
#45133=DIRECTION('center_axis',(0.,0.,1.));
#45134=DIRECTION('ref_axis',(1.,0.,0.));
#45135=DIRECTION('',(1.,1.46081976924362E-16,0.));
#45136=DIRECTION('center_axis',(1.,1.46081976924362E-16,0.));
#45137=DIRECTION('ref_axis',(1.46081976924362E-16,-1.,1.22464679914735E-16));
#45138=DIRECTION('center_axis',(0.,0.,1.));
#45139=DIRECTION('ref_axis',(1.,0.,0.));
#45140=DIRECTION('',(1.,1.46081976924362E-16,0.));
#45141=DIRECTION('center_axis',(0.,0.,1.));
#45142=DIRECTION('ref_axis',(1.,0.,0.));
#45143=DIRECTION('',(1.,1.46081976924362E-16,0.));
#45144=DIRECTION('center_axis',(1.,1.46081976924362E-16,0.));
#45145=DIRECTION('ref_axis',(1.46081976924362E-16,-1.,1.22464679914735E-16));
#45146=DIRECTION('center_axis',(0.,0.,-1.));
#45147=DIRECTION('ref_axis',(-1.,0.,0.));
#45148=DIRECTION('',(1.,1.46081976924362E-16,0.));
#45149=DIRECTION('center_axis',(1.,1.46081976924362E-16,0.));
#45150=DIRECTION('ref_axis',(1.46081976924362E-16,-1.,1.22464679914735E-16));
#45151=DIRECTION('',(1.,1.46081976924362E-16,0.));
#45152=DIRECTION('center_axis',(0.,0.,-1.));
#45153=DIRECTION('ref_axis',(-1.,0.,0.));
#45154=DIRECTION('center_axis',(0.,0.,-1.));
#45155=DIRECTION('ref_axis',(-1.,0.,0.));
#45156=DIRECTION('',(1.,1.46081976924362E-16,0.));
#45157=DIRECTION('center_axis',(1.,1.46081976924362E-16,0.));
#45158=DIRECTION('ref_axis',(1.46081976924362E-16,-1.,1.22464679914735E-16));
#45159=DIRECTION('',(1.,1.46081976924362E-16,0.));
#45160=DIRECTION('center_axis',(0.,0.,-1.));
#45161=DIRECTION('ref_axis',(-1.,0.,0.));
#45162=DIRECTION('center_axis',(0.,0.,1.));
#45163=DIRECTION('ref_axis',(1.,0.,0.));
#45164=DIRECTION('',(1.,1.46081976924362E-16,0.));
#45165=DIRECTION('center_axis',(1.,1.46081976924362E-16,0.));
#45166=DIRECTION('ref_axis',(1.46081976924362E-16,-1.,1.22464679914735E-16));
#45167=DIRECTION('',(1.,1.46081976924362E-16,0.));
#45168=DIRECTION('center_axis',(0.,0.,1.));
#45169=DIRECTION('ref_axis',(1.,0.,0.));
#45170=DIRECTION('center_axis',(0.,0.,1.));
#45171=DIRECTION('ref_axis',(1.,0.,0.));
#45172=DIRECTION('',(1.,1.46081976924362E-16,0.));
#45173=DIRECTION('center_axis',(1.,1.46081976924362E-16,0.));
#45174=DIRECTION('ref_axis',(1.46081976924362E-16,-1.,1.22464679914735E-16));
#45175=DIRECTION('',(1.,1.46081976924362E-16,0.));
#45176=DIRECTION('center_axis',(0.,0.,1.));
#45177=DIRECTION('ref_axis',(1.,0.,0.));
#45178=DIRECTION('center_axis',(0.,0.,-1.));
#45179=DIRECTION('ref_axis',(-1.,0.,0.));
#45180=DIRECTION('',(1.,1.46081976924362E-16,0.));
#45181=DIRECTION('center_axis',(1.,1.46081976924362E-16,0.));
#45182=DIRECTION('ref_axis',(1.46081976924362E-16,-1.,1.22464679914735E-16));
#45183=DIRECTION('',(1.,1.46081976924362E-16,0.));
#45184=DIRECTION('center_axis',(0.,0.,-1.));
#45185=DIRECTION('ref_axis',(-1.,0.,0.));
#45186=DIRECTION('center_axis',(0.,0.,1.));
#45187=DIRECTION('ref_axis',(1.,0.,0.));
#45188=DIRECTION('',(1.,1.46081976924362E-16,0.));
#45189=DIRECTION('center_axis',(1.,1.46081976924362E-16,0.));
#45190=DIRECTION('ref_axis',(1.46081976924362E-16,-1.,1.22464679914735E-16));
#45191=DIRECTION('',(1.,1.46081976924362E-16,0.));
#45192=DIRECTION('center_axis',(0.,0.,1.));
#45193=DIRECTION('ref_axis',(1.,0.,0.));
#45194=DIRECTION('center_axis',(0.,0.,-1.));
#45195=DIRECTION('ref_axis',(-1.,0.,0.));
#45196=DIRECTION('',(1.,1.46081976924362E-16,0.));
#45197=DIRECTION('center_axis',(1.,1.46081976924362E-16,0.));
#45198=DIRECTION('ref_axis',(1.46081976924362E-16,-1.,1.22464679914735E-16));
#45199=DIRECTION('',(1.,1.46081976924362E-16,0.));
#45200=DIRECTION('center_axis',(0.,0.,-1.));
#45201=DIRECTION('ref_axis',(-1.,0.,0.));
#45202=DIRECTION('center_axis',(0.,0.,-1.));
#45203=DIRECTION('ref_axis',(-1.,0.,0.));
#45204=DIRECTION('',(1.,1.46081976924362E-16,0.));
#45205=DIRECTION('center_axis',(1.,1.46081976924362E-16,0.));
#45206=DIRECTION('ref_axis',(1.46081976924362E-16,-1.,1.22464679914735E-16));
#45207=DIRECTION('',(1.,1.46081976924362E-16,0.));
#45208=DIRECTION('center_axis',(0.,0.,-1.));
#45209=DIRECTION('ref_axis',(-1.,0.,0.));
#45210=DIRECTION('center_axis',(0.,0.,1.));
#45211=DIRECTION('ref_axis',(1.,0.,0.));
#45212=DIRECTION('',(1.,1.46081976924362E-16,0.));
#45213=DIRECTION('center_axis',(1.,1.46081976924362E-16,0.));
#45214=DIRECTION('ref_axis',(1.46081976924362E-16,-1.,1.22464679914735E-16));
#45215=DIRECTION('',(1.,1.46081976924362E-16,0.));
#45216=DIRECTION('center_axis',(0.,0.,1.));
#45217=DIRECTION('ref_axis',(1.,0.,0.));
#45218=DIRECTION('center_axis',(0.,0.,1.));
#45219=DIRECTION('ref_axis',(1.,0.,0.));
#45220=DIRECTION('',(1.,1.46081976924362E-16,0.));
#45221=DIRECTION('center_axis',(1.,1.46081976924362E-16,0.));
#45222=DIRECTION('ref_axis',(1.46081976924362E-16,-1.,1.22464679914735E-16));
#45223=DIRECTION('',(1.,1.46081976924362E-16,0.));
#45224=DIRECTION('center_axis',(0.,0.,1.));
#45225=DIRECTION('ref_axis',(1.,0.,0.));
#45226=DIRECTION('center_axis',(0.,0.,1.));
#45227=DIRECTION('ref_axis',(1.,0.,0.));
#45228=DIRECTION('',(1.,1.46081976924362E-16,0.));
#45229=DIRECTION('center_axis',(1.,1.46081976924362E-16,0.));
#45230=DIRECTION('ref_axis',(1.46081976924362E-16,-1.,1.22464679914735E-16));
#45231=DIRECTION('',(1.,1.46081976924362E-16,0.));
#45232=DIRECTION('center_axis',(0.,0.,1.));
#45233=DIRECTION('ref_axis',(1.,0.,0.));
#45234=DIRECTION('center_axis',(0.,0.,1.));
#45235=DIRECTION('ref_axis',(1.,0.,0.));
#45236=DIRECTION('',(1.,1.46081976924362E-16,0.));
#45237=DIRECTION('center_axis',(1.,1.46081976924362E-16,0.));
#45238=DIRECTION('ref_axis',(1.46081976924362E-16,-1.,1.22464679914735E-16));
#45239=DIRECTION('',(1.,1.46081976924362E-16,0.));
#45240=DIRECTION('center_axis',(0.,0.,1.));
#45241=DIRECTION('ref_axis',(1.,0.,0.));
#45242=DIRECTION('center_axis',(0.,0.,-1.));
#45243=DIRECTION('ref_axis',(-1.,0.,0.));
#45244=DIRECTION('',(1.,1.46081976924362E-16,0.));
#45245=DIRECTION('center_axis',(1.,1.46081976924362E-16,0.));
#45246=DIRECTION('ref_axis',(1.46081976924362E-16,-1.,1.22464679914735E-16));
#45247=DIRECTION('',(1.,1.46081976924362E-16,0.));
#45248=DIRECTION('center_axis',(0.,0.,-1.));
#45249=DIRECTION('ref_axis',(-1.,0.,0.));
#45250=DIRECTION('center_axis',(0.,0.,-1.));
#45251=DIRECTION('ref_axis',(-1.,0.,0.));
#45252=DIRECTION('',(1.,1.46081976924362E-16,0.));
#45253=DIRECTION('center_axis',(1.,1.46081976924362E-16,0.));
#45254=DIRECTION('ref_axis',(1.46081976924362E-16,-1.,1.22464679914735E-16));
#45255=DIRECTION('',(1.,1.46081976924362E-16,0.));
#45256=DIRECTION('center_axis',(0.,0.,-1.));
#45257=DIRECTION('ref_axis',(-1.,0.,0.));
#45258=DIRECTION('center_axis',(0.,0.,-1.));
#45259=DIRECTION('ref_axis',(-1.,0.,0.));
#45260=DIRECTION('',(1.,1.46081976924362E-16,0.));
#45261=DIRECTION('center_axis',(1.,1.46081976924362E-16,0.));
#45262=DIRECTION('ref_axis',(1.46081976924362E-16,-1.,1.22464679914735E-16));
#45263=DIRECTION('',(1.,1.46081976924362E-16,0.));
#45264=DIRECTION('center_axis',(0.,0.,-1.));
#45265=DIRECTION('ref_axis',(-1.,0.,0.));
#45266=DIRECTION('center_axis',(0.,0.,-1.));
#45267=DIRECTION('ref_axis',(-1.,0.,0.));
#45268=DIRECTION('',(1.,1.46081976924362E-16,0.));
#45269=DIRECTION('center_axis',(1.,1.46081976924362E-16,0.));
#45270=DIRECTION('ref_axis',(1.46081976924362E-16,-1.,1.22464679914735E-16));
#45271=DIRECTION('',(1.,1.46081976924362E-16,0.));
#45272=DIRECTION('center_axis',(0.,0.,-1.));
#45273=DIRECTION('ref_axis',(-1.,0.,0.));
#45274=DIRECTION('center_axis',(0.,0.,-1.));
#45275=DIRECTION('ref_axis',(-1.,0.,0.));
#45276=DIRECTION('',(1.,1.46081976924362E-16,0.));
#45277=DIRECTION('center_axis',(1.,1.46081976924362E-16,0.));
#45278=DIRECTION('ref_axis',(1.46081976924362E-16,-1.,1.22464679914735E-16));
#45279=DIRECTION('',(1.,1.46081976924362E-16,0.));
#45280=DIRECTION('center_axis',(0.,0.,-1.));
#45281=DIRECTION('ref_axis',(-1.,0.,0.));
#45282=DIRECTION('center_axis',(0.,0.,-1.));
#45283=DIRECTION('ref_axis',(-1.,0.,0.));
#45284=DIRECTION('',(1.,1.46081976924362E-16,0.));
#45285=DIRECTION('center_axis',(1.,1.46081976924362E-16,0.));
#45286=DIRECTION('ref_axis',(1.46081976924362E-16,-1.,1.22464679914735E-16));
#45287=DIRECTION('',(1.,1.46081976924362E-16,0.));
#45288=DIRECTION('center_axis',(0.,0.,-1.));
#45289=DIRECTION('ref_axis',(-1.,0.,0.));
#45290=DIRECTION('center_axis',(0.,0.,-1.));
#45291=DIRECTION('ref_axis',(-1.,0.,0.));
#45292=DIRECTION('',(1.,1.46081976924362E-16,0.));
#45293=DIRECTION('center_axis',(1.,1.46081976924362E-16,0.));
#45294=DIRECTION('ref_axis',(1.46081976924362E-16,-1.,1.22464679914735E-16));
#45295=DIRECTION('',(1.,1.46081976924362E-16,0.));
#45296=DIRECTION('center_axis',(0.,0.,-1.));
#45297=DIRECTION('ref_axis',(-1.,0.,0.));
#45298=DIRECTION('center_axis',(0.,0.,1.));
#45299=DIRECTION('ref_axis',(1.,0.,0.));
#45300=DIRECTION('',(1.,1.46081976924362E-16,0.));
#45301=DIRECTION('center_axis',(1.,1.46081976924362E-16,0.));
#45302=DIRECTION('ref_axis',(1.46081976924362E-16,-1.,1.22464679914735E-16));
#45303=DIRECTION('',(1.,1.46081976924362E-16,0.));
#45304=DIRECTION('center_axis',(0.,0.,1.));
#45305=DIRECTION('ref_axis',(1.,0.,0.));
#45306=DIRECTION('center_axis',(0.,0.,1.));
#45307=DIRECTION('ref_axis',(1.,0.,0.));
#45308=DIRECTION('',(1.,1.46081976924362E-16,0.));
#45309=DIRECTION('center_axis',(1.,1.46081976924362E-16,0.));
#45310=DIRECTION('ref_axis',(1.46081976924362E-16,-1.,1.22464679914735E-16));
#45311=DIRECTION('',(1.,1.46081976924362E-16,0.));
#45312=DIRECTION('center_axis',(0.,0.,1.));
#45313=DIRECTION('ref_axis',(1.,0.,0.));
#45314=DIRECTION('center_axis',(0.,0.,1.));
#45315=DIRECTION('ref_axis',(1.,0.,0.));
#45316=DIRECTION('',(1.,1.46081976924362E-16,0.));
#45317=DIRECTION('center_axis',(1.,1.46081976924362E-16,0.));
#45318=DIRECTION('ref_axis',(1.46081976924362E-16,-1.,1.22464679914735E-16));
#45319=DIRECTION('',(1.,1.46081976924362E-16,0.));
#45320=DIRECTION('center_axis',(0.,0.,1.));
#45321=DIRECTION('ref_axis',(1.,0.,0.));
#45322=DIRECTION('center_axis',(0.,0.,1.));
#45323=DIRECTION('ref_axis',(1.,0.,0.));
#45324=DIRECTION('',(1.,1.46081976924362E-16,0.));
#45325=DIRECTION('center_axis',(1.,1.46081976924362E-16,0.));
#45326=DIRECTION('ref_axis',(1.46081976924362E-16,-1.,1.22464679914735E-16));
#45327=DIRECTION('',(1.,1.46081976924362E-16,0.));
#45328=DIRECTION('center_axis',(0.,0.,1.));
#45329=DIRECTION('ref_axis',(1.,0.,0.));
#45330=DIRECTION('center_axis',(0.,0.,1.));
#45331=DIRECTION('ref_axis',(1.,0.,0.));
#45332=DIRECTION('',(1.,1.46081976924362E-16,0.));
#45333=DIRECTION('center_axis',(1.,1.46081976924362E-16,0.));
#45334=DIRECTION('ref_axis',(1.46081976924362E-16,-1.,1.22464679914735E-16));
#45335=DIRECTION('',(1.,1.46081976924362E-16,0.));
#45336=DIRECTION('center_axis',(0.,0.,1.));
#45337=DIRECTION('ref_axis',(1.,0.,0.));
#45338=DIRECTION('center_axis',(0.,0.,-1.));
#45339=DIRECTION('ref_axis',(-1.,0.,0.));
#45340=DIRECTION('',(1.,1.46081976924362E-16,0.));
#45341=DIRECTION('center_axis',(1.,1.46081976924362E-16,0.));
#45342=DIRECTION('ref_axis',(1.46081976924362E-16,-1.,1.22464679914735E-16));
#45343=DIRECTION('',(1.,1.46081976924362E-16,0.));
#45344=DIRECTION('center_axis',(0.,0.,-1.));
#45345=DIRECTION('ref_axis',(-1.,0.,0.));
#45346=DIRECTION('center_axis',(-1.,-2.30915603506606E-31,-3.77113799125394E-15));
#45347=DIRECTION('ref_axis',(-3.77113799125394E-15,0.,1.));
#45348=DIRECTION('',(0.,-1.,6.12323399573677E-17));
#45349=DIRECTION('center_axis',(0.,6.12323399573677E-17,1.));
#45350=DIRECTION('ref_axis',(0.,-1.,6.12323399573677E-17));
#45351=DIRECTION('',(0.,-1.,6.12323399573677E-17));
#45352=DIRECTION('center_axis',(1.,0.,0.));
#45353=DIRECTION('ref_axis',(0.,0.,-1.));
#45354=DIRECTION('',(0.,-1.,0.));
#45355=DIRECTION('center_axis',(-1.,0.,0.));
#45356=DIRECTION('ref_axis',(0.,0.,1.));
#45357=DIRECTION('',(0.,-1.,0.));
#45358=DIRECTION('',(0.,-1.,6.12323399573677E-17));
#45359=DIRECTION('center_axis',(0.,6.12323399573677E-17,1.));
#45360=DIRECTION('ref_axis',(0.,-1.,6.12323399573677E-17));
#45361=DIRECTION('',(0.,-1.,6.12323399573677E-17));
#45362=DIRECTION('center_axis',(1.,0.,0.));
#45363=DIRECTION('ref_axis',(0.,0.,-1.));
#45364=DIRECTION('center_axis',(-1.,0.,0.));
#45365=DIRECTION('ref_axis',(0.,0.,1.));
#45366=DIRECTION('',(0.,0.,1.));
#45367=DIRECTION('center_axis',(-1.,0.,0.));
#45368=DIRECTION('ref_axis',(0.,0.,-1.));
#45369=DIRECTION('center_axis',(-1.,0.,0.));
#45370=DIRECTION('ref_axis',(0.,0.,-1.));
#45371=DIRECTION('center_axis',(-1.,0.,0.));
#45372=DIRECTION('ref_axis',(0.,0.,1.));
#45373=DIRECTION('center_axis',(1.,0.,0.));
#45374=DIRECTION('ref_axis',(0.,0.,-1.));
#45375=DIRECTION('',(0.,0.,1.));
#45376=DIRECTION('center_axis',(1.,0.,0.));
#45377=DIRECTION('ref_axis',(0.,0.,-1.));
#45378=DIRECTION('center_axis',(1.,0.,0.));
#45379=DIRECTION('ref_axis',(0.,0.,1.));
#45380=DIRECTION('center_axis',(1.,0.,0.));
#45381=DIRECTION('ref_axis',(0.,0.,1.));
#45382=DIRECTION('center_axis',(-1.,-1.15648231731787E-15,0.));
#45383=DIRECTION('ref_axis',(1.15648231731787E-15,-1.,0.));
#45384=DIRECTION('',(0.,0.,-1.));
#45385=DIRECTION('center_axis',(1.,0.,0.));
#45386=DIRECTION('ref_axis',(0.,0.,-1.));
#45387=DIRECTION('',(0.,0.,-1.));
#45388=DIRECTION('center_axis',(0.,0.,-1.));
#45389=DIRECTION('ref_axis',(-1.,0.,0.));
#45390=DIRECTION('',(0.,0.,-1.));
#45391=DIRECTION('center_axis',(3.56237856673809E-16,-1.,0.));
#45392=DIRECTION('ref_axis',(1.,3.56237856673809E-16,0.));
#45393=DIRECTION('',(0.,0.,-1.));
#45394=DIRECTION('center_axis',(0.,0.,-1.));
#45395=DIRECTION('ref_axis',(-1.,0.,0.));
#45396=DIRECTION('center_axis',(0.,-1.,0.));
#45397=DIRECTION('ref_axis',(-1.,0.,0.));
#45398=DIRECTION('center_axis',(0.,-1.,0.));
#45399=DIRECTION('ref_axis',(-1.,0.,0.));
#45400=DIRECTION('center_axis',(0.,-1.,0.));
#45401=DIRECTION('ref_axis',(-1.,0.,0.));
#45402=DIRECTION('center_axis',(0.,-1.,0.));
#45403=DIRECTION('ref_axis',(-1.,0.,0.));
#45404=DIRECTION('center_axis',(0.,1.,0.));
#45405=DIRECTION('ref_axis',(-1.,0.,0.));
#45406=DIRECTION('center_axis',(0.,1.,0.));
#45407=DIRECTION('ref_axis',(-1.,0.,0.));
#45408=DIRECTION('center_axis',(0.,-1.,0.));
#45409=DIRECTION('ref_axis',(-1.,0.,0.));
#45410=DIRECTION('center_axis',(0.,-1.,0.));
#45411=DIRECTION('ref_axis',(-1.,0.,0.));
#45412=DIRECTION('',(0.,-1.,0.));
#45413=DIRECTION('center_axis',(0.,1.,0.));
#45414=DIRECTION('ref_axis',(-1.,0.,0.));
#45415=DIRECTION('center_axis',(0.,-1.,0.));
#45416=DIRECTION('ref_axis',(-1.,0.,0.));
#45417=DIRECTION('center_axis',(0.,1.,0.));
#45418=DIRECTION('ref_axis',(-1.,0.,0.));
#45419=DIRECTION('',(0.,1.,0.));
#45420=DIRECTION('center_axis',(0.,-1.,0.));
#45421=DIRECTION('ref_axis',(-1.,0.,0.));
#45422=DIRECTION('center_axis',(0.,1.,0.));
#45423=DIRECTION('ref_axis',(0.,0.,1.));
#45424=DIRECTION('center_axis',(0.,1.,0.));
#45425=DIRECTION('ref_axis',(0.,0.,-1.));
#45426=DIRECTION('',(0.42443387623072,0.,-0.905458935958868));
#45427=DIRECTION('center_axis',(0.,-1.,0.));
#45428=DIRECTION('ref_axis',(0.,0.,-1.));
#45429=DIRECTION('',(1.,0.,0.));
#45430=DIRECTION('center_axis',(0.,-1.,0.));
#45431=DIRECTION('ref_axis',(0.,0.,-1.));
#45432=DIRECTION('',(0.42443387623072,0.,0.905458935958868));
#45433=DIRECTION('center_axis',(0.,1.,0.));
#45434=DIRECTION('ref_axis',(0.,0.,-1.));
#45435=DIRECTION('',(0.42443387623072,0.,0.905458935958868));
#45436=DIRECTION('center_axis',(0.,-1.,0.));
#45437=DIRECTION('ref_axis',(-1.,0.,0.));
#45438=DIRECTION('',(1.,0.,0.));
#45439=DIRECTION('center_axis',(0.,-1.,0.));
#45440=DIRECTION('ref_axis',(-1.,0.,0.));
#45441=DIRECTION('',(0.42443387623072,0.,-0.905458935958868));
#45442=DIRECTION('center_axis',(0.,1.,0.));
#45443=DIRECTION('ref_axis',(0.42443387623072,0.,0.905458935958868));
#45444=DIRECTION('center_axis',(0.,-1.,0.));
#45445=DIRECTION('ref_axis',(0.,0.,-1.));
#45446=DIRECTION('',(0.42443387623072,0.,0.905458935958868));
#45447=DIRECTION('center_axis',(0.,1.,0.));
#45448=DIRECTION('ref_axis',(0.,0.,-1.));
#45449=DIRECTION('',(1.,0.,0.));
#45450=DIRECTION('center_axis',(0.,1.,0.));
#45451=DIRECTION('ref_axis',(0.,0.,-1.));
#45452=DIRECTION('',(0.42443387623072,0.,-0.905458935958868));
#45453=DIRECTION('center_axis',(0.,-1.,0.));
#45454=DIRECTION('ref_axis',(0.,0.,-1.));
#45455=DIRECTION('',(0.42443387623072,0.,-0.905458935958868));
#45456=DIRECTION('center_axis',(0.,1.,0.));
#45457=DIRECTION('ref_axis',(-1.,0.,0.));
#45458=DIRECTION('',(1.,0.,0.));
#45459=DIRECTION('center_axis',(0.,1.,0.));
#45460=DIRECTION('ref_axis',(-1.,0.,0.));
#45461=DIRECTION('',(0.42443387623072,0.,0.905458935958868));
#45462=DIRECTION('center_axis',(0.,-1.,0.));
#45463=DIRECTION('ref_axis',(-1.,0.,0.));
#45464=DIRECTION('',(0.,-1.,0.));
#45465=DIRECTION('',(0.,1.,0.));
#45466=DIRECTION('center_axis',(0.,-1.,0.));
#45467=DIRECTION('ref_axis',(-1.,0.,0.));
#45468=DIRECTION('',(0.,-1.,0.));
#45469=DIRECTION('',(0.,1.,0.));
#45470=DIRECTION('center_axis',(0.905458935958868,0.,-0.42443387623072));
#45471=DIRECTION('ref_axis',(0.42443387623072,0.,0.905458935958868));
#45472=DIRECTION('center_axis',(-0.905458935958868,0.,-0.42443387623072));
#45473=DIRECTION('ref_axis',(0.42443387623072,0.,-0.905458935958868));
#45474=DIRECTION('center_axis',(0.,0.,-1.));
#45475=DIRECTION('ref_axis',(0.,-1.,0.));
#45476=DIRECTION('center_axis',(0.,-1.,0.));
#45477=DIRECTION('ref_axis',(-1.,0.,0.));
#45478=DIRECTION('',(0.,1.,0.));
#45479=DIRECTION('',(0.,-1.,0.));
#45480=DIRECTION('center_axis',(0.,-1.,0.));
#45481=DIRECTION('ref_axis',(-1.,0.,0.));
#45482=DIRECTION('',(0.,1.,0.));
#45483=DIRECTION('',(0.,-1.,0.));
#45484=DIRECTION('center_axis',(0.,-1.,0.));
#45485=DIRECTION('ref_axis',(-1.,0.,0.));
#45486=DIRECTION('',(0.,1.,0.));
#45487=DIRECTION('center_axis',(0.,-1.,0.));
#45488=DIRECTION('ref_axis',(-1.,0.,0.));
#45489=DIRECTION('',(0.,-1.,0.));
#45490=DIRECTION('center_axis',(0.905458935958868,0.,-0.42443387623072));
#45491=DIRECTION('ref_axis',(0.42443387623072,0.,0.905458935958868));
#45492=DIRECTION('center_axis',(-0.905458935958868,0.,-0.42443387623072));
#45493=DIRECTION('ref_axis',(0.42443387623072,0.,-0.905458935958868));
#45494=DIRECTION('center_axis',(0.,0.,-1.));
#45495=DIRECTION('ref_axis',(0.,-1.,0.));
#45496=DIRECTION('center_axis',(5.8432790769745E-16,-1.,0.));
#45497=DIRECTION('ref_axis',(1.,5.8432790769745E-16,0.));
#45498=DIRECTION('center_axis',(-5.8432790769745E-16,1.,0.));
#45499=DIRECTION('ref_axis',(1.,5.8432790769745E-16,0.));
#45500=DIRECTION('center_axis',(-5.8432790769745E-16,1.,0.));
#45501=DIRECTION('ref_axis',(1.,5.8432790769745E-16,0.));
#45502=DIRECTION('center_axis',(5.8432790769745E-16,-1.,0.));
#45503=DIRECTION('ref_axis',(1.,5.8432790769745E-16,0.));
#45504=DIRECTION('center_axis',(5.8432790769745E-16,-1.,0.));
#45505=DIRECTION('ref_axis',(1.,5.8432790769745E-16,0.));
#45506=DIRECTION('center_axis',(5.8432790769745E-16,-1.,0.));
#45507=DIRECTION('ref_axis',(1.,5.8432790769745E-16,0.));
#45508=DIRECTION('center_axis',(5.8432790769745E-16,-1.,0.));
#45509=DIRECTION('ref_axis',(1.,5.8432790769745E-16,0.));
#45510=DIRECTION('center_axis',(5.8432790769745E-16,-1.,0.));
#45511=DIRECTION('ref_axis',(1.,5.8432790769745E-16,-6.93889390390722E-15));
#45512=DIRECTION('',(5.8432790769745E-16,-1.,0.));
#45513=DIRECTION('center_axis',(-5.8432790769745E-16,1.,0.));
#45514=DIRECTION('ref_axis',(1.,5.8432790769745E-16,0.));
#45515=DIRECTION('center_axis',(5.8432790769745E-16,-1.,0.));
#45516=DIRECTION('ref_axis',(1.,5.8432790769745E-16,0.));
#45517=DIRECTION('center_axis',(-5.8432790769745E-16,1.,0.));
#45518=DIRECTION('ref_axis',(1.,5.8432790769745E-16,0.));
#45519=DIRECTION('',(-5.8432790769745E-16,1.,0.));
#45520=DIRECTION('center_axis',(5.8432790769745E-16,-1.,0.));
#45521=DIRECTION('ref_axis',(1.,5.8432790769745E-16,0.));
#45522=DIRECTION('center_axis',(5.8432790769745E-16,-1.,0.));
#45523=DIRECTION('ref_axis',(1.,5.8432790769745E-16,0.));
#45524=DIRECTION('center_axis',(5.8432790769745E-16,-1.,0.));
#45525=DIRECTION('ref_axis',(1.,5.8432790769745E-16,0.));
#45526=DIRECTION('',(-0.42443387623072,-2.48008558853815E-16,0.905458935958868));
#45527=DIRECTION('center_axis',(-5.8432790769745E-16,1.,0.));
#45528=DIRECTION('ref_axis',(1.,5.8432790769745E-16,0.));
#45529=DIRECTION('',(-1.,-5.8432790769745E-16,0.));
#45530=DIRECTION('center_axis',(-5.8432790769745E-16,1.,0.));
#45531=DIRECTION('ref_axis',(1.,5.8432790769745E-16,0.));
#45532=DIRECTION('',(-0.42443387623072,-2.48008558853815E-16,-0.905458935958868));
#45533=DIRECTION('center_axis',(5.8432790769745E-16,-1.,0.));
#45534=DIRECTION('ref_axis',(1.,5.8432790769745E-16,0.));
#45535=DIRECTION('',(-0.42443387623072,-2.48008558853815E-16,-0.905458935958868));
#45536=DIRECTION('center_axis',(-5.8432790769745E-16,1.,0.));
#45537=DIRECTION('ref_axis',(1.,5.8432790769745E-16,0.));
#45538=DIRECTION('',(-1.,-5.8432790769745E-16,0.));
#45539=DIRECTION('center_axis',(-5.8432790769745E-16,1.,0.));
#45540=DIRECTION('ref_axis',(1.,5.8432790769745E-16,0.));
#45541=DIRECTION('',(-0.42443387623072,-2.48008558853815E-16,0.905458935958868));
#45542=DIRECTION('center_axis',(5.8432790769745E-16,-1.,0.));
#45543=DIRECTION('ref_axis',(-1.,-5.8432790769745E-16,0.));
#45544=DIRECTION('center_axis',(-5.8432790769745E-16,1.,0.));
#45545=DIRECTION('ref_axis',(1.,5.8432790769745E-16,0.));
#45546=DIRECTION('',(-0.42443387623072,-2.48008558853815E-16,-0.905458935958868));
#45547=DIRECTION('center_axis',(5.8432790769745E-16,-1.,0.));
#45548=DIRECTION('ref_axis',(1.,5.8432790769745E-16,0.));
#45549=DIRECTION('',(-1.,-5.8432790769745E-16,0.));
#45550=DIRECTION('center_axis',(5.8432790769745E-16,-1.,0.));
#45551=DIRECTION('ref_axis',(1.,5.8432790769745E-16,0.));
#45552=DIRECTION('',(-0.42443387623072,-2.48008558853815E-16,0.905458935958868));
#45553=DIRECTION('center_axis',(-5.8432790769745E-16,1.,0.));
#45554=DIRECTION('ref_axis',(1.,5.8432790769745E-16,0.));
#45555=DIRECTION('',(-0.42443387623072,-2.48008558853815E-16,0.905458935958868));
#45556=DIRECTION('center_axis',(5.8432790769745E-16,-1.,0.));
#45557=DIRECTION('ref_axis',(1.,5.8432790769745E-16,0.));
#45558=DIRECTION('',(-1.,-5.8432790769745E-16,0.));
#45559=DIRECTION('center_axis',(5.8432790769745E-16,-1.,0.));
#45560=DIRECTION('ref_axis',(1.,5.8432790769745E-16,0.));
#45561=DIRECTION('',(-0.42443387623072,-2.48008558853815E-16,-0.905458935958868));
#45562=DIRECTION('center_axis',(5.8432790769745E-16,-1.,0.));
#45563=DIRECTION('ref_axis',(1.,5.8432790769745E-16,0.));
#45564=DIRECTION('',(-5.8432790769745E-16,1.,0.));
#45565=DIRECTION('',(5.8432790769745E-16,-1.,0.));
#45566=DIRECTION('center_axis',(5.8432790769745E-16,-1.,0.));
#45567=DIRECTION('ref_axis',(1.,5.8432790769745E-16,0.));
#45568=DIRECTION('',(-5.8432790769745E-16,1.,0.));
#45569=DIRECTION('',(5.8432790769745E-16,-1.,0.));
#45570=DIRECTION('center_axis',(-0.905458935958868,-5.29084925554805E-16,
-0.42443387623072));
#45571=DIRECTION('ref_axis',(-0.42443387623072,-2.48008558853815E-16,0.905458935958868));
#45572=DIRECTION('center_axis',(0.905458935958868,5.29084925554805E-16,
-0.42443387623072));
#45573=DIRECTION('ref_axis',(-0.42443387623072,-2.48008558853815E-16,-0.905458935958868));
#45574=DIRECTION('center_axis',(0.,0.,-1.));
#45575=DIRECTION('ref_axis',(5.8432790769745E-16,-1.,0.));
#45576=DIRECTION('center_axis',(5.8432790769745E-16,-1.,0.));
#45577=DIRECTION('ref_axis',(1.,5.8432790769745E-16,0.));
#45578=DIRECTION('',(5.8432790769745E-16,-1.,0.));
#45579=DIRECTION('',(-5.8432790769745E-16,1.,0.));
#45580=DIRECTION('center_axis',(5.8432790769745E-16,-1.,0.));
#45581=DIRECTION('ref_axis',(1.,5.8432790769745E-16,0.));
#45582=DIRECTION('',(5.8432790769745E-16,-1.,0.));
#45583=DIRECTION('',(-5.8432790769745E-16,1.,0.));
#45584=DIRECTION('center_axis',(5.8432790769745E-16,-1.,0.));
#45585=DIRECTION('ref_axis',(1.,5.8432790769745E-16,0.));
#45586=DIRECTION('',(-5.8432790769745E-16,1.,0.));
#45587=DIRECTION('center_axis',(5.8432790769745E-16,-1.,0.));
#45588=DIRECTION('ref_axis',(1.,5.8432790769745E-16,0.));
#45589=DIRECTION('',(5.8432790769745E-16,-1.,0.));
#45590=DIRECTION('center_axis',(-0.905458935958868,-5.29084925554805E-16,
-0.42443387623072));
#45591=DIRECTION('ref_axis',(-0.42443387623072,-2.48008558853815E-16,0.905458935958868));
#45592=DIRECTION('center_axis',(0.905458935958868,5.29084925554805E-16,
-0.42443387623072));
#45593=DIRECTION('ref_axis',(-0.42443387623072,-2.48008558853815E-16,-0.905458935958868));
#45594=DIRECTION('center_axis',(0.,0.,-1.));
#45595=DIRECTION('ref_axis',(5.8432790769745E-16,-1.,0.));
#45596=DIRECTION('center_axis',(1.,0.,0.));
#45597=DIRECTION('ref_axis',(0.,0.,-1.));
#45598=DIRECTION('',(0.,-1.,6.12323399573677E-17));
#45599=DIRECTION('center_axis',(0.,-6.12323399573677E-17,-1.));
#45600=DIRECTION('ref_axis',(0.,1.,-6.12323399573677E-17));
#45601=DIRECTION('',(0.,-1.,6.12323399573677E-17));
#45602=DIRECTION('center_axis',(-1.,0.,0.));
#45603=DIRECTION('ref_axis',(0.,0.,1.));
#45604=DIRECTION('',(0.,-1.,0.));
#45605=DIRECTION('center_axis',(1.,0.,0.));
#45606=DIRECTION('ref_axis',(0.,0.,-1.));
#45607=DIRECTION('',(0.,-1.,0.));
#45608=DIRECTION('',(0.,-1.,6.12323399573677E-17));
#45609=DIRECTION('center_axis',(0.,-6.12323399573677E-17,-1.));
#45610=DIRECTION('ref_axis',(0.,1.,-6.12323399573677E-17));
#45611=DIRECTION('',(0.,-1.,6.12323399573677E-17));
#45612=DIRECTION('center_axis',(-1.,2.30915603506606E-31,3.77113799125394E-15));
#45613=DIRECTION('ref_axis',(3.77113799125394E-15,0.,1.));
#45614=DIRECTION('center_axis',(1.,0.,0.));
#45615=DIRECTION('ref_axis',(0.,0.,-1.));
#45616=DIRECTION('',(-8.07567285923481E-30,6.98296267768627E-15,-1.));
#45617=DIRECTION('center_axis',(1.,0.,0.));
#45618=DIRECTION('ref_axis',(0.,0.,1.));
#45619=DIRECTION('center_axis',(1.,0.,0.));
#45620=DIRECTION('ref_axis',(0.,0.,1.));
#45621=DIRECTION('center_axis',(1.,0.,0.));
#45622=DIRECTION('ref_axis',(0.,0.,-1.));
#45623=DIRECTION('center_axis',(-1.,0.,0.));
#45624=DIRECTION('ref_axis',(0.,0.,1.));
#45625=DIRECTION('',(0.,6.98296267768627E-15,-1.));
#45626=DIRECTION('center_axis',(-1.,0.,0.));
#45627=DIRECTION('ref_axis',(0.,0.,1.));
#45628=DIRECTION('center_axis',(-1.,0.,0.));
#45629=DIRECTION('ref_axis',(0.,0.,-1.));
#45630=DIRECTION('',(1.,-8.07567285923482E-31,0.));
#45631=DIRECTION('center_axis',(-1.,0.,0.));
#45632=DIRECTION('ref_axis',(0.,0.,-1.));
#45633=DIRECTION('',(-1.,8.07567285923482E-31,0.));
#45634=DIRECTION('center_axis',(1.,1.15648231731787E-15,0.));
#45635=DIRECTION('ref_axis',(-1.15648231731787E-15,1.,0.));
#45636=DIRECTION('',(-1.15648231731787E-15,1.,0.));
#45637=DIRECTION('',(-1.15648231731787E-15,1.,0.));
#45638=DIRECTION('',(0.,0.,1.));
#45639=DIRECTION('center_axis',(-1.,0.,0.));
#45640=DIRECTION('ref_axis',(0.,0.,1.));
#45641=DIRECTION('',(0.,-1.,0.));
#45642=DIRECTION('',(0.,-1.,0.));
#45643=DIRECTION('',(0.,0.,1.));
#45644=DIRECTION('center_axis',(0.,0.,1.));
#45645=DIRECTION('ref_axis',(-1.,0.,0.));
#45646=DIRECTION('center_axis',(0.,0.,1.));
#45647=DIRECTION('ref_axis',(1.,0.,0.));
#45648=DIRECTION('',(-1.,-3.56237856673809E-16,0.));
#45649=DIRECTION('center_axis',(0.,0.,1.));
#45650=DIRECTION('ref_axis',(1.,0.,0.));
#45651=DIRECTION('center_axis',(0.,0.,1.));
#45652=DIRECTION('ref_axis',(-1.,0.,0.));
#45653=DIRECTION('center_axis',(0.,0.,1.));
#45654=DIRECTION('ref_axis',(1.,0.,0.));
#45655=DIRECTION('',(-1.,-3.56237856673809E-16,0.));
#45656=DIRECTION('center_axis',(0.,0.,1.));
#45657=DIRECTION('ref_axis',(1.,0.,0.));
#45658=DIRECTION('center_axis',(0.,0.,1.));
#45659=DIRECTION('ref_axis',(1.,0.,0.));
#45660=DIRECTION('',(0.,0.,1.));
#45661=DIRECTION('center_axis',(-3.56237856673809E-16,1.,0.));
#45662=DIRECTION('ref_axis',(-1.,-3.56237856673809E-16,0.));
#45663=DIRECTION('',(0.,0.,1.));
#45664=DIRECTION('center_axis',(0.,0.,1.));
#45665=DIRECTION('ref_axis',(1.,0.,0.));
#52452=CARTESIAN_POINT('',(0.,0.,0.));
#52453=CARTESIAN_POINT('Origin',(-74.39,83.,-72.));
#52454=CARTESIAN_POINT('',(-83.59,84.75,-72.));
#52455=CARTESIAN_POINT('Origin',(-83.59,83.,-72.));
#52456=CARTESIAN_POINT('',(-84.39,84.75,-72.));
#52457=CARTESIAN_POINT('',(-74.39,84.75,-72.));
#52458=CARTESIAN_POINT('Origin',(-84.39,83.,-72.));
#52459=CARTESIAN_POINT('Origin',(-74.39,1.15752220392301,-72.));
#52460=CARTESIAN_POINT('',(-83.59,2.907522203923,-72.));
#52461=CARTESIAN_POINT('Origin',(-83.59,1.157522203923,-72.));
#52462=CARTESIAN_POINT('',(-84.39,2.907522203923,-72.));
#52463=CARTESIAN_POINT('',(-74.39,2.907522203923,-72.));
#52464=CARTESIAN_POINT('Origin',(-84.39,1.157522203923,-72.));
#52465=CARTESIAN_POINT('Origin',(-74.39,1.15752220392301,72.));
#52466=CARTESIAN_POINT('',(-83.59,2.907522203923,72.));
#52467=CARTESIAN_POINT('Origin',(-83.59,1.157522203923,72.));
#52468=CARTESIAN_POINT('',(-84.39,2.907522203923,72.));
#52469=CARTESIAN_POINT('',(-74.39,2.907522203923,72.));
#52470=CARTESIAN_POINT('Origin',(-84.39,1.157522203923,72.));
#52471=CARTESIAN_POINT('Origin',(-74.39,83.,72.));
#52472=CARTESIAN_POINT('',(-83.59,84.75,72.));
#52473=CARTESIAN_POINT('Origin',(-83.59,83.,72.));
#52474=CARTESIAN_POINT('',(-84.39,84.75,72.));
#52475=CARTESIAN_POINT('',(-74.39,84.75,72.));
#52476=CARTESIAN_POINT('Origin',(-84.39,83.,72.));
#52477=CARTESIAN_POINT('Origin',(38.3304246383764,1.80000000000005,76.7999999999841));
#52478=CARTESIAN_POINT('',(39.5804246383764,1.80000000000005,76.7999999999841));
#52479=CARTESIAN_POINT('Origin',(38.3304246383764,1.80000000000005,76.7999999999841));
#52480=CARTESIAN_POINT('',(39.5804246383764,1.80000000000005,75.9999999999841));
#52481=CARTESIAN_POINT('',(39.5804246383764,1.80000000000005,76.7999999999841));
#52482=CARTESIAN_POINT('Origin',(38.3304246383764,1.80000000000005,75.9999999999841));
#52483=CARTESIAN_POINT('Origin',(-52.1104246383764,1.80000000000003,76.7999999999841));
#52484=CARTESIAN_POINT('',(-50.8604246383764,1.80000000000003,76.7999999999841));
#52485=CARTESIAN_POINT('Origin',(-52.1104246383764,1.80000000000003,76.7999999999841));
#52486=CARTESIAN_POINT('',(-50.8604246383764,1.80000000000003,75.9999999999841));
#52487=CARTESIAN_POINT('',(-50.8604246383764,1.80000000000003,76.7999999999841));
#52488=CARTESIAN_POINT('Origin',(-52.1104246383764,1.80000000000003,75.9999999999841));
#52489=CARTESIAN_POINT('Origin',(60.61,66.0787611019615,38.));
#52490=CARTESIAN_POINT('',(69.81,66.0787611019615,36.5));
#52491=CARTESIAN_POINT('',(69.81,66.0787611019615,39.5));
#52492=CARTESIAN_POINT('Origin',(69.81,66.0787611019615,38.));
#52493=CARTESIAN_POINT('',(70.61,66.0787611019615,36.5));
#52494=CARTESIAN_POINT('',(60.61,66.0787611019615,36.5));
#52495=CARTESIAN_POINT('',(70.61,66.0787611019615,39.5));
#52496=CARTESIAN_POINT('Origin',(70.61,66.0787611019615,38.));
#52497=CARTESIAN_POINT('',(60.61,66.0787611019615,39.5));
#52498=CARTESIAN_POINT('Origin',(60.61,38.0787611019615,68.));
#52499=CARTESIAN_POINT('',(69.81,38.0787611019615,69.5));
#52500=CARTESIAN_POINT('',(69.81,38.0787611019615,66.5));
#52501=CARTESIAN_POINT('Origin',(69.81,38.0787611019615,68.));
#52502=CARTESIAN_POINT('',(70.61,38.0787611019615,66.5));
#52503=CARTESIAN_POINT('',(60.61,38.0787611019615,66.5));
#52504=CARTESIAN_POINT('',(70.61,38.0787611019615,69.5));
#52505=CARTESIAN_POINT('Origin',(70.61,38.0787611019615,68.));
#52506=CARTESIAN_POINT('',(60.61,38.0787611019615,69.5));
#52507=CARTESIAN_POINT('Origin',(60.61,38.0787611019615,63.));
#52508=CARTESIAN_POINT('',(69.81,38.0787611019615,64.5));
#52509=CARTESIAN_POINT('',(69.81,38.0787611019615,61.5));
#52510=CARTESIAN_POINT('Origin',(69.81,38.0787611019615,63.));
#52511=CARTESIAN_POINT('',(70.61,38.0787611019615,61.5));
#52512=CARTESIAN_POINT('',(60.61,38.0787611019615,61.5));
#52513=CARTESIAN_POINT('',(70.61,38.0787611019615,64.5));
#52514=CARTESIAN_POINT('Origin',(70.61,38.0787611019615,63.));
#52515=CARTESIAN_POINT('',(60.61,38.0787611019615,64.5));
#52516=CARTESIAN_POINT('Origin',(60.61,38.0787611019615,58.));
#52517=CARTESIAN_POINT('',(69.81,38.0787611019615,59.5));
#52518=CARTESIAN_POINT('',(69.81,38.0787611019615,56.5));
#52519=CARTESIAN_POINT('Origin',(69.81,38.0787611019615,58.));
#52520=CARTESIAN_POINT('',(70.61,38.0787611019615,56.5));
#52521=CARTESIAN_POINT('',(60.61,38.0787611019615,56.5));
#52522=CARTESIAN_POINT('',(70.61,38.0787611019615,59.5));
#52523=CARTESIAN_POINT('Origin',(70.61,38.0787611019615,58.));
#52524=CARTESIAN_POINT('',(60.61,38.0787611019615,59.5));
#52525=CARTESIAN_POINT('Origin',(60.61,38.0787611019615,38.));
#52526=CARTESIAN_POINT('',(69.81,38.0787611019615,39.5));
#52527=CARTESIAN_POINT('',(69.81,38.0787611019615,36.5));
#52528=CARTESIAN_POINT('Origin',(69.81,38.0787611019615,38.));
#52529=CARTESIAN_POINT('',(70.61,38.0787611019615,36.5));
#52530=CARTESIAN_POINT('',(60.61,38.0787611019615,36.5));
#52531=CARTESIAN_POINT('',(70.61,38.0787611019615,39.5));
#52532=CARTESIAN_POINT('Origin',(70.61,38.0787611019615,38.));
#52533=CARTESIAN_POINT('',(60.61,38.0787611019615,39.5));
#52534=CARTESIAN_POINT('Origin',(60.61,38.0787611019615,33.));
#52535=CARTESIAN_POINT('',(69.81,38.0787611019615,34.5));
#52536=CARTESIAN_POINT('',(69.81,38.0787611019615,31.5));
#52537=CARTESIAN_POINT('Origin',(69.81,38.0787611019615,33.));
#52538=CARTESIAN_POINT('',(70.61,38.0787611019615,31.5));
#52539=CARTESIAN_POINT('',(60.61,38.0787611019615,31.5));
#52540=CARTESIAN_POINT('',(70.61,38.0787611019615,34.5));
#52541=CARTESIAN_POINT('Origin',(70.61,38.0787611019615,33.));
#52542=CARTESIAN_POINT('',(60.61,38.0787611019615,34.5));
#52543=CARTESIAN_POINT('Origin',(60.61,66.0787611019615,33.));
#52544=CARTESIAN_POINT('',(69.81,66.0787611019615,31.5));
#52545=CARTESIAN_POINT('',(69.81,66.0787611019615,34.5));
#52546=CARTESIAN_POINT('Origin',(69.81,66.0787611019615,33.));
#52547=CARTESIAN_POINT('',(70.61,66.0787611019615,31.5));
#52548=CARTESIAN_POINT('',(60.61,66.0787611019615,31.5));
#52549=CARTESIAN_POINT('',(70.61,66.0787611019615,34.5));
#52550=CARTESIAN_POINT('Origin',(70.61,66.0787611019615,33.));
#52551=CARTESIAN_POINT('',(60.61,66.0787611019615,34.5));
#52552=CARTESIAN_POINT('Origin',(60.61,66.0787611019615,28.));
#52553=CARTESIAN_POINT('',(69.81,66.0787611019615,26.5));
#52554=CARTESIAN_POINT('',(69.81,66.0787611019615,29.5));
#52555=CARTESIAN_POINT('Origin',(69.81,66.0787611019615,28.));
#52556=CARTESIAN_POINT('',(70.61,66.0787611019615,26.5));
#52557=CARTESIAN_POINT('',(60.61,66.0787611019615,26.5));
#52558=CARTESIAN_POINT('',(70.61,66.0787611019615,29.5));
#52559=CARTESIAN_POINT('Origin',(70.61,66.0787611019615,28.));
#52560=CARTESIAN_POINT('',(60.61,66.0787611019615,29.5));
#52561=CARTESIAN_POINT('Origin',(60.61,66.0787611019615,63.));
#52562=CARTESIAN_POINT('',(69.81,66.0787611019615,61.5));
#52563=CARTESIAN_POINT('',(69.81,66.0787611019615,64.5));
#52564=CARTESIAN_POINT('Origin',(69.81,66.0787611019615,63.));
#52565=CARTESIAN_POINT('',(70.61,66.0787611019615,61.5));
#52566=CARTESIAN_POINT('',(60.61,66.0787611019615,61.5));
#52567=CARTESIAN_POINT('',(70.61,66.0787611019615,64.5));
#52568=CARTESIAN_POINT('Origin',(70.61,66.0787611019615,63.));
#52569=CARTESIAN_POINT('',(60.61,66.0787611019615,64.5));
#52570=CARTESIAN_POINT('Origin',(60.61,66.0787611019615,58.));
#52571=CARTESIAN_POINT('',(69.81,66.0787611019615,56.5));
#52572=CARTESIAN_POINT('',(69.81,66.0787611019615,59.5));
#52573=CARTESIAN_POINT('Origin',(69.81,66.0787611019615,58.));
#52574=CARTESIAN_POINT('',(70.61,66.0787611019615,56.5));
#52575=CARTESIAN_POINT('',(60.61,66.0787611019615,56.5));
#52576=CARTESIAN_POINT('',(70.61,66.0787611019615,59.5));
#52577=CARTESIAN_POINT('Origin',(70.61,66.0787611019615,58.));
#52578=CARTESIAN_POINT('',(60.61,66.0787611019615,59.5));
#52579=CARTESIAN_POINT('Origin',(60.61,66.0787611019615,53.));
#52580=CARTESIAN_POINT('',(69.81,66.0787611019615,51.5));
#52581=CARTESIAN_POINT('',(69.81,66.0787611019615,54.5));
#52582=CARTESIAN_POINT('Origin',(69.81,66.0787611019615,53.));
#52583=CARTESIAN_POINT('',(70.61,66.0787611019615,51.5));
#52584=CARTESIAN_POINT('',(60.61,66.0787611019615,51.5));
#52585=CARTESIAN_POINT('',(70.61,66.0787611019615,54.5));
#52586=CARTESIAN_POINT('Origin',(70.61,66.0787611019615,53.));
#52587=CARTESIAN_POINT('',(60.61,66.0787611019615,54.5));
#52588=CARTESIAN_POINT('Origin',(60.61,66.0787611019615,48.));
#52589=CARTESIAN_POINT('',(69.81,66.0787611019615,46.5));
#52590=CARTESIAN_POINT('',(69.81,66.0787611019615,49.5));
#52591=CARTESIAN_POINT('Origin',(69.81,66.0787611019615,48.));
#52592=CARTESIAN_POINT('',(70.61,66.0787611019615,46.5));
#52593=CARTESIAN_POINT('',(60.61,66.0787611019615,46.5));
#52594=CARTESIAN_POINT('',(70.61,66.0787611019615,49.5));
#52595=CARTESIAN_POINT('Origin',(70.61,66.0787611019615,48.));
#52596=CARTESIAN_POINT('',(60.61,66.0787611019615,49.5));
#52597=CARTESIAN_POINT('Origin',(60.61,66.0787611019615,43.));
#52598=CARTESIAN_POINT('',(69.81,66.0787611019615,41.5));
#52599=CARTESIAN_POINT('',(69.81,66.0787611019615,44.5));
#52600=CARTESIAN_POINT('Origin',(69.81,66.0787611019615,43.));
#52601=CARTESIAN_POINT('',(70.61,66.0787611019615,41.5));
#52602=CARTESIAN_POINT('',(60.61,66.0787611019615,41.5));
#52603=CARTESIAN_POINT('',(70.61,66.0787611019615,44.5));
#52604=CARTESIAN_POINT('Origin',(70.61,66.0787611019615,43.));
#52605=CARTESIAN_POINT('',(60.61,66.0787611019615,44.5));
#52606=CARTESIAN_POINT('Origin',(60.61,38.0787611019615,43.));
#52607=CARTESIAN_POINT('',(69.81,38.0787611019615,44.5));
#52608=CARTESIAN_POINT('',(69.81,38.0787611019615,41.5));
#52609=CARTESIAN_POINT('Origin',(69.81,38.0787611019615,43.));
#52610=CARTESIAN_POINT('',(70.61,38.0787611019615,41.5));
#52611=CARTESIAN_POINT('',(60.61,38.0787611019615,41.5));
#52612=CARTESIAN_POINT('',(70.61,38.0787611019615,44.5));
#52613=CARTESIAN_POINT('Origin',(70.61,38.0787611019615,43.));
#52614=CARTESIAN_POINT('',(60.61,38.0787611019615,44.5));
#52615=CARTESIAN_POINT('Origin',(60.61,38.0787611019615,48.));
#52616=CARTESIAN_POINT('',(69.81,38.0787611019615,49.5));
#52617=CARTESIAN_POINT('',(69.81,38.0787611019615,46.5));
#52618=CARTESIAN_POINT('Origin',(69.81,38.0787611019615,48.));
#52619=CARTESIAN_POINT('',(70.61,38.0787611019615,46.5));
#52620=CARTESIAN_POINT('',(60.61,38.0787611019615,46.5));
#52621=CARTESIAN_POINT('',(70.61,38.0787611019615,49.5));
#52622=CARTESIAN_POINT('Origin',(70.61,38.0787611019615,48.));
#52623=CARTESIAN_POINT('',(60.61,38.0787611019615,49.5));
#52624=CARTESIAN_POINT('Origin',(60.61,38.0787611019615,53.));
#52625=CARTESIAN_POINT('',(69.81,38.0787611019615,54.5));
#52626=CARTESIAN_POINT('',(69.81,38.0787611019615,51.5));
#52627=CARTESIAN_POINT('Origin',(69.81,38.0787611019615,53.));
#52628=CARTESIAN_POINT('',(70.61,38.0787611019615,51.5));
#52629=CARTESIAN_POINT('',(60.61,38.0787611019615,51.5));
#52630=CARTESIAN_POINT('',(70.61,38.0787611019615,54.5));
#52631=CARTESIAN_POINT('Origin',(70.61,38.0787611019615,53.));
#52632=CARTESIAN_POINT('',(60.61,38.0787611019615,54.5));
#52633=CARTESIAN_POINT('Origin',(60.61,38.0787611019615,13.));
#52634=CARTESIAN_POINT('',(69.81,38.0787611019615,14.5));
#52635=CARTESIAN_POINT('',(69.81,38.0787611019615,11.5));
#52636=CARTESIAN_POINT('Origin',(69.81,38.0787611019615,13.));
#52637=CARTESIAN_POINT('',(70.61,38.0787611019615,11.5));
#52638=CARTESIAN_POINT('',(60.61,38.0787611019615,11.5));
#52639=CARTESIAN_POINT('',(70.61,38.0787611019615,14.5));
#52640=CARTESIAN_POINT('Origin',(70.61,38.0787611019615,13.));
#52641=CARTESIAN_POINT('',(60.61,38.0787611019615,14.5));
#52642=CARTESIAN_POINT('Origin',(60.61,66.0787611019615,13.));
#52643=CARTESIAN_POINT('',(69.81,66.0787611019615,11.5));
#52644=CARTESIAN_POINT('',(69.81,66.0787611019615,14.5));
#52645=CARTESIAN_POINT('Origin',(69.81,66.0787611019615,13.));
#52646=CARTESIAN_POINT('',(70.61,66.0787611019615,11.5));
#52647=CARTESIAN_POINT('',(60.61,66.0787611019615,11.5));
#52648=CARTESIAN_POINT('',(70.61,66.0787611019615,14.5));
#52649=CARTESIAN_POINT('Origin',(70.61,66.0787611019615,13.));
#52650=CARTESIAN_POINT('',(60.61,66.0787611019615,14.5));
#52651=CARTESIAN_POINT('Origin',(60.61,66.0787611019615,18.));
#52652=CARTESIAN_POINT('',(69.81,66.0787611019615,16.5));
#52653=CARTESIAN_POINT('',(69.81,66.0787611019615,19.5));
#52654=CARTESIAN_POINT('Origin',(69.81,66.0787611019615,18.));
#52655=CARTESIAN_POINT('',(70.61,66.0787611019615,16.5));
#52656=CARTESIAN_POINT('',(60.61,66.0787611019615,16.5));
#52657=CARTESIAN_POINT('',(70.61,66.0787611019615,19.5));
#52658=CARTESIAN_POINT('Origin',(70.61,66.0787611019615,18.));
#52659=CARTESIAN_POINT('',(60.61,66.0787611019615,19.5));
#52660=CARTESIAN_POINT('Origin',(60.61,38.0787611019615,28.));
#52661=CARTESIAN_POINT('',(69.81,38.0787611019615,29.5));
#52662=CARTESIAN_POINT('',(69.81,38.0787611019615,26.5));
#52663=CARTESIAN_POINT('Origin',(69.81,38.0787611019615,28.));
#52664=CARTESIAN_POINT('',(70.61,38.0787611019615,26.5));
#52665=CARTESIAN_POINT('',(60.61,38.0787611019615,26.5));
#52666=CARTESIAN_POINT('',(70.61,38.0787611019615,29.5));
#52667=CARTESIAN_POINT('Origin',(70.61,38.0787611019615,28.));
#52668=CARTESIAN_POINT('',(60.61,38.0787611019615,29.5));
#52669=CARTESIAN_POINT('Origin',(60.61,66.0787611019615,23.));
#52670=CARTESIAN_POINT('',(69.81,66.0787611019615,21.5));
#52671=CARTESIAN_POINT('',(69.81,66.0787611019615,24.5));
#52672=CARTESIAN_POINT('Origin',(69.81,66.0787611019615,23.));
#52673=CARTESIAN_POINT('',(70.61,66.0787611019615,21.5));
#52674=CARTESIAN_POINT('',(60.61,66.0787611019615,21.5));
#52675=CARTESIAN_POINT('',(70.61,66.0787611019615,24.5));
#52676=CARTESIAN_POINT('Origin',(70.61,66.0787611019615,23.));
#52677=CARTESIAN_POINT('',(60.61,66.0787611019615,24.5));
#52678=CARTESIAN_POINT('Origin',(60.61,38.0787611019615,23.));
#52679=CARTESIAN_POINT('',(69.81,38.0787611019615,24.5));
#52680=CARTESIAN_POINT('',(69.81,38.0787611019615,21.5));
#52681=CARTESIAN_POINT('Origin',(69.81,38.0787611019615,23.));
#52682=CARTESIAN_POINT('',(70.61,38.0787611019615,21.5));
#52683=CARTESIAN_POINT('',(60.61,38.0787611019615,21.5));
#52684=CARTESIAN_POINT('',(70.61,38.0787611019615,24.5));
#52685=CARTESIAN_POINT('Origin',(70.61,38.0787611019615,23.));
#52686=CARTESIAN_POINT('',(60.61,38.0787611019615,24.5));
#52687=CARTESIAN_POINT('Origin',(60.61,38.0787611019615,18.));
#52688=CARTESIAN_POINT('',(69.81,38.0787611019615,19.5));
#52689=CARTESIAN_POINT('',(69.81,38.0787611019615,16.5));
#52690=CARTESIAN_POINT('Origin',(69.81,38.0787611019615,18.));
#52691=CARTESIAN_POINT('',(70.61,38.0787611019615,16.5));
#52692=CARTESIAN_POINT('',(60.61,38.0787611019615,16.5));
#52693=CARTESIAN_POINT('',(70.61,38.0787611019615,19.5));
#52694=CARTESIAN_POINT('Origin',(70.61,38.0787611019615,18.));
#52695=CARTESIAN_POINT('',(60.61,38.0787611019615,19.5));
#52696=CARTESIAN_POINT('Origin',(60.61,66.0787611019615,68.));
#52697=CARTESIAN_POINT('',(69.81,66.0787611019615,66.5));
#52698=CARTESIAN_POINT('',(69.81,66.0787611019615,69.5));
#52699=CARTESIAN_POINT('Origin',(69.81,66.0787611019615,68.));
#52700=CARTESIAN_POINT('',(70.61,66.0787611019615,66.5));
#52701=CARTESIAN_POINT('',(60.61,66.0787611019615,66.5));
#52702=CARTESIAN_POINT('',(70.61,66.0787611019615,69.5));
#52703=CARTESIAN_POINT('Origin',(70.61,66.0787611019615,68.));
#52704=CARTESIAN_POINT('',(60.61,66.0787611019615,69.5));
#52705=CARTESIAN_POINT('Origin',(60.61,66.0787611019615,-38.));
#52706=CARTESIAN_POINT('',(69.81,66.0787611019615,-36.5));
#52707=CARTESIAN_POINT('',(69.81,66.0787611019615,-39.5));
#52708=CARTESIAN_POINT('Origin',(69.81,66.0787611019615,-38.));
#52709=CARTESIAN_POINT('',(70.61,66.0787611019615,-39.5));
#52710=CARTESIAN_POINT('',(60.61,66.0787611019615,-39.5));
#52711=CARTESIAN_POINT('',(70.61,66.0787611019615,-36.5));
#52712=CARTESIAN_POINT('Origin',(70.61,66.0787611019615,-38.));
#52713=CARTESIAN_POINT('',(60.61,66.0787611019615,-36.5));
#52714=CARTESIAN_POINT('Origin',(60.61,38.0787611019615,-68.));
#52715=CARTESIAN_POINT('',(69.81,38.0787611019615,-69.5));
#52716=CARTESIAN_POINT('',(69.81,38.0787611019615,-66.5));
#52717=CARTESIAN_POINT('Origin',(69.81,38.0787611019615,-68.));
#52718=CARTESIAN_POINT('',(70.61,38.0787611019615,-69.5));
#52719=CARTESIAN_POINT('',(60.61,38.0787611019615,-69.5));
#52720=CARTESIAN_POINT('',(70.61,38.0787611019615,-66.5));
#52721=CARTESIAN_POINT('Origin',(70.61,38.0787611019615,-68.));
#52722=CARTESIAN_POINT('',(60.61,38.0787611019615,-66.5));
#52723=CARTESIAN_POINT('Origin',(60.61,38.0787611019615,-63.));
#52724=CARTESIAN_POINT('',(69.81,38.0787611019615,-64.5));
#52725=CARTESIAN_POINT('',(69.81,38.0787611019615,-61.5));
#52726=CARTESIAN_POINT('Origin',(69.81,38.0787611019615,-63.));
#52727=CARTESIAN_POINT('',(70.61,38.0787611019615,-64.5));
#52728=CARTESIAN_POINT('',(60.61,38.0787611019615,-64.5));
#52729=CARTESIAN_POINT('',(70.61,38.0787611019615,-61.5));
#52730=CARTESIAN_POINT('Origin',(70.61,38.0787611019615,-63.));
#52731=CARTESIAN_POINT('',(60.61,38.0787611019615,-61.5));
#52732=CARTESIAN_POINT('Origin',(60.61,38.0787611019615,-58.));
#52733=CARTESIAN_POINT('',(69.81,38.0787611019615,-59.5));
#52734=CARTESIAN_POINT('',(69.81,38.0787611019615,-56.5));
#52735=CARTESIAN_POINT('Origin',(69.81,38.0787611019615,-58.));
#52736=CARTESIAN_POINT('',(70.61,38.0787611019615,-59.5));
#52737=CARTESIAN_POINT('',(60.61,38.0787611019615,-59.5));
#52738=CARTESIAN_POINT('',(70.61,38.0787611019615,-56.5));
#52739=CARTESIAN_POINT('Origin',(70.61,38.0787611019615,-58.));
#52740=CARTESIAN_POINT('',(60.61,38.0787611019615,-56.5));
#52741=CARTESIAN_POINT('Origin',(60.61,38.0787611019615,-38.));
#52742=CARTESIAN_POINT('',(69.81,38.0787611019615,-39.5));
#52743=CARTESIAN_POINT('',(69.81,38.0787611019615,-36.5));
#52744=CARTESIAN_POINT('Origin',(69.81,38.0787611019615,-38.));
#52745=CARTESIAN_POINT('',(70.61,38.0787611019615,-39.5));
#52746=CARTESIAN_POINT('',(60.61,38.0787611019615,-39.5));
#52747=CARTESIAN_POINT('',(70.61,38.0787611019615,-36.5));
#52748=CARTESIAN_POINT('Origin',(70.61,38.0787611019615,-38.));
#52749=CARTESIAN_POINT('',(60.61,38.0787611019615,-36.5));
#52750=CARTESIAN_POINT('Origin',(60.61,38.0787611019615,-33.));
#52751=CARTESIAN_POINT('',(69.81,38.0787611019615,-34.5));
#52752=CARTESIAN_POINT('',(69.81,38.0787611019615,-31.5));
#52753=CARTESIAN_POINT('Origin',(69.81,38.0787611019615,-33.));
#52754=CARTESIAN_POINT('',(70.61,38.0787611019615,-34.5));
#52755=CARTESIAN_POINT('',(60.61,38.0787611019615,-34.5));
#52756=CARTESIAN_POINT('',(70.61,38.0787611019615,-31.5));
#52757=CARTESIAN_POINT('Origin',(70.61,38.0787611019615,-33.));
#52758=CARTESIAN_POINT('',(60.61,38.0787611019615,-31.5));
#52759=CARTESIAN_POINT('Origin',(60.61,66.0787611019615,-33.));
#52760=CARTESIAN_POINT('',(69.81,66.0787611019615,-31.5));
#52761=CARTESIAN_POINT('',(69.81,66.0787611019615,-34.5));
#52762=CARTESIAN_POINT('Origin',(69.81,66.0787611019615,-33.));
#52763=CARTESIAN_POINT('',(70.61,66.0787611019615,-34.5));
#52764=CARTESIAN_POINT('',(60.61,66.0787611019615,-34.5));
#52765=CARTESIAN_POINT('',(70.61,66.0787611019615,-31.5));
#52766=CARTESIAN_POINT('Origin',(70.61,66.0787611019615,-33.));
#52767=CARTESIAN_POINT('',(60.61,66.0787611019615,-31.5));
#52768=CARTESIAN_POINT('Origin',(60.61,66.0787611019615,-28.));
#52769=CARTESIAN_POINT('',(69.81,66.0787611019615,-26.5));
#52770=CARTESIAN_POINT('',(69.81,66.0787611019615,-29.5));
#52771=CARTESIAN_POINT('Origin',(69.81,66.0787611019615,-28.));
#52772=CARTESIAN_POINT('',(70.61,66.0787611019615,-29.5));
#52773=CARTESIAN_POINT('',(60.61,66.0787611019615,-29.5));
#52774=CARTESIAN_POINT('',(70.61,66.0787611019615,-26.5));
#52775=CARTESIAN_POINT('Origin',(70.61,66.0787611019615,-28.));
#52776=CARTESIAN_POINT('',(60.61,66.0787611019615,-26.5));
#52777=CARTESIAN_POINT('Origin',(60.61,66.0787611019615,-63.));
#52778=CARTESIAN_POINT('',(69.81,66.0787611019615,-61.5));
#52779=CARTESIAN_POINT('',(69.81,66.0787611019615,-64.5));
#52780=CARTESIAN_POINT('Origin',(69.81,66.0787611019615,-63.));
#52781=CARTESIAN_POINT('',(70.61,66.0787611019615,-64.5));
#52782=CARTESIAN_POINT('',(60.61,66.0787611019615,-64.5));
#52783=CARTESIAN_POINT('',(70.61,66.0787611019615,-61.5));
#52784=CARTESIAN_POINT('Origin',(70.61,66.0787611019615,-63.));
#52785=CARTESIAN_POINT('',(60.61,66.0787611019615,-61.5));
#52786=CARTESIAN_POINT('Origin',(60.61,66.0787611019615,-58.));
#52787=CARTESIAN_POINT('',(69.81,66.0787611019615,-56.5));
#52788=CARTESIAN_POINT('',(69.81,66.0787611019615,-59.5));
#52789=CARTESIAN_POINT('Origin',(69.81,66.0787611019615,-58.));
#52790=CARTESIAN_POINT('',(70.61,66.0787611019615,-59.5));
#52791=CARTESIAN_POINT('',(60.61,66.0787611019615,-59.5));
#52792=CARTESIAN_POINT('',(70.61,66.0787611019615,-56.5));
#52793=CARTESIAN_POINT('Origin',(70.61,66.0787611019615,-58.));
#52794=CARTESIAN_POINT('',(60.61,66.0787611019615,-56.5));
#52795=CARTESIAN_POINT('Origin',(60.61,66.0787611019615,-53.));
#52796=CARTESIAN_POINT('',(69.81,66.0787611019615,-51.5));
#52797=CARTESIAN_POINT('',(69.81,66.0787611019615,-54.5));
#52798=CARTESIAN_POINT('Origin',(69.81,66.0787611019615,-53.));
#52799=CARTESIAN_POINT('',(70.61,66.0787611019615,-54.5));
#52800=CARTESIAN_POINT('',(60.61,66.0787611019615,-54.5));
#52801=CARTESIAN_POINT('',(70.61,66.0787611019615,-51.5));
#52802=CARTESIAN_POINT('Origin',(70.61,66.0787611019615,-53.));
#52803=CARTESIAN_POINT('',(60.61,66.0787611019615,-51.5));
#52804=CARTESIAN_POINT('Origin',(60.61,66.0787611019615,-48.));
#52805=CARTESIAN_POINT('',(69.81,66.0787611019615,-46.5));
#52806=CARTESIAN_POINT('',(69.81,66.0787611019615,-49.5));
#52807=CARTESIAN_POINT('Origin',(69.81,66.0787611019615,-48.));
#52808=CARTESIAN_POINT('',(70.61,66.0787611019615,-49.5));
#52809=CARTESIAN_POINT('',(60.61,66.0787611019615,-49.5));
#52810=CARTESIAN_POINT('',(70.61,66.0787611019615,-46.5));
#52811=CARTESIAN_POINT('Origin',(70.61,66.0787611019615,-48.));
#52812=CARTESIAN_POINT('',(60.61,66.0787611019615,-46.5));
#52813=CARTESIAN_POINT('Origin',(60.61,66.0787611019615,-43.));
#52814=CARTESIAN_POINT('',(69.81,66.0787611019615,-41.5));
#52815=CARTESIAN_POINT('',(69.81,66.0787611019615,-44.5));
#52816=CARTESIAN_POINT('Origin',(69.81,66.0787611019615,-43.));
#52817=CARTESIAN_POINT('',(70.61,66.0787611019615,-44.5));
#52818=CARTESIAN_POINT('',(60.61,66.0787611019615,-44.5));
#52819=CARTESIAN_POINT('',(70.61,66.0787611019615,-41.5));
#52820=CARTESIAN_POINT('Origin',(70.61,66.0787611019615,-43.));
#52821=CARTESIAN_POINT('',(60.61,66.0787611019615,-41.5));
#52822=CARTESIAN_POINT('Origin',(60.61,38.0787611019615,-43.));
#52823=CARTESIAN_POINT('',(69.81,38.0787611019615,-44.5));
#52824=CARTESIAN_POINT('',(69.81,38.0787611019615,-41.5));
#52825=CARTESIAN_POINT('Origin',(69.81,38.0787611019615,-43.));
#52826=CARTESIAN_POINT('',(70.61,38.0787611019615,-44.5));
#52827=CARTESIAN_POINT('',(60.61,38.0787611019615,-44.5));
#52828=CARTESIAN_POINT('',(70.61,38.0787611019615,-41.5));
#52829=CARTESIAN_POINT('Origin',(70.61,38.0787611019615,-43.));
#52830=CARTESIAN_POINT('',(60.61,38.0787611019615,-41.5));
#52831=CARTESIAN_POINT('Origin',(60.61,38.0787611019615,-48.));
#52832=CARTESIAN_POINT('',(69.81,38.0787611019615,-49.5));
#52833=CARTESIAN_POINT('',(69.81,38.0787611019615,-46.5));
#52834=CARTESIAN_POINT('Origin',(69.81,38.0787611019615,-48.));
#52835=CARTESIAN_POINT('',(70.61,38.0787611019615,-49.5));
#52836=CARTESIAN_POINT('',(60.61,38.0787611019615,-49.5));
#52837=CARTESIAN_POINT('',(70.61,38.0787611019615,-46.5));
#52838=CARTESIAN_POINT('Origin',(70.61,38.0787611019615,-48.));
#52839=CARTESIAN_POINT('',(60.61,38.0787611019615,-46.5));
#52840=CARTESIAN_POINT('Origin',(60.61,38.0787611019615,-53.));
#52841=CARTESIAN_POINT('',(69.81,38.0787611019615,-54.5));
#52842=CARTESIAN_POINT('',(69.81,38.0787611019615,-51.5));
#52843=CARTESIAN_POINT('Origin',(69.81,38.0787611019615,-53.));
#52844=CARTESIAN_POINT('',(70.61,38.0787611019615,-54.5));
#52845=CARTESIAN_POINT('',(60.61,38.0787611019615,-54.5));
#52846=CARTESIAN_POINT('',(70.61,38.0787611019615,-51.5));
#52847=CARTESIAN_POINT('Origin',(70.61,38.0787611019615,-53.));
#52848=CARTESIAN_POINT('',(60.61,38.0787611019615,-51.5));
#52849=CARTESIAN_POINT('Origin',(60.61,38.0787611019615,-13.));
#52850=CARTESIAN_POINT('',(69.81,38.0787611019615,-14.5));
#52851=CARTESIAN_POINT('',(69.81,38.0787611019615,-11.5));
#52852=CARTESIAN_POINT('Origin',(69.81,38.0787611019615,-13.));
#52853=CARTESIAN_POINT('',(70.61,38.0787611019615,-14.5));
#52854=CARTESIAN_POINT('',(60.61,38.0787611019615,-14.5));
#52855=CARTESIAN_POINT('',(70.61,38.0787611019615,-11.5));
#52856=CARTESIAN_POINT('Origin',(70.61,38.0787611019615,-13.));
#52857=CARTESIAN_POINT('',(60.61,38.0787611019615,-11.5));
#52858=CARTESIAN_POINT('Origin',(60.61,66.0787611019615,-13.));
#52859=CARTESIAN_POINT('',(69.81,66.0787611019615,-11.5));
#52860=CARTESIAN_POINT('',(69.81,66.0787611019615,-14.5));
#52861=CARTESIAN_POINT('Origin',(69.81,66.0787611019615,-13.));
#52862=CARTESIAN_POINT('',(70.61,66.0787611019615,-14.5));
#52863=CARTESIAN_POINT('',(60.61,66.0787611019615,-14.5));
#52864=CARTESIAN_POINT('',(70.61,66.0787611019615,-11.5));
#52865=CARTESIAN_POINT('Origin',(70.61,66.0787611019615,-13.));
#52866=CARTESIAN_POINT('',(60.61,66.0787611019615,-11.5));
#52867=CARTESIAN_POINT('Origin',(60.61,66.0787611019615,-18.));
#52868=CARTESIAN_POINT('',(69.81,66.0787611019615,-16.5));
#52869=CARTESIAN_POINT('',(69.81,66.0787611019615,-19.5));
#52870=CARTESIAN_POINT('Origin',(69.81,66.0787611019615,-18.));
#52871=CARTESIAN_POINT('',(70.61,66.0787611019615,-19.5));
#52872=CARTESIAN_POINT('',(60.61,66.0787611019615,-19.5));
#52873=CARTESIAN_POINT('',(70.61,66.0787611019615,-16.5));
#52874=CARTESIAN_POINT('Origin',(70.61,66.0787611019615,-18.));
#52875=CARTESIAN_POINT('',(60.61,66.0787611019615,-16.5));
#52876=CARTESIAN_POINT('Origin',(60.61,38.0787611019615,-28.));
#52877=CARTESIAN_POINT('',(69.81,38.0787611019615,-29.5));
#52878=CARTESIAN_POINT('',(69.81,38.0787611019615,-26.5));
#52879=CARTESIAN_POINT('Origin',(69.81,38.0787611019615,-28.));
#52880=CARTESIAN_POINT('',(70.61,38.0787611019615,-29.5));
#52881=CARTESIAN_POINT('',(60.61,38.0787611019615,-29.5));
#52882=CARTESIAN_POINT('',(70.61,38.0787611019615,-26.5));
#52883=CARTESIAN_POINT('Origin',(70.61,38.0787611019615,-28.));
#52884=CARTESIAN_POINT('',(60.61,38.0787611019615,-26.5));
#52885=CARTESIAN_POINT('Origin',(60.61,66.0787611019615,-23.));
#52886=CARTESIAN_POINT('',(69.81,66.0787611019615,-21.5));
#52887=CARTESIAN_POINT('',(69.81,66.0787611019615,-24.5));
#52888=CARTESIAN_POINT('Origin',(69.81,66.0787611019615,-23.));
#52889=CARTESIAN_POINT('',(70.61,66.0787611019615,-24.5));
#52890=CARTESIAN_POINT('',(60.61,66.0787611019615,-24.5));
#52891=CARTESIAN_POINT('',(70.61,66.0787611019615,-21.5));
#52892=CARTESIAN_POINT('Origin',(70.61,66.0787611019615,-23.));
#52893=CARTESIAN_POINT('',(60.61,66.0787611019615,-21.5));
#52894=CARTESIAN_POINT('Origin',(60.61,38.0787611019615,-23.));
#52895=CARTESIAN_POINT('',(69.81,38.0787611019615,-24.5));
#52896=CARTESIAN_POINT('',(69.81,38.0787611019615,-21.5));
#52897=CARTESIAN_POINT('Origin',(69.81,38.0787611019615,-23.));
#52898=CARTESIAN_POINT('',(70.61,38.0787611019615,-24.5));
#52899=CARTESIAN_POINT('',(60.61,38.0787611019615,-24.5));
#52900=CARTESIAN_POINT('',(70.61,38.0787611019615,-21.5));
#52901=CARTESIAN_POINT('Origin',(70.61,38.0787611019615,-23.));
#52902=CARTESIAN_POINT('',(60.61,38.0787611019615,-21.5));
#52903=CARTESIAN_POINT('Origin',(60.61,38.0787611019615,-18.));
#52904=CARTESIAN_POINT('',(69.81,38.0787611019615,-19.5));
#52905=CARTESIAN_POINT('',(69.81,38.0787611019615,-16.5));
#52906=CARTESIAN_POINT('Origin',(69.81,38.0787611019615,-18.));
#52907=CARTESIAN_POINT('',(70.61,38.0787611019615,-19.5));
#52908=CARTESIAN_POINT('',(60.61,38.0787611019615,-19.5));
#52909=CARTESIAN_POINT('',(70.61,38.0787611019615,-16.5));
#52910=CARTESIAN_POINT('Origin',(70.61,38.0787611019615,-18.));
#52911=CARTESIAN_POINT('',(60.61,38.0787611019615,-16.5));
#52912=CARTESIAN_POINT('Origin',(60.61,66.0787611019615,-68.));
#52913=CARTESIAN_POINT('',(69.81,66.0787611019615,-66.5));
#52914=CARTESIAN_POINT('',(69.81,66.0787611019615,-69.5));
#52915=CARTESIAN_POINT('Origin',(69.81,66.0787611019615,-68.));
#52916=CARTESIAN_POINT('',(70.61,66.0787611019615,-69.5));
#52917=CARTESIAN_POINT('',(60.61,66.0787611019615,-69.5));
#52918=CARTESIAN_POINT('',(70.61,66.0787611019615,-66.5));
#52919=CARTESIAN_POINT('Origin',(70.61,66.0787611019615,-68.));
#52920=CARTESIAN_POINT('',(60.61,66.0787611019615,-66.5));
#52921=CARTESIAN_POINT('Origin',(-85.9899999999996,51.6837646578732,-23.6937728532034));
#52922=CARTESIAN_POINT('',(-85.5900000000003,50.5618748736031,-24.689445144648));
#52923=CARTESIAN_POINT('',(-85.5900000000001,50.3847265521965,-22.9437728532035));
#52924=CARTESIAN_POINT('Origin',(-85.59,51.6837646578732,-23.6937728532034));
#52925=CARTESIAN_POINT('',(-86.39,50.5618748740111,-24.6894451438606));
#52926=CARTESIAN_POINT('',(-86.3899999999996,50.5618748736031,-24.689445144648));
#52927=CARTESIAN_POINT('',(-86.39,50.3847265521965,-22.9437728532035));
#52928=CARTESIAN_POINT('Origin',(-86.39,51.6837646578732,-23.6937728532034));
#52929=CARTESIAN_POINT('',(-86.3899999999997,50.3847265521965,-22.9437728532035));
#52930=CARTESIAN_POINT('Origin',(-85.9899999999996,51.6837646578732,-36.3062271467966));
#52931=CARTESIAN_POINT('',(-85.5900000000001,50.3847265521965,-37.0562271467966));
#52932=CARTESIAN_POINT('',(-85.5900000000003,50.5618748736031,-35.310554855352));
#52933=CARTESIAN_POINT('Origin',(-85.59,51.6837646578732,-36.3062271467966));
#52934=CARTESIAN_POINT('',(-86.39,50.3847265521965,-37.0562271467966));
#52935=CARTESIAN_POINT('',(-85.5899999999991,50.3847265521965,-37.0562271467966));
#52936=CARTESIAN_POINT('',(-86.39,50.5618748739028,-35.3105548560302));
#52937=CARTESIAN_POINT('Origin',(-86.39,51.6837646578732,-36.3062271467966));
#52938=CARTESIAN_POINT('',(-85.5900000000004,50.5618748736031,-35.310554855352));
#52939=CARTESIAN_POINT('Origin',(-85.9899999999998,28.8625290471562,-27.));
#52940=CARTESIAN_POINT('',(-85.5900000000001,28.8625290471562,-28.5));
#52941=CARTESIAN_POINT('',(-85.5900000000002,27.3891253349642,-26.7187856673305));
#52942=CARTESIAN_POINT('Origin',(-85.59,28.8625290471562,-27.));
#52943=CARTESIAN_POINT('',(-86.39,28.8625290471562,-28.5));
#52944=CARTESIAN_POINT('',(-85.5899999999995,28.8625290471562,-28.5));
#52945=CARTESIAN_POINT('',(-86.39,27.3891253344444,-26.7187856670729));
#52946=CARTESIAN_POINT('Origin',(-86.39,28.8625290471562,-27.));
#52947=CARTESIAN_POINT('',(-85.5900000000002,27.3891253349642,-26.7187856673305));
#52948=CARTESIAN_POINT('Origin',(-85.9899999999998,28.8625290471562,-33.));
#52949=CARTESIAN_POINT('',(-85.5900000000001,27.3891253349642,-33.2812143326694));
#52950=CARTESIAN_POINT('',(-85.5900000000001,28.8625290471562,-31.5));
#52951=CARTESIAN_POINT('Origin',(-85.59,28.8625290471562,-33.));
#52952=CARTESIAN_POINT('',(-86.39,27.3891253342258,-33.2812143328545));
#52953=CARTESIAN_POINT('',(-86.39,27.3891253349642,-33.2812143326695));
#52954=CARTESIAN_POINT('',(-86.39,28.8625290471562,-31.5));
#52955=CARTESIAN_POINT('Origin',(-86.39,28.8625290471562,-33.));
#52956=CARTESIAN_POINT('',(-86.3900000000002,28.8625290471562,-31.5));
#52957=CARTESIAN_POINT('Origin',(-85.9899999999998,39.3187444720575,-45.1106160516509));
#52958=CARTESIAN_POINT('',(-85.59,38.8257009268133,-46.5272698775706));
#52959=CARTESIAN_POINT('',(-85.5900000000001,38.0197063663809,-44.3606160516509));
#52960=CARTESIAN_POINT('Origin',(-85.59,39.3187444720575,-45.1106160516509));
#52961=CARTESIAN_POINT('',(-86.39,38.825700926233,-46.5272698779012));
#52962=CARTESIAN_POINT('',(-86.3900000000002,38.8257009268133,-46.5272698775706));
#52963=CARTESIAN_POINT('',(-86.39,38.0197063663809,-44.3606160516509));
#52964=CARTESIAN_POINT('Origin',(-86.39,39.3187444720575,-45.1106160516509));
#52965=CARTESIAN_POINT('',(-86.3900000000002,38.0197063663809,-44.3606160516509));
#52966=CARTESIAN_POINT('Origin',(-85.9899999999998,39.3187444720576,-14.8893839483491));
#52967=CARTESIAN_POINT('',(-85.5900000000001,38.0197063663809,-15.6393839483491));
#52968=CARTESIAN_POINT('',(-85.59,38.8257009268133,-13.4727301224294));
#52969=CARTESIAN_POINT('Origin',(-85.59,39.3187444720576,-14.8893839483491));
#52970=CARTESIAN_POINT('',(-86.39,38.0197063663809,-15.6393839483491));
#52971=CARTESIAN_POINT('',(-85.5899999999993,38.0197063663809,-15.6393839483491));
#52972=CARTESIAN_POINT('',(-86.3900000000001,38.8257009252949,-13.4727301229578));
#52973=CARTESIAN_POINT('Origin',(-86.39,39.3187444720576,-14.8893839483491));
#52974=CARTESIAN_POINT('',(-85.5900000000001,38.8257009268133,-13.4727301224294));
#52975=CARTESIAN_POINT('Origin',(-85.9899999999998,58.0740500613155,-12.6254738595756));
#52976=CARTESIAN_POINT('',(-85.5900000000001,57.1538693431447,-13.8100697594109));
#52977=CARTESIAN_POINT('',(-85.5900000000001,56.7750119556388,-11.8754738595756));
#52978=CARTESIAN_POINT('Origin',(-85.59,58.0740500613155,-12.6254738595756));
#52979=CARTESIAN_POINT('',(-86.39,57.1538693432358,-13.8100697584817));
#52980=CARTESIAN_POINT('',(-86.3900000000001,57.1538693431447,-13.8100697594109));
#52981=CARTESIAN_POINT('',(-86.39,56.7750119556388,-11.8754738595756));
#52982=CARTESIAN_POINT('Origin',(-86.39,58.0740500613155,-12.6254738595756));
#52983=CARTESIAN_POINT('',(-86.3900000000001,56.7750119556388,-11.8754738595756));
#52984=CARTESIAN_POINT('Origin',(-85.9899999999996,58.0740500613155,-47.3745261404244));
#52985=CARTESIAN_POINT('',(-85.5900000000001,56.7750119556388,-48.1245261404244));
#52986=CARTESIAN_POINT('',(-85.59,57.1538693431447,-46.1899302405891));
#52987=CARTESIAN_POINT('Origin',(-85.59,58.0740500613155,-47.3745261404244));
#52988=CARTESIAN_POINT('',(-86.39,56.7750119556388,-48.1245261404244));
#52989=CARTESIAN_POINT('',(-85.5899999999992,56.7750119556388,-48.1245261404244));
#52990=CARTESIAN_POINT('',(-86.39,57.1538693431799,-46.1899302415125));
#52991=CARTESIAN_POINT('Origin',(-86.39,58.0740500613155,-47.3745261404244));
#52992=CARTESIAN_POINT('',(-85.59,57.1538693431447,-46.1899302405891));
#52993=CARTESIAN_POINT('Origin',(-85.9899999999995,16.7400532252403,-27.));
#52994=CARTESIAN_POINT('',(-85.5900000000001,16.7400532252403,-28.5));
#52995=CARTESIAN_POINT('',(-85.59,15.2486853399007,-26.8393082747068));
#52996=CARTESIAN_POINT('Origin',(-85.59,16.7400532252403,-27.));
#52997=CARTESIAN_POINT('',(-86.39,16.7400532252403,-28.5));
#52998=CARTESIAN_POINT('',(-85.5899999999992,16.7400532252403,-28.5));
#52999=CARTESIAN_POINT('',(-86.39,15.2486853393764,-26.8393082746143));
#53000=CARTESIAN_POINT('Origin',(-86.39,16.7400532252403,-27.));
#53001=CARTESIAN_POINT('',(-85.5900000000001,15.2486853399007,-26.8393082747068));
#53002=CARTESIAN_POINT('Origin',(-85.9899999999995,16.7400532252403,-33.));
#53003=CARTESIAN_POINT('',(-85.59,15.2486853399007,-33.1606917252932));
#53004=CARTESIAN_POINT('',(-85.5900000000001,16.7400532252403,-31.5));
#53005=CARTESIAN_POINT('Origin',(-85.59,16.7400532252403,-33.));
#53006=CARTESIAN_POINT('',(-86.39,15.2486853407812,-33.1606917252392));
#53007=CARTESIAN_POINT('',(-86.3899999999997,15.2486853399007,-33.1606917252932));
#53008=CARTESIAN_POINT('',(-86.39,16.7400532252403,-31.5));
#53009=CARTESIAN_POINT('Origin',(-86.39,16.7400532252403,-33.));
#53010=CARTESIAN_POINT('',(-86.3899999999997,16.7400532252403,-31.5));
#53011=CARTESIAN_POINT('Origin',(-85.9899999999996,33.2574367244157,-55.6091090308774));
#53012=CARTESIAN_POINT('',(-85.59,32.6508629759236,-56.980993970528));
#53013=CARTESIAN_POINT('',(-85.5900000000001,31.9583986187391,-54.8591090308774));
#53014=CARTESIAN_POINT('Origin',(-85.59,33.2574367244157,-55.6091090308774));
#53015=CARTESIAN_POINT('',(-86.39,32.6508629762386,-56.9809939712314));
#53016=CARTESIAN_POINT('',(-86.3899999999996,32.6508629759238,-56.9809939705281));
#53017=CARTESIAN_POINT('',(-86.39,31.9583986187391,-54.8591090308774));
#53018=CARTESIAN_POINT('Origin',(-86.39,33.2574367244157,-55.6091090308774));
#53019=CARTESIAN_POINT('',(-86.3899999999997,31.9583986187391,-54.8591090308774));
#53020=CARTESIAN_POINT('Origin',(-85.9899999999995,33.2574367244158,-4.3908909691226));
#53021=CARTESIAN_POINT('',(-85.5900000000001,31.9583986187391,-5.14089096912259));
#53022=CARTESIAN_POINT('',(-85.59,32.6508629759237,-3.01900602947195));
#53023=CARTESIAN_POINT('Origin',(-85.59,33.2574367244158,-4.3908909691226));
#53024=CARTESIAN_POINT('',(-86.39,31.9583986187391,-5.14089096912259));
#53025=CARTESIAN_POINT('',(-85.5899999999992,31.9583986187391,-5.1408909691226));
#53026=CARTESIAN_POINT('',(-86.39,32.6508629756065,-3.01900602877295));
#53027=CARTESIAN_POINT('Origin',(-86.39,33.2574367244158,-4.3908909691226));
#53028=CARTESIAN_POINT('',(-85.5900000000001,32.6508629759238,-3.0190060294719));
#53029=CARTESIAN_POINT('Origin',(-85.9899999999993,64.1105207282856,-2.16999996598415));
#53030=CARTESIAN_POINT('',(-85.5899999999999,63.2487659305948,-3.39775347082817));
#53031=CARTESIAN_POINT('',(-85.5900000000001,62.811482622609,-1.41999996598415));
#53032=CARTESIAN_POINT('Origin',(-85.59,64.1105207282856,-2.16999996598415));
#53033=CARTESIAN_POINT('',(-86.39,63.2487659307941,-3.39775346999418));
#53034=CARTESIAN_POINT('',(-86.39,63.2487659305948,-3.39775347082816));
#53035=CARTESIAN_POINT('',(-86.39,62.811482622609,-1.41999996598415));
#53036=CARTESIAN_POINT('Origin',(-86.39,64.1105207282856,-2.16999996598415));
#53037=CARTESIAN_POINT('',(-86.3899999999996,62.811482622609,-1.41999996598415));
#53038=CARTESIAN_POINT('Origin',(-85.9899999999999,64.1105207282856,-57.8300000340159));
#53039=CARTESIAN_POINT('',(-85.5900000000001,62.8114826226089,-58.5800000340159));
#53040=CARTESIAN_POINT('',(-85.5900000000001,63.2487659305946,-56.6022465291719));
#53041=CARTESIAN_POINT('Origin',(-85.59,64.1105207282856,-57.8300000340159));
#53042=CARTESIAN_POINT('',(-86.39,62.8114826226089,-58.5800000340159));
#53043=CARTESIAN_POINT('',(-85.5899999999994,62.8114826226089,-58.5800000340159));
#53044=CARTESIAN_POINT('',(-86.39,63.248765930775,-56.602246529842));
#53045=CARTESIAN_POINT('Origin',(-86.39,64.1105207282856,-57.8300000340159));
#53046=CARTESIAN_POINT('',(-85.5900000000001,63.2487659305946,-56.602246529172));
#53047=CARTESIAN_POINT('Origin',(-85.9900000001603,27.9852423132283,4.74081761843475));
#53048=CARTESIAN_POINT('',(-85.59,26.6862042075517,3.99081761843476));
#53049=CARTESIAN_POINT('',(-85.5899999999998,27.3389968866617,6.09446707403308));
#53050=CARTESIAN_POINT('Origin',(-85.59,27.9852423132283,4.74081761843475));
#53051=CARTESIAN_POINT('',(-86.39,26.6862042075517,3.99081761843476));
#53052=CARTESIAN_POINT('',(913.61,26.6862042075521,3.99081761843475));
#53053=CARTESIAN_POINT('',(-86.3899999999999,27.3389968866617,6.09446707403308));
#53054=CARTESIAN_POINT('Origin',(-86.39,27.9852423132283,4.74081761843475));
#53055=CARTESIAN_POINT('',(-85.5899999999998,27.3389968866617,6.09446707403308));
#53056=CARTESIAN_POINT('Origin',(-85.9900000000819,6.19540997866983,-27.));
#53057=CARTESIAN_POINT('',(-85.5900000000001,6.19540997866983,-28.5));
#53058=CARTESIAN_POINT('',(-85.59,4.69995568091292,-26.8833104832455));
#53059=CARTESIAN_POINT('Origin',(-85.59,6.19540997866983,-27.));
#53060=CARTESIAN_POINT('',(-86.39,6.19540997866983,-28.5));
#53061=CARTESIAN_POINT('',(913.61,6.19540997867027,-28.5));
#53062=CARTESIAN_POINT('',(-86.39,4.69995568091292,-26.8833104832455));
#53063=CARTESIAN_POINT('Origin',(-86.39,6.19540997866983,-27.));
#53064=CARTESIAN_POINT('',(-85.59,4.69995568091292,-26.8833104832455));
#53065=CARTESIAN_POINT('Origin',(-85.99,6.19541004646761,-33.));
#53066=CARTESIAN_POINT('',(-85.5899999999999,4.69995574181559,-33.1166894283889));
#53067=CARTESIAN_POINT('',(-85.5900000000001,6.19541004646761,-31.5));
#53068=CARTESIAN_POINT('Origin',(-85.59,6.19541004646761,-33.));
#53069=CARTESIAN_POINT('',(-86.3899999999999,4.69995574181559,-33.1166894283889));
#53070=CARTESIAN_POINT('',(-86.3899999999999,4.69995574181558,-33.1166894283889));
#53071=CARTESIAN_POINT('',(-86.39,6.19541004646761,-31.5));
#53072=CARTESIAN_POINT('Origin',(-86.39,6.19541004646761,-33.));
#53073=CARTESIAN_POINT('',(913.61,6.19541004646805,-31.5));
#53074=CARTESIAN_POINT('Origin',(-85.9900000000002,27.9852422140127,-64.7408177902812));
#53075=CARTESIAN_POINT('',(-85.5899999999997,27.338996733446,-66.0944672200995));
#53076=CARTESIAN_POINT('',(-85.59,26.686204108336,-63.9908177902812));
#53077=CARTESIAN_POINT('Origin',(-85.59,27.9852422140127,-64.7408177902812));
#53078=CARTESIAN_POINT('',(-86.3899999999998,27.338996733446,-66.0944672200995));
#53079=CARTESIAN_POINT('',(-86.3899999999999,27.338996733446,-66.0944672200995));
#53080=CARTESIAN_POINT('',(-86.39,26.686204108336,-63.9908177902812));
#53081=CARTESIAN_POINT('Origin',(-86.39,27.9852422140127,-64.7408177902812));
#53082=CARTESIAN_POINT('',(913.61,26.6862041083364,-63.9908177902812));
#53083=CARTESIAN_POINT('Ctrl Pts',(-85.5900000000001,42.9713195513441,-22.1631559443849));
#53084=CARTESIAN_POINT('Ctrl Pts',(-86.55,42.9713195513441,-22.1631559443849));
#53085=CARTESIAN_POINT('Ctrl Pts',(-85.5900000000001,42.9868830995498,-22.1599633677126));
#53086=CARTESIAN_POINT('Ctrl Pts',(-86.55,42.9868830995498,-22.1599633677126));
#53087=CARTESIAN_POINT('Ctrl Pts',(-85.5900000000001,43.5156846168693,-22.0531343444844));
#53088=CARTESIAN_POINT('Ctrl Pts',(-86.55,43.5156846168693,-22.0531343444844));
#53089=CARTESIAN_POINT('Ctrl Pts',(-85.5900000000002,44.0551666698534,-22.));
#53090=CARTESIAN_POINT('Ctrl Pts',(-86.5500000000001,44.0551666698534,-22.));
#53091=CARTESIAN_POINT('Ctrl Pts',(-85.5900000000002,44.5787611019615,-22.));
#53092=CARTESIAN_POINT('Ctrl Pts',(-86.5500000000001,44.5787611019615,-22.));
#53093=CARTESIAN_POINT('',(-85.5900000000004,44.5787611019615,-22.));
#53094=CARTESIAN_POINT('',(-85.5900000000003,42.9713195513605,-22.1631559443815));
#53095=CARTESIAN_POINT('Ctrl Pts',(-85.5900000000003,44.5787611019615,-22.));
#53096=CARTESIAN_POINT('Ctrl Pts',(-85.5900000000003,44.0551666698534,-22.));
#53097=CARTESIAN_POINT('Ctrl Pts',(-85.5900000000001,43.5315722377453,-22.0515695504083));
#53098=CARTESIAN_POINT('Ctrl Pts',(-85.5900000000001,43.0180385258325,-22.1537177567742));
#53099=CARTESIAN_POINT('Ctrl Pts',(-85.5900000000001,43.0024561811422,-22.1568172778458));
#53100=CARTESIAN_POINT('Ctrl Pts',(-85.5900000000001,42.9868830995607,-22.1599633677104));
#53101=CARTESIAN_POINT('Ctrl Pts',(-85.5900000000001,42.9713195513605,-22.1631559443815));
#53102=CARTESIAN_POINT('',(-86.39,44.5787611019615,-22.));
#53103=CARTESIAN_POINT('',(913.61,44.578761101962,-22.));
#53104=CARTESIAN_POINT('',(-86.39,42.9713195515195,-22.1631559452401));
#53105=CARTESIAN_POINT('Ctrl Pts',(-86.3899999999999,42.9713195513441,-22.1631559443849));
#53106=CARTESIAN_POINT('Ctrl Pts',(-86.3899999999999,42.9868830995498,-22.1599633677126));
#53107=CARTESIAN_POINT('Ctrl Pts',(-86.3899999999999,43.0024561811367,-22.1568172778469));
#53108=CARTESIAN_POINT('Ctrl Pts',(-86.3899999999999,43.0180385258325,-22.1537177567742));
#53109=CARTESIAN_POINT('Ctrl Pts',(-86.3899999999999,43.5315722377453,-22.0515695504083));
#53110=CARTESIAN_POINT('Ctrl Pts',(-86.39,44.0551666698534,-22.));
#53111=CARTESIAN_POINT('Ctrl Pts',(-86.39,44.5787611019615,-22.));
#53112=CARTESIAN_POINT('',(-86.3899999999997,42.9713195513605,-22.1631559443815));
#53113=CARTESIAN_POINT('Ctrl Pts',(-85.59,36.8454205805627,-11.0146003459994));
#53114=CARTESIAN_POINT('Ctrl Pts',(-86.55,36.8454205805627,-11.0146003459994));
#53115=CARTESIAN_POINT('Ctrl Pts',(-85.59,38.0507425034688,-10.5236598584192));
#53116=CARTESIAN_POINT('Ctrl Pts',(-86.55,38.0507425034688,-10.5236598584192));
#53117=CARTESIAN_POINT('Ctrl Pts',(-85.59,40.5938700965656,-9.76033053442545));
#53118=CARTESIAN_POINT('Ctrl Pts',(-86.5499999999999,40.5938700965656,-9.76033053442545));
#53119=CARTESIAN_POINT('Ctrl Pts',(-85.5900000000001,43.2370503696844,-9.5));
#53120=CARTESIAN_POINT('Ctrl Pts',(-86.5500000000001,43.2370503696844,-9.5));
#53121=CARTESIAN_POINT('Ctrl Pts',(-85.5900000000001,44.5787611019615,-9.5));
#53122=CARTESIAN_POINT('Ctrl Pts',(-86.5500000000001,44.5787611019615,-9.5));
#53123=CARTESIAN_POINT('',(-85.5900000000001,44.5787611019615,-9.5));
#53124=CARTESIAN_POINT('',(-85.59,36.8454205811755,-11.0146003457498));
#53125=CARTESIAN_POINT('Ctrl Pts',(-85.5900000000001,44.5787611019615,-9.5));
#53126=CARTESIAN_POINT('Ctrl Pts',(-85.5900000000001,43.2370503696844,-9.5));
#53127=CARTESIAN_POINT('Ctrl Pts',(-85.59,40.5938700967862,-9.76033053440373));
#53128=CARTESIAN_POINT('Ctrl Pts',(-85.59,38.0507425038933,-10.5236598582919));
#53129=CARTESIAN_POINT('Ctrl Pts',(-85.59,36.8454205811755,-11.0146003457498));
#53130=CARTESIAN_POINT('',(-86.39,44.5787611019615,-9.5));
#53131=CARTESIAN_POINT('',(913.61,44.578761101962,-9.5));
#53132=CARTESIAN_POINT('',(-86.39,36.8454205803542,-11.0146003454874));
#53133=CARTESIAN_POINT('Ctrl Pts',(-86.3899999999999,36.8454205805627,-11.0146003459994));
#53134=CARTESIAN_POINT('Ctrl Pts',(-86.3899999999999,38.0507425034688,-10.5236598584192));
#53135=CARTESIAN_POINT('Ctrl Pts',(-86.3899999999999,40.5938700965656,-9.76033053442545));
#53136=CARTESIAN_POINT('Ctrl Pts',(-86.39,43.2370503696844,-9.5));
#53137=CARTESIAN_POINT('Ctrl Pts',(-86.39,44.5787611019615,-9.5));
#53138=CARTESIAN_POINT('',(-86.39,36.8454205811755,-11.0146003457498));
#53139=CARTESIAN_POINT('Ctrl Pts',(-85.59,50.3318213149459,-13.4727301355976));
#53140=CARTESIAN_POINT('Ctrl Pts',(-86.5500000000005,50.3318213149459,-13.4727301355976));
#53141=CARTESIAN_POINT('Ctrl Pts',(-85.59,49.5680966220862,-13.206928056047));
#53142=CARTESIAN_POINT('Ctrl Pts',(-86.5500000000006,49.5680966220862,-13.206928056047));
#53143=CARTESIAN_POINT('Ctrl Pts',(-85.5900000000001,47.6781372544074,-12.6924535152679));
#53144=CARTESIAN_POINT('Ctrl Pts',(-86.5500000000007,47.6781372544074,-12.6924535152679));
#53145=CARTESIAN_POINT('Ctrl Pts',(-85.5899999999996,45.7241239221981,-12.5));
#53146=CARTESIAN_POINT('Ctrl Pts',(-86.5500000000002,45.7241239221981,-12.5));
#53147=CARTESIAN_POINT('Ctrl Pts',(-85.5899999999996,44.5787611019615,-12.5));
#53148=CARTESIAN_POINT('Ctrl Pts',(-86.5500000000002,44.5787611019615,-12.5));
#53149=CARTESIAN_POINT('',(-85.5900000000002,50.3318212771098,-13.4727301224294));
#53150=CARTESIAN_POINT('',(-85.5899999999998,44.5787611019615,-12.5));
#53151=CARTESIAN_POINT('Ctrl Pts',(-85.5900000000002,50.3318212771098,-13.4727301224294));
#53152=CARTESIAN_POINT('Ctrl Pts',(-85.5900000000002,49.5680965962538,-13.2069280490151));
#53153=CARTESIAN_POINT('Ctrl Pts',(-85.5900000000003,47.6781372410534,-12.6924535139526));
#53154=CARTESIAN_POINT('Ctrl Pts',(-85.5899999999999,45.7241239221981,-12.5));
#53155=CARTESIAN_POINT('Ctrl Pts',(-85.5899999999998,44.5787611019615,-12.5));
#53156=CARTESIAN_POINT('',(-86.39,44.5787611019615,-12.5));
#53157=CARTESIAN_POINT('',(913.61,44.578761101962,-12.5));
#53158=CARTESIAN_POINT('',(-86.3900000000001,50.3318212785861,-13.4727301229432));
#53159=CARTESIAN_POINT('Ctrl Pts',(-86.3900000000002,50.3318212785861,-13.4727301229432));
#53160=CARTESIAN_POINT('Ctrl Pts',(-86.3900000000003,49.5680965972618,-13.2069280492894));
#53161=CARTESIAN_POINT('Ctrl Pts',(-86.3900000000004,47.6781372415745,-12.692453514004));
#53162=CARTESIAN_POINT('Ctrl Pts',(-86.3899999999999,45.7241239221981,-12.5));
#53163=CARTESIAN_POINT('Ctrl Pts',(-86.3899999999998,44.5787611019615,-12.5));
#53164=CARTESIAN_POINT('',(-86.3900000000003,50.3318212771098,-13.4727301224294));
#53165=CARTESIAN_POINT('Ctrl Pts',(-85.5899999999998,30.8757056257453,-0.530143046109299));
#53166=CARTESIAN_POINT('Ctrl Pts',(-86.55,30.8757056257453,-0.530143046109299));
#53167=CARTESIAN_POINT('Ctrl Pts',(-85.5899999999998,31.2936434644341,-0.335776881547456));
#53168=CARTESIAN_POINT('Ctrl Pts',(-86.55,31.2936434644341,-0.335776881547456));
#53169=CARTESIAN_POINT('Ctrl Pts',(-85.5899999999998,33.6635280544018,0.70564601555246));
#53170=CARTESIAN_POINT('Ctrl Pts',(-86.55,33.6635280544018,0.70564601555246));
#53171=CARTESIAN_POINT('Ctrl Pts',(-85.5899999999998,38.1974539606436,2.08099740293234));
#53172=CARTESIAN_POINT('Ctrl Pts',(-86.55,38.1974539606436,2.08099740293234));
#53173=CARTESIAN_POINT('Ctrl Pts',(-85.5899999999998,42.4516587215222,2.5));
#53174=CARTESIAN_POINT('Ctrl Pts',(-86.55,42.4516587215222,2.5));
#53175=CARTESIAN_POINT('Ctrl Pts',(-85.5899999999998,44.5787611019615,2.5));
#53176=CARTESIAN_POINT('Ctrl Pts',(-86.55,44.5787611019615,2.5));
#53177=CARTESIAN_POINT('',(-85.59,44.5787611019615,2.5));
#53178=CARTESIAN_POINT('',(-85.5900000000001,30.8757056257996,-0.53014304608406));
#53179=CARTESIAN_POINT('Ctrl Pts',(-85.59,44.5787611019615,2.5));
#53180=CARTESIAN_POINT('Ctrl Pts',(-85.5900000000001,42.4516587215222,2.5));
#53181=CARTESIAN_POINT('Ctrl Pts',(-85.5900000000001,38.1974539606436,2.08099740293234));
#53182=CARTESIAN_POINT('Ctrl Pts',(-85.5900000000001,33.6635280544172,0.705646015557152));
#53183=CARTESIAN_POINT('Ctrl Pts',(-85.5900000000001,31.2936434644636,-0.335776881534512));
#53184=CARTESIAN_POINT('Ctrl Pts',(-85.5900000000001,30.8757056257996,-0.53014304608406));
#53185=CARTESIAN_POINT('',(-86.39,44.5787611019615,2.5));
#53186=CARTESIAN_POINT('',(913.61,44.578761101962,2.5));
#53187=CARTESIAN_POINT('',(-86.39,30.8757056270897,-0.530143045484072));
#53188=CARTESIAN_POINT('Ctrl Pts',(-86.39,30.8757056270897,-0.530143045484066));
#53189=CARTESIAN_POINT('Ctrl Pts',(-86.39,31.2936434644341,-0.335776881547456));
#53190=CARTESIAN_POINT('Ctrl Pts',(-86.39,33.6635280544018,0.70564601555246));
#53191=CARTESIAN_POINT('Ctrl Pts',(-86.39,38.1974539606436,2.08099740293234));
#53192=CARTESIAN_POINT('Ctrl Pts',(-86.39,42.4516587215222,2.5));
#53193=CARTESIAN_POINT('Ctrl Pts',(-86.39,44.5787611019615,2.5));
#53194=CARTESIAN_POINT('',(-86.39,30.8757056258048,-0.530143046081613));
#53195=CARTESIAN_POINT('Ctrl Pts',(-85.5899999999995,56.5066592280182,-3.0190060294803));
#53196=CARTESIAN_POINT('Ctrl Pts',(-86.5500000000001,56.5066592280182,-3.0190060294803));
#53197=CARTESIAN_POINT('Ctrl Pts',(-85.5899999999995,56.2948319481592,-2.92534739713906));
#53198=CARTESIAN_POINT('Ctrl Pts',(-86.5500000000001,56.2948319481592,-2.92534739713906));
#53199=CARTESIAN_POINT('Ctrl Pts',(-85.5899999999995,54.3068457690469,-2.07424376132673));
#53200=CARTESIAN_POINT('Ctrl Pts',(-86.5500000000001,54.3068457690469,-2.07424376132673));
#53201=CARTESIAN_POINT('Ctrl Pts',(-85.5899999999994,50.3710245071578,-0.880325434261424));
#53202=CARTESIAN_POINT('Ctrl Pts',(-86.5499999999999,50.3710245071578,-0.880325434261424));
#53203=CARTESIAN_POINT('Ctrl Pts',(-85.5899999999998,46.5095155703603,-0.500000000000001));
#53204=CARTESIAN_POINT('Ctrl Pts',(-86.5500000000004,46.5095155703603,-0.500000000000001));
#53205=CARTESIAN_POINT('Ctrl Pts',(-85.5899999999998,44.5787611019615,-0.5));
#53206=CARTESIAN_POINT('Ctrl Pts',(-86.5500000000004,44.5787611019615,-0.5));
#53207=CARTESIAN_POINT('',(-85.59,56.5066592279994,-3.01900602947196));
#53208=CARTESIAN_POINT('',(-85.5900000000003,44.5787611019615,-0.5));
#53209=CARTESIAN_POINT('Ctrl Pts',(-85.59,56.5066592279994,-3.01900602947196));
#53210=CARTESIAN_POINT('Ctrl Pts',(-85.59,56.2948319481467,-2.92534739713372));
#53211=CARTESIAN_POINT('Ctrl Pts',(-85.59,54.3068457690404,-2.07424376132475));
#53212=CARTESIAN_POINT('Ctrl Pts',(-85.5899999999998,50.3710245071578,-0.880325434261424));
#53213=CARTESIAN_POINT('Ctrl Pts',(-85.5900000000003,46.5095155703603,-0.500000000000001));
#53214=CARTESIAN_POINT('Ctrl Pts',(-85.5900000000003,44.5787611019615,-0.5));
#53215=CARTESIAN_POINT('',(-86.39,44.5787611019615,-0.5));
#53216=CARTESIAN_POINT('',(913.61,44.578761101962,-0.5));
#53217=CARTESIAN_POINT('',(-86.39,56.5066592282128,-3.01900602900217));
#53218=CARTESIAN_POINT('Ctrl Pts',(-86.3899999999997,56.5066592280182,-3.0190060294803));
#53219=CARTESIAN_POINT('Ctrl Pts',(-86.3899999999997,56.2948319481592,-2.92534739713906));
#53220=CARTESIAN_POINT('Ctrl Pts',(-86.3899999999997,54.3068457690469,-2.07424376132673));
#53221=CARTESIAN_POINT('Ctrl Pts',(-86.3899999999995,50.3710245071578,-0.880325434261424));
#53222=CARTESIAN_POINT('Ctrl Pts',(-86.39,46.5095155703603,-0.500000000000001));
#53223=CARTESIAN_POINT('Ctrl Pts',(-86.39,44.5787611019615,-0.5));
#53224=CARTESIAN_POINT('',(-86.3899999999997,56.5066592279993,-3.01900602947191));
#53225=CARTESIAN_POINT('Origin',(-74.39,80.0825925853381,-65.5038314833765));
#53226=CARTESIAN_POINT('',(-83.59,81.8325925853381,-65.5038314833765));
#53227=CARTESIAN_POINT('Origin',(-83.59,80.0825925853381,-65.5038314833765));
#53228=CARTESIAN_POINT('',(-84.39,81.8325925853381,-65.5038314833765));
#53229=CARTESIAN_POINT('',(-74.39,81.8325925853381,-65.5038314833765));
#53230=CARTESIAN_POINT('Origin',(-84.39,80.0825925853381,-65.5038314833765));
#53231=CARTESIAN_POINT('Origin',(-74.39,9.0749296185849,-65.5038314833765));
#53232=CARTESIAN_POINT('',(-83.59,10.8249296185849,-65.5038314833765));
#53233=CARTESIAN_POINT('Origin',(-83.59,9.07492961858489,-65.5038314833765));
#53234=CARTESIAN_POINT('',(-84.39,10.8249296185849,-65.5038314833765));
#53235=CARTESIAN_POINT('',(-74.39,10.8249296185849,-65.5038314833765));
#53236=CARTESIAN_POINT('Origin',(-84.39,9.07492961858489,-65.5038314833765));
#53237=CARTESIAN_POINT('Origin',(-74.39,9.0749296185849,5.50383148337648));
#53238=CARTESIAN_POINT('',(-83.59,10.8249296185849,5.50383148337648));
#53239=CARTESIAN_POINT('Origin',(-83.59,9.07492961858489,5.50383148337648));
#53240=CARTESIAN_POINT('',(-84.39,10.8249296185849,5.50383148337648));
#53241=CARTESIAN_POINT('',(-74.39,10.8249296185849,5.50383148337648));
#53242=CARTESIAN_POINT('Origin',(-84.39,9.07492961858489,5.50383148337648));
#53243=CARTESIAN_POINT('Origin',(-74.39,80.0825925853381,5.50383148337648));
#53244=CARTESIAN_POINT('',(-83.59,81.8325925853382,5.50383148337648));
#53245=CARTESIAN_POINT('Origin',(-83.59,80.0825925853381,5.50383148337648));
#53246=CARTESIAN_POINT('',(-84.39,81.8325925853382,5.50383148337648));
#53247=CARTESIAN_POINT('',(-74.39,81.8325925853382,5.50383148337648));
#53248=CARTESIAN_POINT('Origin',(-84.39,80.0825925853381,5.50383148337648));
#53249=CARTESIAN_POINT('Origin',(-85.09,44.5787611019615,-30.));
#53250=CARTESIAN_POINT('',(-85.1899999999999,44.5787611019615,-72.4898979485563));
#53251=CARTESIAN_POINT('Origin',(-85.1899999999999,44.5787611019615,-30.));
#53252=CARTESIAN_POINT('',(-85.59,44.5787611019615,-72.));
#53253=CARTESIAN_POINT('Origin',(-85.09,44.5787611019615,-72.));
#53254=CARTESIAN_POINT('Origin',(-85.59,44.5787611019615,-30.));
#53255=CARTESIAN_POINT('Origin',(-85.59,44.5787611019615,-30.));
#53256=CARTESIAN_POINT('',(-85.35,44.5787611019615,-73.2737346662473));
#53257=CARTESIAN_POINT('Origin',(-85.35,44.5787611019615,-30.));
#53258=CARTESIAN_POINT('',(-84.39,44.5787611019615,-74.4494897427832));
#53259=CARTESIAN_POINT('Origin',(-85.59,44.5787611019615,-74.4494897427832));
#53260=CARTESIAN_POINT('Origin',(-84.39,44.5787611019615,-30.));
#53261=CARTESIAN_POINT('Origin',(-85.09,44.5787611019615,-30.));
#53262=CARTESIAN_POINT('',(-86.39,44.5787611019615,-72.));
#53263=CARTESIAN_POINT('Origin',(-86.39,44.5787611019615,-30.));
#53264=CARTESIAN_POINT('Origin',(-85.09,44.5787611019615,-72.));
#53265=CARTESIAN_POINT('Origin',(-85.59,44.5787611019615,-30.));
#53266=CARTESIAN_POINT('',(-83.59,44.5787611019615,-74.4494897427832));
#53267=CARTESIAN_POINT('Origin',(-83.59,44.5787611019615,-30.));
#53268=CARTESIAN_POINT('Origin',(-85.59,44.5787611019615,-74.4494897427832));
#53269=CARTESIAN_POINT('Origin',(-48.39,-0.8,-66.39));
#53270=CARTESIAN_POINT('',(-48.39,-0.8,-67.64));
#53271=CARTESIAN_POINT('Origin',(-48.39,-0.8,-66.39));
#53272=CARTESIAN_POINT('',(-48.39,1.38777878078145E-16,-67.64));
#53273=CARTESIAN_POINT('',(-48.39,-0.8,-67.64));
#53274=CARTESIAN_POINT('Origin',(-48.39,1.0842021724855E-16,-66.39));
#53275=CARTESIAN_POINT('Origin',(-48.39,-0.8,67.61));
#53276=CARTESIAN_POINT('',(-48.39,-0.8,66.36));
#53277=CARTESIAN_POINT('Origin',(-48.39,-0.8,67.61));
#53278=CARTESIAN_POINT('',(-48.39,1.38777878078145E-16,66.36));
#53279=CARTESIAN_POINT('',(-48.39,-0.8,66.36));
#53280=CARTESIAN_POINT('Origin',(-48.39,1.0842021724855E-16,67.61));
#53281=CARTESIAN_POINT('Origin',(61.61,-0.8,67.61));
#53282=CARTESIAN_POINT('',(61.61,-0.8,66.36));
#53283=CARTESIAN_POINT('Origin',(61.61,-0.8,67.61));
#53284=CARTESIAN_POINT('',(61.61,1.38777878078145E-16,66.36));
#53285=CARTESIAN_POINT('',(61.61,-0.8,66.36));
#53286=CARTESIAN_POINT('Origin',(61.61,1.0842021724855E-16,67.61));
#53287=CARTESIAN_POINT('Origin',(61.61,-0.8,-66.39));
#53288=CARTESIAN_POINT('',(61.61,-0.8,-67.64));
#53289=CARTESIAN_POINT('Origin',(61.61,-0.8,-66.39));
#53290=CARTESIAN_POINT('',(61.61,1.38777878078145E-16,-67.64));
#53291=CARTESIAN_POINT('',(61.61,-0.8,-67.64));
#53292=CARTESIAN_POINT('Origin',(61.61,1.0842021724855E-16,-66.39));
#53293=CARTESIAN_POINT('Ctrl Pts',(-85.5899999999997,44.5787611019615,10.));
#53294=CARTESIAN_POINT('Ctrl Pts',(-86.5500000000002,44.5787611019615,10.));
#53295=CARTESIAN_POINT('Ctrl Pts',(-85.5899999999997,45.8877414717319,9.99999275845459));
#53296=CARTESIAN_POINT('Ctrl Pts',(-86.5500000000002,45.8877414717319,9.99999275845459));
#53297=CARTESIAN_POINT('Ctrl Pts',(-85.5899999999995,48.505792262655,9.872293593712));
#53298=CARTESIAN_POINT('Ctrl Pts',(-86.55,48.505792262655,9.872293593712));
#53299=CARTESIAN_POINT('Ctrl Pts',(-85.5899999999998,52.3946948078235,9.29405950036845));
#53300=CARTESIAN_POINT('Ctrl Pts',(-86.5500000000003,52.3946948078235,9.29405950036845));
#53301=CARTESIAN_POINT('Ctrl Pts',(-85.5899999999998,56.2089960261238,8.34006566164691));
#53302=CARTESIAN_POINT('Ctrl Pts',(-86.5500000000003,56.2089960261238,8.34006566164691));
#53303=CARTESIAN_POINT('Ctrl Pts',(-85.5899999999998,59.3413461461202,7.21805787048124));
#53304=CARTESIAN_POINT('Ctrl Pts',(-86.5500000000003,59.3413461461202,7.21805787048124));
#53305=CARTESIAN_POINT('Ctrl Pts',(-85.5899999999999,61.1821105626304,6.39829807210438));
#53306=CARTESIAN_POINT('Ctrl Pts',(-86.5500000000004,61.1821105626304,6.39829807210438));
#53307=CARTESIAN_POINT('Ctrl Pts',(-85.5899999999999,61.8185255808726,6.09446728275319));
#53308=CARTESIAN_POINT('Ctrl Pts',(-86.5500000000004,61.8185255808726,6.09446728275319));
#53309=CARTESIAN_POINT('',(-85.59,61.8185255808636,6.09446728275746));
#53310=CARTESIAN_POINT('',(-85.5899999999999,44.5787611019615,10.));
#53311=CARTESIAN_POINT('Ctrl Pts',(-85.5899999999999,61.8185255808636,6.09446728275746));
#53312=CARTESIAN_POINT('Ctrl Pts',(-85.5899999999999,61.1821105626304,6.39829807210438));
#53313=CARTESIAN_POINT('Ctrl Pts',(-85.5899999999998,59.3413461461202,7.21805787048124));
#53314=CARTESIAN_POINT('Ctrl Pts',(-85.5899999999998,56.2089960261238,8.34006566164691));
#53315=CARTESIAN_POINT('Ctrl Pts',(-85.5899999999998,52.3946948078235,9.29405950036845));
#53316=CARTESIAN_POINT('Ctrl Pts',(-85.5899999999995,48.505792262655,9.872293593712));
#53317=CARTESIAN_POINT('Ctrl Pts',(-85.5899999999997,45.8877414717319,9.99999275845459));
#53318=CARTESIAN_POINT('Ctrl Pts',(-85.5899999999997,44.5787611019615,10.));
#53319=CARTESIAN_POINT('',(-86.3899999999999,44.5787611019615,10.));
#53320=CARTESIAN_POINT('',(903.61,44.578761101962,10.));
#53321=CARTESIAN_POINT('',(-86.39,61.8185255808636,6.09446728275746));
#53322=CARTESIAN_POINT('Ctrl Pts',(-86.39,61.8185255808636,6.09446728275747));
#53323=CARTESIAN_POINT('Ctrl Pts',(-86.39,61.1821105626304,6.39829807210438));
#53324=CARTESIAN_POINT('Ctrl Pts',(-86.39,59.3413461461202,7.21805787048124));
#53325=CARTESIAN_POINT('Ctrl Pts',(-86.39,56.2089960261238,8.34006566164691));
#53326=CARTESIAN_POINT('Ctrl Pts',(-86.39,52.3946948078235,9.29405950036845));
#53327=CARTESIAN_POINT('Ctrl Pts',(-86.3899999999996,48.505792262655,9.872293593712));
#53328=CARTESIAN_POINT('Ctrl Pts',(-86.3899999999998,45.8877414717319,9.99999275845459));
#53329=CARTESIAN_POINT('Ctrl Pts',(-86.3899999999998,44.5787611019615,10.));
#53330=CARTESIAN_POINT('',(-86.39,61.8185255808636,6.09446728275746));
#53331=CARTESIAN_POINT('Origin',(-84.39,-3.2,80.));
#53332=CARTESIAN_POINT('',(-67.3504246383764,-3.20000000000001,-80.));
#53333=CARTESIAN_POINT('',(-67.3504246383764,-3.20000000000001,-78.16));
#53334=CARTESIAN_POINT('',(-67.3504246383764,-3.20000000000001,-80.));
#53335=CARTESIAN_POINT('',(-82.2324777960769,-3.2,-80.));
#53336=CARTESIAN_POINT('',(-84.39,-3.2,-80.));
#53337=CARTESIAN_POINT('',(-82.2324777960769,-3.2,-70.));
#53338=CARTESIAN_POINT('',(-82.2324777960769,-3.2,-70.));
#53339=CARTESIAN_POINT('',(-82.79,-3.2,-68.8330657242578));
#53340=CARTESIAN_POINT('Origin',(-83.7324777960769,-3.2,-70.));
#53341=CARTESIAN_POINT('',(-82.79,-3.2,68.8330657242578));
#53342=CARTESIAN_POINT('',(-82.79,-3.2,80.));
#53343=CARTESIAN_POINT('',(-82.2324777960769,-3.2,70.));
#53344=CARTESIAN_POINT('Origin',(-83.7324777960769,-3.2,70.));
#53345=CARTESIAN_POINT('',(-82.2324777960769,-3.2,80.));
#53346=CARTESIAN_POINT('',(-82.2324777960769,-3.2,70.));
#53347=CARTESIAN_POINT('',(-67.3504246383764,-3.2,80.));
#53348=CARTESIAN_POINT('',(-84.39,-3.2,80.));
#53349=CARTESIAN_POINT('',(-67.3504246383764,-3.19999999999999,78.16));
#53350=CARTESIAN_POINT('',(-67.3504246383764,-3.19999999999999,78.16));
#53351=CARTESIAN_POINT('',(-67.1104246383764,-3.19999999999999,78.16));
#53352=CARTESIAN_POINT('',(-67.1104246383764,-3.19999999999999,78.16));
#53353=CARTESIAN_POINT('',(-67.1104246383764,-3.19999999999999,78.4));
#53354=CARTESIAN_POINT('',(-67.1104246383764,-3.19999999999999,78.4));
#53355=CARTESIAN_POINT('',(52.8895753616236,-3.19999999999999,78.4));
#53356=CARTESIAN_POINT('',(52.8895753616236,-3.19999999999999,78.4));
#53357=CARTESIAN_POINT('',(52.8895753616236,-3.19999999999999,78.16));
#53358=CARTESIAN_POINT('',(52.8895753616236,-3.19999999999999,78.16));
#53359=CARTESIAN_POINT('',(53.1295753616236,-3.19999999999999,78.16));
#53360=CARTESIAN_POINT('',(53.1295753616236,-3.19999999999999,78.16));
#53361=CARTESIAN_POINT('',(53.1295753616236,-3.2,80.));
#53362=CARTESIAN_POINT('',(53.1295753616236,-3.2,80.));
#53363=CARTESIAN_POINT('',(68.4524777960769,-3.2,80.));
#53364=CARTESIAN_POINT('',(-84.39,-3.2,80.));
#53365=CARTESIAN_POINT('',(68.4524777960769,-3.2,70.));
#53366=CARTESIAN_POINT('',(68.4524777960769,-3.2,70.));
#53367=CARTESIAN_POINT('',(69.01,-3.2,68.8330657242578));
#53368=CARTESIAN_POINT('Origin',(69.9524777960769,-3.2,70.));
#53369=CARTESIAN_POINT('',(69.01,-3.2,-68.8330657242578));
#53370=CARTESIAN_POINT('',(69.01,-3.2,80.));
#53371=CARTESIAN_POINT('',(68.4524777960769,-3.2,-70.));
#53372=CARTESIAN_POINT('Origin',(69.9524777960769,-3.2,-70.));
#53373=CARTESIAN_POINT('',(68.4524777960769,-3.2,-80.));
#53374=CARTESIAN_POINT('',(68.4524777960769,-3.2,-70.));
#53375=CARTESIAN_POINT('',(53.1295753616236,-3.2,-80.));
#53376=CARTESIAN_POINT('',(-84.39,-3.2,-80.));
#53377=CARTESIAN_POINT('',(53.1295753616236,-3.20000000000001,-78.16));
#53378=CARTESIAN_POINT('',(53.1295753616236,-3.20000000000001,-78.16));
#53379=CARTESIAN_POINT('',(52.8895753616236,-3.20000000000001,-78.16));
#53380=CARTESIAN_POINT('',(52.8895753616236,-3.20000000000001,-78.16));
#53381=CARTESIAN_POINT('',(52.8895753616236,-3.20000000000001,-78.4));
#53382=CARTESIAN_POINT('',(52.8895753616236,-3.20000000000001,-78.4));
#53383=CARTESIAN_POINT('',(-67.1104246383764,-3.20000000000001,-78.4));
#53384=CARTESIAN_POINT('',(-67.1104246383764,-3.20000000000001,-78.4));
#53385=CARTESIAN_POINT('',(-67.1104246383764,-3.20000000000001,-78.16));
#53386=CARTESIAN_POINT('',(-67.1104246383764,-3.20000000000001,-78.16));
#53387=CARTESIAN_POINT('',(-67.3504246383764,-3.20000000000001,-78.16));
#53388=CARTESIAN_POINT('',(-44.7186753691159,-3.2,69.61));
#53389=CARTESIAN_POINT('',(-43.1186753691159,-3.2,69.61));
#53390=CARTESIAN_POINT('',(-84.39,-3.2,69.61));
#53391=CARTESIAN_POINT('',(-52.061324630884,-3.2,69.61));
#53392=CARTESIAN_POINT('',(-84.39,-3.2,69.61));
#53393=CARTESIAN_POINT('',(-53.661324630884,-3.2,69.61));
#53394=CARTESIAN_POINT('',(-84.39,-3.2,69.61));
#53395=CARTESIAN_POINT('',(-53.661324630884,-3.2,65.61));
#53396=CARTESIAN_POINT('',(-53.661324630884,-3.2,65.61));
#53397=CARTESIAN_POINT('',(-52.061324630884,-3.2,65.61));
#53398=CARTESIAN_POINT('',(-84.39,-3.2,65.61));
#53399=CARTESIAN_POINT('',(-44.7186753691159,-3.2,65.61));
#53400=CARTESIAN_POINT('',(-84.39,-3.2,65.61));
#53401=CARTESIAN_POINT('',(-43.1186753691159,-3.2,65.61));
#53402=CARTESIAN_POINT('',(-84.39,-3.2,65.61));
#53403=CARTESIAN_POINT('',(-43.1186753691159,-3.2,67.61));
#53404=CARTESIAN_POINT('',(65.2813246308841,-3.2,-64.39));
#53405=CARTESIAN_POINT('',(66.8813246308841,-3.2,-64.39));
#53406=CARTESIAN_POINT('',(-84.39,-3.2,-64.39));
#53407=CARTESIAN_POINT('',(57.938675369116,-3.2,-64.39));
#53408=CARTESIAN_POINT('',(-84.39,-3.2,-64.39));
#53409=CARTESIAN_POINT('',(56.338675369116,-3.2,-64.39));
#53410=CARTESIAN_POINT('',(-84.39,-3.2,-64.39));
#53411=CARTESIAN_POINT('',(56.338675369116,-3.2,-68.39));
#53412=CARTESIAN_POINT('',(56.338675369116,-3.2,-68.39));
#53413=CARTESIAN_POINT('',(57.938675369116,-3.2,-68.39));
#53414=CARTESIAN_POINT('',(-84.39,-3.2,-68.39));
#53415=CARTESIAN_POINT('',(65.2813246308841,-3.2,-68.39));
#53416=CARTESIAN_POINT('',(-84.39,-3.2,-68.39));
#53417=CARTESIAN_POINT('',(66.8813246308841,-3.2,-68.39));
#53418=CARTESIAN_POINT('',(-84.39,-3.2,-68.39));
#53419=CARTESIAN_POINT('',(66.8813246308841,-3.2,-66.39));
#53420=CARTESIAN_POINT('',(65.2813246308841,-3.2,69.61));
#53421=CARTESIAN_POINT('',(66.8813246308841,-3.2,69.61));
#53422=CARTESIAN_POINT('',(-84.39,-3.2,69.61));
#53423=CARTESIAN_POINT('',(57.938675369116,-3.2,69.61));
#53424=CARTESIAN_POINT('',(-84.39,-3.2,69.61));
#53425=CARTESIAN_POINT('',(56.338675369116,-3.2,69.61));
#53426=CARTESIAN_POINT('',(-84.39,-3.2,69.61));
#53427=CARTESIAN_POINT('',(56.338675369116,-3.2,65.61));
#53428=CARTESIAN_POINT('',(56.338675369116,-3.2,65.61));
#53429=CARTESIAN_POINT('',(57.938675369116,-3.2,65.61));
#53430=CARTESIAN_POINT('',(-84.39,-3.2,65.61));
#53431=CARTESIAN_POINT('',(65.2813246308841,-3.2,65.61));
#53432=CARTESIAN_POINT('',(-84.39,-3.2,65.61));
#53433=CARTESIAN_POINT('',(66.8813246308841,-3.2,65.61));
#53434=CARTESIAN_POINT('',(-84.39,-3.2,65.61));
#53435=CARTESIAN_POINT('',(66.8813246308841,-3.2,67.61));
#53436=CARTESIAN_POINT('',(-44.7186753691159,-3.2,-64.39));
#53437=CARTESIAN_POINT('',(-43.1186753691159,-3.2,-64.39));
#53438=CARTESIAN_POINT('',(-84.39,-3.2,-64.39));
#53439=CARTESIAN_POINT('',(-52.061324630884,-3.2,-64.39));
#53440=CARTESIAN_POINT('',(-84.39,-3.2,-64.39));
#53441=CARTESIAN_POINT('',(-53.661324630884,-3.2,-64.39));
#53442=CARTESIAN_POINT('',(-84.39,-3.2,-64.39));
#53443=CARTESIAN_POINT('',(-53.661324630884,-3.2,-68.39));
#53444=CARTESIAN_POINT('',(-53.661324630884,-3.2,-68.39));
#53445=CARTESIAN_POINT('',(-52.061324630884,-3.2,-68.39));
#53446=CARTESIAN_POINT('',(-84.39,-3.2,-68.39));
#53447=CARTESIAN_POINT('',(-44.7186753691159,-3.2,-68.39));
#53448=CARTESIAN_POINT('',(-84.39,-3.2,-68.39));
#53449=CARTESIAN_POINT('',(-43.1186753691159,-3.2,-68.39));
#53450=CARTESIAN_POINT('',(-84.39,-3.2,-68.39));
#53451=CARTESIAN_POINT('',(-43.1186753691159,-3.2,-66.39));
#53452=CARTESIAN_POINT('Origin',(-84.39,-4.,80.));
#53453=CARTESIAN_POINT('',(-67.3504246383764,-4.,-80.));
#53454=CARTESIAN_POINT('',(-82.2324777960769,-4.,-80.));
#53455=CARTESIAN_POINT('',(-84.39,-4.,-80.));
#53456=CARTESIAN_POINT('',(-67.3504246383764,-4.,-78.16));
#53457=CARTESIAN_POINT('',(-67.3504246383764,-4.,80.));
#53458=CARTESIAN_POINT('',(-67.1104246383764,-4.,-78.16));
#53459=CARTESIAN_POINT('',(-84.39,-4.,-78.16));
#53460=CARTESIAN_POINT('',(-67.1104246383764,-4.00000000000001,-78.4));
#53461=CARTESIAN_POINT('',(-67.1104246383764,-4.,80.));
#53462=CARTESIAN_POINT('',(52.8895753616236,-4.,-78.4));
#53463=CARTESIAN_POINT('',(-67.1104246383764,-4.00000000000001,-78.4));
#53464=CARTESIAN_POINT('',(52.8895753616236,-4.,-78.16));
#53465=CARTESIAN_POINT('',(52.8895753616236,-4.,80.));
#53466=CARTESIAN_POINT('',(53.1295753616236,-4.,-78.16));
#53467=CARTESIAN_POINT('',(-84.39,-4.,-78.16));
#53468=CARTESIAN_POINT('',(53.1295753616236,-4.,-80.));
#53469=CARTESIAN_POINT('',(53.1295753616241,-4.,79.9999999999995));
#53470=CARTESIAN_POINT('',(68.4524777960769,-4.,-80.));
#53471=CARTESIAN_POINT('',(-84.39,-4.,-80.));
#53472=CARTESIAN_POINT('',(68.4524777960769,-4.,-70.));
#53473=CARTESIAN_POINT('',(68.4524777960769,-4.,80.));
#53474=CARTESIAN_POINT('',(69.01,-4.,-68.8330657242578));
#53475=CARTESIAN_POINT('Origin',(69.9524777960769,-4.,-70.));
#53476=CARTESIAN_POINT('',(69.01,-4.,68.8330657242578));
#53477=CARTESIAN_POINT('',(69.01,-4.,80.));
#53478=CARTESIAN_POINT('',(68.4524777960769,-4.,70.));
#53479=CARTESIAN_POINT('Origin',(69.9524777960769,-4.,70.));
#53480=CARTESIAN_POINT('',(68.4524777960769,-4.,80.));
#53481=CARTESIAN_POINT('',(68.4524777960769,-4.,80.));
#53482=CARTESIAN_POINT('',(53.1295753616236,-4.,80.));
#53483=CARTESIAN_POINT('',(-84.39,-4.,80.));
#53484=CARTESIAN_POINT('',(53.1295753616236,-4.,78.16));
#53485=CARTESIAN_POINT('',(53.1295753616236,-4.,80.0000000000005));
#53486=CARTESIAN_POINT('',(52.8895753616236,-4.,78.16));
#53487=CARTESIAN_POINT('',(-84.39,-4.,78.16));
#53488=CARTESIAN_POINT('',(52.8895753616236,-3.99999999999999,78.4));
#53489=CARTESIAN_POINT('',(52.8895753616236,-4.,80.));
#53490=CARTESIAN_POINT('',(-67.1104246383764,-4.,78.4));
#53491=CARTESIAN_POINT('',(52.8895753616236,-3.99999999999999,78.4));
#53492=CARTESIAN_POINT('',(-67.1104246383764,-4.,78.16));
#53493=CARTESIAN_POINT('',(-67.1104246383764,-4.,80.));
#53494=CARTESIAN_POINT('',(-67.3504246383764,-4.,78.16));
#53495=CARTESIAN_POINT('',(-84.39,-4.,78.16));
#53496=CARTESIAN_POINT('',(-67.3504246383764,-4.,80.));
#53497=CARTESIAN_POINT('',(-67.3504246383764,-4.,80.));
#53498=CARTESIAN_POINT('',(-82.2324777960769,-4.,80.));
#53499=CARTESIAN_POINT('',(-84.39,-4.,80.));
#53500=CARTESIAN_POINT('',(-82.2324777960769,-4.,70.));
#53501=CARTESIAN_POINT('',(-82.2324777960769,-4.,80.));
#53502=CARTESIAN_POINT('',(-82.79,-4.,68.8330657242578));
#53503=CARTESIAN_POINT('Origin',(-83.7324777960769,-4.,70.));
#53504=CARTESIAN_POINT('',(-82.79,-4.,-68.8330657242578));
#53505=CARTESIAN_POINT('',(-82.79,-4.,80.));
#53506=CARTESIAN_POINT('',(-82.2324777960769,-4.,-70.));
#53507=CARTESIAN_POINT('Origin',(-83.7324777960769,-4.,-70.));
#53508=CARTESIAN_POINT('',(-82.2324777960769,-4.,80.));
#53509=CARTESIAN_POINT('',(56.338675369116,-4.,-68.39));
#53510=CARTESIAN_POINT('',(66.8813246308841,-4.,-68.39));
#53511=CARTESIAN_POINT('',(57.61,-4.,-68.39));
#53512=CARTESIAN_POINT('',(56.338675369116,-4.,-64.39));
#53513=CARTESIAN_POINT('',(56.338675369116,-4.,-66.39));
#53514=CARTESIAN_POINT('',(66.8813246308841,-4.,-64.39));
#53515=CARTESIAN_POINT('',(57.61,-4.,-64.39));
#53516=CARTESIAN_POINT('',(66.8813246308841,-4.,-66.39));
#53517=CARTESIAN_POINT('',(56.338675369116,-4.,65.61));
#53518=CARTESIAN_POINT('',(66.8813246308841,-4.,65.61));
#53519=CARTESIAN_POINT('',(57.61,-4.,65.61));
#53520=CARTESIAN_POINT('',(56.338675369116,-4.,69.61));
#53521=CARTESIAN_POINT('',(56.338675369116,-4.,67.61));
#53522=CARTESIAN_POINT('',(66.8813246308841,-4.,69.61));
#53523=CARTESIAN_POINT('',(57.61,-4.,69.61));
#53524=CARTESIAN_POINT('',(66.8813246308841,-4.,67.61));
#53525=CARTESIAN_POINT('',(-53.661324630884,-4.,65.61));
#53526=CARTESIAN_POINT('',(-43.1186753691159,-4.,65.61));
#53527=CARTESIAN_POINT('',(-52.39,-4.,65.61));
#53528=CARTESIAN_POINT('',(-53.661324630884,-4.,69.61));
#53529=CARTESIAN_POINT('',(-53.661324630884,-4.,67.61));
#53530=CARTESIAN_POINT('',(-43.1186753691159,-4.,69.61));
#53531=CARTESIAN_POINT('',(-52.39,-4.,69.61));
#53532=CARTESIAN_POINT('',(-43.1186753691159,-4.,67.61));
#53533=CARTESIAN_POINT('',(-53.661324630884,-4.,-68.39));
#53534=CARTESIAN_POINT('',(-43.1186753691159,-4.,-68.39));
#53535=CARTESIAN_POINT('',(-52.39,-4.,-68.39));
#53536=CARTESIAN_POINT('',(-53.661324630884,-4.,-64.39));
#53537=CARTESIAN_POINT('',(-53.661324630884,-4.,-66.39));
#53538=CARTESIAN_POINT('',(-43.1186753691159,-4.,-64.39));
#53539=CARTESIAN_POINT('',(-52.39,-4.,-64.39));
#53540=CARTESIAN_POINT('',(-43.1186753691159,-4.,-66.39));
#53541=CARTESIAN_POINT('Origin',(-83.59,-2.4,-80.));
#53542=CARTESIAN_POINT('',(-67.3504246383764,-3.20000000000001,-80.));
#53543=CARTESIAN_POINT('',(-82.2324777960769,-2.4,-80.));
#53544=CARTESIAN_POINT('Origin',(-83.59,-2.4,-80.));
#53545=CARTESIAN_POINT('',(53.1295753616236,-3.20000000000001,-80.));
#53546=CARTESIAN_POINT('',(68.4524777960769,-2.4,-80.));
#53547=CARTESIAN_POINT('Origin',(-63.1104246383764,2.79999999999999,79.2));
#53548=CARTESIAN_POINT('',(52.8895753616236,-2.4,79.2));
#53549=CARTESIAN_POINT('',(52.8895753616236,2.80000000000002,79.2));
#53550=CARTESIAN_POINT('',(52.8895753616236,2.80000000000001,79.2));
#53551=CARTESIAN_POINT('',(-67.1104246383764,-2.4,79.2));
#53552=CARTESIAN_POINT('',(-67.1104246383764,-2.4,79.2));
#53553=CARTESIAN_POINT('',(-67.1104246383764,2.79999999999997,79.2));
#53554=CARTESIAN_POINT('',(-67.1104246383764,-3.2,79.2));
#53555=CARTESIAN_POINT('',(-63.1104246383764,6.79999999999999,79.2));
#53556=CARTESIAN_POINT('Origin',(-63.1104246383764,2.79999999999999,79.2));
#53557=CARTESIAN_POINT('',(48.8895753616235,6.80000000000003,79.2));
#53558=CARTESIAN_POINT('',(-63.1104246383764,6.79999999999999,79.2));
#53559=CARTESIAN_POINT('Origin',(48.8895753616236,2.80000000000003,79.2));
#53560=CARTESIAN_POINT('',(-57.3817492692605,3.80000000000003,79.1999999999841));
#53561=CARTESIAN_POINT('',(-57.3817492692605,-0.199999999999971,79.199999999992));
#53562=CARTESIAN_POINT('',(-57.3817492692605,1.80000000000003,79.1999999999841));
#53563=CARTESIAN_POINT('',(-55.7817492692724,-0.199999999999971,79.2));
#53564=CARTESIAN_POINT('',(-63.1104246383764,-0.199999999999971,79.2));
#53565=CARTESIAN_POINT('',(-48.4391000074804,-0.199999999999971,79.2));
#53566=CARTESIAN_POINT('',(-63.1104246383764,-0.199999999999972,79.2));
#53567=CARTESIAN_POINT('',(-46.8391000074924,-0.199999999999969,79.1999999999841));
#53568=CARTESIAN_POINT('',(-63.1104246383764,-0.199999999999971,79.2));
#53569=CARTESIAN_POINT('',(-46.8391000074924,3.80000000000003,79.199999999992));
#53570=CARTESIAN_POINT('',(-46.8391000074924,3.80000000000003,79.1999999999841));
#53571=CARTESIAN_POINT('',(-48.4391000074804,3.80000000000003,79.2));
#53572=CARTESIAN_POINT('',(-63.1104246383764,3.80000000000003,79.2));
#53573=CARTESIAN_POINT('',(-55.7817492692724,3.80000000000003,79.2));
#53574=CARTESIAN_POINT('',(-63.1104246383764,3.80000000000003,79.2));
#53575=CARTESIAN_POINT('',(-63.1104246383764,3.80000000000003,79.2));
#53576=CARTESIAN_POINT('',(33.0591000074924,-0.199999999999946,79.199999999992));
#53577=CARTESIAN_POINT('',(33.0591000074924,3.80000000000005,79.1999999999841));
#53578=CARTESIAN_POINT('',(33.0591000074924,3.80000000000005,79.1999999999841));
#53579=CARTESIAN_POINT('',(34.6591000074805,-0.199999999999947,79.2));
#53580=CARTESIAN_POINT('',(-63.1104246383764,-0.200000000000004,79.2));
#53581=CARTESIAN_POINT('',(42.0017492692724,-0.199999999999943,79.2));
#53582=CARTESIAN_POINT('',(-63.1104246383764,-0.200000000000005,79.2));
#53583=CARTESIAN_POINT('',(43.6017492692605,-0.19999999999994,79.1999999999841));
#53584=CARTESIAN_POINT('',(-63.1104246383764,-0.200000000000004,79.2));
#53585=CARTESIAN_POINT('',(43.6017492692605,3.80000000000006,79.199999999992));
#53586=CARTESIAN_POINT('',(43.6017492692605,1.80000000000006,79.1999999999841));
#53587=CARTESIAN_POINT('',(42.0017492692724,3.80000000000006,79.2));
#53588=CARTESIAN_POINT('',(-63.1104246383764,3.8,79.2));
#53589=CARTESIAN_POINT('',(34.6591000074805,3.80000000000005,79.2));
#53590=CARTESIAN_POINT('',(-63.1104246383764,3.8,79.2));
#53591=CARTESIAN_POINT('',(-63.1104246383764,3.8,79.2));
#53592=CARTESIAN_POINT('Origin',(-63.1104246383764,2.79999999999999,80.));
#53593=CARTESIAN_POINT('',(52.8895753616236,-2.4,80.));
#53594=CARTESIAN_POINT('',(-67.1104246383764,-2.4,80.));
#53595=CARTESIAN_POINT('',(-67.1104246383764,-2.4,80.));
#53596=CARTESIAN_POINT('',(52.8895753616236,2.80000000000002,80.));
#53597=CARTESIAN_POINT('',(52.8895753616236,2.80000000000012,80.));
#53598=CARTESIAN_POINT('',(48.8895753616235,6.80000000000003,80.));
#53599=CARTESIAN_POINT('Origin',(48.8895753616236,2.80000000000003,80.));
#53600=CARTESIAN_POINT('',(-63.1104246383764,6.79999999999999,80.));
#53601=CARTESIAN_POINT('',(-63.1104246383764,6.79999999999999,80.));
#53602=CARTESIAN_POINT('',(-67.1104246383764,2.79999999999997,80.));
#53603=CARTESIAN_POINT('Origin',(-63.1104246383764,2.79999999999999,80.));
#53604=CARTESIAN_POINT('',(-67.1104246383764,2.79999999999999,80.));
#53605=CARTESIAN_POINT('',(-46.8391000074924,3.80000000000003,79.9999999999841));
#53606=CARTESIAN_POINT('',(-57.3817492692605,3.80000000000003,79.999999999992));
#53607=CARTESIAN_POINT('',(-48.1104246383764,3.80000000000003,79.9999999999841));
#53608=CARTESIAN_POINT('',(-46.8391000074924,-0.199999999999972,79.9999999999841));
#53609=CARTESIAN_POINT('',(-46.8391000074924,1.80000000000003,79.9999999999841));
#53610=CARTESIAN_POINT('',(-57.3817492692605,-0.199999999999971,79.9999999999841));
#53611=CARTESIAN_POINT('',(-48.1104246383764,-0.199999999999972,79.9999999999841));
#53612=CARTESIAN_POINT('',(-57.3817492692605,1.80000000000003,79.9999999999841));
#53613=CARTESIAN_POINT('',(33.0591000074924,-0.199999999999949,79.9999999999841));
#53614=CARTESIAN_POINT('',(33.0591000074924,3.80000000000005,79.9999999999841));
#53615=CARTESIAN_POINT('',(33.0591000074924,1.80000000000005,79.9999999999841));
#53616=CARTESIAN_POINT('',(43.6017492692605,3.80000000000006,79.9999999999841));
#53617=CARTESIAN_POINT('',(34.3304246383764,3.80000000000005,79.9999999999841));
#53618=CARTESIAN_POINT('',(43.6017492692605,-0.199999999999941,79.999999999992));
#53619=CARTESIAN_POINT('',(43.6017492692605,1.80000000000006,79.9999999999841));
#53620=CARTESIAN_POINT('',(34.3304246383764,-0.199999999999948,79.9999999999841));
#53621=CARTESIAN_POINT('Origin',(69.81,-2.4,80.));
#53622=CARTESIAN_POINT('',(53.1295753616236,-3.2,80.));
#53623=CARTESIAN_POINT('',(68.4524777960769,-2.4,80.));
#53624=CARTESIAN_POINT('Origin',(69.81,-2.4,80.));
#53625=CARTESIAN_POINT('',(-67.3504246383764,-3.2,80.));
#53626=CARTESIAN_POINT('',(-82.2324777960769,-2.4,80.));
#53627=CARTESIAN_POINT('Origin',(70.61,91.,80.));
#53628=CARTESIAN_POINT('',(70.61,86.,-80.));
#53629=CARTESIAN_POINT('',(70.6100000000008,-1.84247779607696,-80.));
#53630=CARTESIAN_POINT('',(70.61,91.,-80.));
#53631=CARTESIAN_POINT('',(70.61,91.,-75.));
#53632=CARTESIAN_POINT('',(70.61,168.5,2.50000000000003));
#53633=CARTESIAN_POINT('',(70.61,91.,75.));
#53634=CARTESIAN_POINT('',(70.61,91.,80.));
#53635=CARTESIAN_POINT('',(70.61,86.,80.));
#53636=CARTESIAN_POINT('',(70.61,88.5,77.5));
#53637=CARTESIAN_POINT('',(70.61,-1.84247779607696,80.));
#53638=CARTESIAN_POINT('',(70.61,91.,80.));
#53639=CARTESIAN_POINT('',(70.61,-1.84247779607696,70.));
#53640=CARTESIAN_POINT('',(70.61,-1.84247779607696,80.));
#53641=CARTESIAN_POINT('',(70.61,-2.4,68.8330657242578));
#53642=CARTESIAN_POINT('Origin',(70.61,-3.34247779607697,70.));
#53643=CARTESIAN_POINT('',(70.61,-2.4,-68.8330657242578));
#53644=CARTESIAN_POINT('',(70.61,-2.4,80.));
#53645=CARTESIAN_POINT('',(70.61,-1.84247779607696,-70.));
#53646=CARTESIAN_POINT('Origin',(70.61,-3.34247779607697,-70.));
#53647=CARTESIAN_POINT('',(70.61,-1.84247779607696,80.));
#53648=CARTESIAN_POINT('',(70.61,46.0787611019615,-66.5));
#53649=CARTESIAN_POINT('',(70.61,1.35867816760341E-14,-66.5));
#53650=CARTESIAN_POINT('',(70.61,46.0787611019615,-69.5));
#53651=CARTESIAN_POINT('',(70.61,1.35867816760341E-14,-69.5));
#53652=CARTESIAN_POINT('Origin',(70.61,46.0787611019615,-68.));
#53653=CARTESIAN_POINT('',(70.61,46.0787611019615,-21.5));
#53654=CARTESIAN_POINT('',(70.61,1.35867816760341E-14,-21.5));
#53655=CARTESIAN_POINT('',(70.61,46.0787611019615,-24.5));
#53656=CARTESIAN_POINT('',(70.61,1.35867816760341E-14,-24.5));
#53657=CARTESIAN_POINT('Origin',(70.61,46.0787611019615,-23.));
#53658=CARTESIAN_POINT('',(70.61,46.0787611019615,-16.5));
#53659=CARTESIAN_POINT('',(70.61,1.35867816760341E-14,-16.5));
#53660=CARTESIAN_POINT('',(70.61,46.0787611019615,-19.5));
#53661=CARTESIAN_POINT('',(70.61,1.35867816760341E-14,-19.5));
#53662=CARTESIAN_POINT('Origin',(70.61,46.0787611019615,-18.));
#53663=CARTESIAN_POINT('',(70.61,46.0787611019615,-11.5));
#53664=CARTESIAN_POINT('',(70.61,1.35867816760341E-14,-11.5));
#53665=CARTESIAN_POINT('',(70.61,46.0787611019615,-14.5));
#53666=CARTESIAN_POINT('',(70.61,1.35867816760341E-14,-14.5));
#53667=CARTESIAN_POINT('Origin',(70.61,46.0787611019615,-13.));
#53668=CARTESIAN_POINT('',(70.61,46.0787611019615,-41.5));
#53669=CARTESIAN_POINT('',(70.61,1.35867816760341E-14,-41.5));
#53670=CARTESIAN_POINT('',(70.61,46.0787611019615,-44.5));
#53671=CARTESIAN_POINT('',(70.61,1.35867816760341E-14,-44.5));
#53672=CARTESIAN_POINT('Origin',(70.61,46.0787611019615,-43.));
#53673=CARTESIAN_POINT('',(70.61,46.0787611019615,-46.5));
#53674=CARTESIAN_POINT('',(70.61,1.35867816760341E-14,-46.5));
#53675=CARTESIAN_POINT('',(70.61,46.0787611019615,-49.5));
#53676=CARTESIAN_POINT('',(70.61,1.35867816760341E-14,-49.5));
#53677=CARTESIAN_POINT('Origin',(70.61,46.0787611019615,-48.));
#53678=CARTESIAN_POINT('',(70.61,46.0787611019615,-51.5));
#53679=CARTESIAN_POINT('',(70.61,1.35867816760341E-14,-51.5));
#53680=CARTESIAN_POINT('',(70.61,46.0787611019615,-54.5));
#53681=CARTESIAN_POINT('',(70.61,1.35867816760341E-14,-54.5));
#53682=CARTESIAN_POINT('Origin',(70.61,46.0787611019615,-53.));
#53683=CARTESIAN_POINT('',(70.61,46.0787611019615,-56.5));
#53684=CARTESIAN_POINT('',(70.61,1.35867816760341E-14,-56.5));
#53685=CARTESIAN_POINT('',(70.61,46.0787611019615,-59.5));
#53686=CARTESIAN_POINT('',(70.61,1.35867816760341E-14,-59.5));
#53687=CARTESIAN_POINT('Origin',(70.61,46.0787611019615,-58.));
#53688=CARTESIAN_POINT('',(70.61,46.0787611019615,-61.5));
#53689=CARTESIAN_POINT('',(70.61,1.35867816760341E-14,-61.5));
#53690=CARTESIAN_POINT('',(70.61,46.0787611019615,-64.5));
#53691=CARTESIAN_POINT('',(70.61,1.35867816760341E-14,-64.5));
#53692=CARTESIAN_POINT('Origin',(70.61,46.0787611019615,-63.));
#53693=CARTESIAN_POINT('',(70.61,46.0787611019615,-26.5));
#53694=CARTESIAN_POINT('',(70.61,1.35867816760341E-14,-26.5));
#53695=CARTESIAN_POINT('',(70.61,46.0787611019615,-29.5));
#53696=CARTESIAN_POINT('',(70.61,1.35867816760341E-14,-29.5));
#53697=CARTESIAN_POINT('Origin',(70.61,46.0787611019615,-28.));
#53698=CARTESIAN_POINT('',(70.61,46.0787611019615,-31.5));
#53699=CARTESIAN_POINT('',(70.61,1.35867816760341E-14,-31.5));
#53700=CARTESIAN_POINT('',(70.61,46.0787611019615,-34.5));
#53701=CARTESIAN_POINT('',(70.61,1.35867816760341E-14,-34.5));
#53702=CARTESIAN_POINT('Origin',(70.61,46.0787611019615,-33.));
#53703=CARTESIAN_POINT('',(70.61,46.0787611019615,-36.5));
#53704=CARTESIAN_POINT('',(70.61,1.35867816760341E-14,-36.5));
#53705=CARTESIAN_POINT('',(70.61,46.0787611019615,-39.5));
#53706=CARTESIAN_POINT('',(70.61,1.35867816760341E-14,-39.5));
#53707=CARTESIAN_POINT('Origin',(70.61,46.0787611019615,-38.));
#53708=CARTESIAN_POINT('',(70.61,18.0787611019615,16.5));
#53709=CARTESIAN_POINT('',(70.61,1.35867816760341E-14,16.5));
#53710=CARTESIAN_POINT('',(70.61,18.0787611019615,19.5));
#53711=CARTESIAN_POINT('Origin',(70.61,18.0787611019615,18.));
#53712=CARTESIAN_POINT('',(70.61,1.35867816760341E-14,19.5));
#53713=CARTESIAN_POINT('',(70.61,18.0787611019615,21.5));
#53714=CARTESIAN_POINT('',(70.61,1.35867816760341E-14,21.5));
#53715=CARTESIAN_POINT('',(70.61,18.0787611019615,24.5));
#53716=CARTESIAN_POINT('Origin',(70.61,18.0787611019615,23.));
#53717=CARTESIAN_POINT('',(70.61,1.35867816760341E-14,24.5));
#53718=CARTESIAN_POINT('',(70.61,18.0787611019615,26.5));
#53719=CARTESIAN_POINT('',(70.61,1.35867816760341E-14,26.5));
#53720=CARTESIAN_POINT('',(70.61,18.0787611019615,29.5));
#53721=CARTESIAN_POINT('Origin',(70.61,18.0787611019615,28.));
#53722=CARTESIAN_POINT('',(70.61,1.35867816760341E-14,29.5));
#53723=CARTESIAN_POINT('',(70.61,18.0787611019615,11.5));
#53724=CARTESIAN_POINT('',(70.61,1.35867816760341E-14,11.5));
#53725=CARTESIAN_POINT('',(70.61,18.0787611019615,14.5));
#53726=CARTESIAN_POINT('Origin',(70.61,18.0787611019615,13.));
#53727=CARTESIAN_POINT('',(70.61,1.35867816760341E-14,14.5));
#53728=CARTESIAN_POINT('',(70.61,18.0787611019615,51.5));
#53729=CARTESIAN_POINT('',(70.61,1.35867816760341E-14,51.5));
#53730=CARTESIAN_POINT('',(70.61,18.0787611019615,54.5));
#53731=CARTESIAN_POINT('Origin',(70.61,18.0787611019615,53.));
#53732=CARTESIAN_POINT('',(70.61,1.35867816760341E-14,54.5));
#53733=CARTESIAN_POINT('',(70.61,18.0787611019615,46.5));
#53734=CARTESIAN_POINT('',(70.61,1.35867816760341E-14,46.5));
#53735=CARTESIAN_POINT('',(70.61,18.0787611019615,49.5));
#53736=CARTESIAN_POINT('Origin',(70.61,18.0787611019615,48.));
#53737=CARTESIAN_POINT('',(70.61,1.35867816760341E-14,49.5));
#53738=CARTESIAN_POINT('',(70.61,18.0787611019615,41.5));
#53739=CARTESIAN_POINT('',(70.61,1.35867816760341E-14,41.5));
#53740=CARTESIAN_POINT('',(70.61,18.0787611019615,44.5));
#53741=CARTESIAN_POINT('Origin',(70.61,18.0787611019615,43.));
#53742=CARTESIAN_POINT('',(70.61,1.35867816760341E-14,44.5));
#53743=CARTESIAN_POINT('',(70.61,18.0787611019615,31.5));
#53744=CARTESIAN_POINT('',(70.61,1.35867816760341E-14,31.5));
#53745=CARTESIAN_POINT('',(70.61,18.0787611019615,34.5));
#53746=CARTESIAN_POINT('Origin',(70.61,18.0787611019615,33.));
#53747=CARTESIAN_POINT('',(70.61,1.35867816760341E-14,34.5));
#53748=CARTESIAN_POINT('',(70.61,18.0787611019615,36.5));
#53749=CARTESIAN_POINT('',(70.61,1.35867816760341E-14,36.5));
#53750=CARTESIAN_POINT('',(70.61,18.0787611019615,39.5));
#53751=CARTESIAN_POINT('Origin',(70.61,18.0787611019615,38.));
#53752=CARTESIAN_POINT('',(70.61,1.35867816760341E-14,39.5));
#53753=CARTESIAN_POINT('',(70.61,18.0787611019615,56.5));
#53754=CARTESIAN_POINT('',(70.61,1.35867816760341E-14,56.5));
#53755=CARTESIAN_POINT('',(70.61,18.0787611019615,59.5));
#53756=CARTESIAN_POINT('Origin',(70.61,18.0787611019615,58.));
#53757=CARTESIAN_POINT('',(70.61,1.35867816760341E-14,59.5));
#53758=CARTESIAN_POINT('',(70.61,18.0787611019615,61.5));
#53759=CARTESIAN_POINT('',(70.61,1.35867816760341E-14,61.5));
#53760=CARTESIAN_POINT('',(70.61,18.0787611019615,64.5));
#53761=CARTESIAN_POINT('Origin',(70.61,18.0787611019615,63.));
#53762=CARTESIAN_POINT('',(70.61,1.35867816760341E-14,64.5));
#53763=CARTESIAN_POINT('',(70.61,18.0787611019615,66.5));
#53764=CARTESIAN_POINT('',(70.61,1.35867816760341E-14,66.5));
#53765=CARTESIAN_POINT('',(70.61,18.0787611019615,69.5));
#53766=CARTESIAN_POINT('Origin',(70.61,18.0787611019615,68.));
#53767=CARTESIAN_POINT('',(70.61,1.35867816760341E-14,69.5));
#53768=CARTESIAN_POINT('',(70.61,46.0787611019615,36.5));
#53769=CARTESIAN_POINT('',(70.61,1.35867816760341E-14,36.5));
#53770=CARTESIAN_POINT('',(70.61,46.0787611019615,39.5));
#53771=CARTESIAN_POINT('Origin',(70.61,46.0787611019615,38.));
#53772=CARTESIAN_POINT('',(70.61,1.35867816760341E-14,39.5));
#53773=CARTESIAN_POINT('',(70.61,46.0787611019615,31.5));
#53774=CARTESIAN_POINT('',(70.61,1.35867816760341E-14,31.5));
#53775=CARTESIAN_POINT('',(70.61,46.0787611019615,34.5));
#53776=CARTESIAN_POINT('Origin',(70.61,46.0787611019615,33.));
#53777=CARTESIAN_POINT('',(70.61,1.35867816760341E-14,34.5));
#53778=CARTESIAN_POINT('',(70.61,46.0787611019615,26.5));
#53779=CARTESIAN_POINT('',(70.61,1.35867816760341E-14,26.5));
#53780=CARTESIAN_POINT('',(70.61,46.0787611019615,29.5));
#53781=CARTESIAN_POINT('Origin',(70.61,46.0787611019615,28.));
#53782=CARTESIAN_POINT('',(70.61,1.35867816760341E-14,29.5));
#53783=CARTESIAN_POINT('',(70.61,46.0787611019615,61.5));
#53784=CARTESIAN_POINT('',(70.61,1.35867816760341E-14,61.5));
#53785=CARTESIAN_POINT('',(70.61,46.0787611019615,64.5));
#53786=CARTESIAN_POINT('Origin',(70.61,46.0787611019615,63.));
#53787=CARTESIAN_POINT('',(70.61,1.35867816760341E-14,64.5));
#53788=CARTESIAN_POINT('',(70.61,46.0787611019615,56.5));
#53789=CARTESIAN_POINT('',(70.61,1.35867816760341E-14,56.5));
#53790=CARTESIAN_POINT('',(70.61,46.0787611019615,59.5));
#53791=CARTESIAN_POINT('Origin',(70.61,46.0787611019615,58.));
#53792=CARTESIAN_POINT('',(70.61,1.35867816760341E-14,59.5));
#53793=CARTESIAN_POINT('',(70.61,46.0787611019615,51.5));
#53794=CARTESIAN_POINT('',(70.61,1.35867816760341E-14,51.5));
#53795=CARTESIAN_POINT('',(70.61,46.0787611019615,54.5));
#53796=CARTESIAN_POINT('Origin',(70.61,46.0787611019615,53.));
#53797=CARTESIAN_POINT('',(70.61,1.35867816760341E-14,54.5));
#53798=CARTESIAN_POINT('',(70.61,46.0787611019615,46.5));
#53799=CARTESIAN_POINT('',(70.61,1.35867816760341E-14,46.5));
#53800=CARTESIAN_POINT('',(70.61,46.0787611019615,49.5));
#53801=CARTESIAN_POINT('Origin',(70.61,46.0787611019615,48.));
#53802=CARTESIAN_POINT('',(70.61,1.35867816760341E-14,49.5));
#53803=CARTESIAN_POINT('',(70.61,46.0787611019615,41.5));
#53804=CARTESIAN_POINT('',(70.61,1.35867816760341E-14,41.5));
#53805=CARTESIAN_POINT('',(70.61,46.0787611019615,44.5));
#53806=CARTESIAN_POINT('Origin',(70.61,46.0787611019615,43.));
#53807=CARTESIAN_POINT('',(70.61,1.35867816760341E-14,44.5));
#53808=CARTESIAN_POINT('',(70.61,46.0787611019615,11.5));
#53809=CARTESIAN_POINT('',(70.61,1.35867816760341E-14,11.5));
#53810=CARTESIAN_POINT('',(70.61,46.0787611019615,14.5));
#53811=CARTESIAN_POINT('Origin',(70.61,46.0787611019615,13.));
#53812=CARTESIAN_POINT('',(70.61,1.35867816760341E-14,14.5));
#53813=CARTESIAN_POINT('',(70.61,46.0787611019615,16.5));
#53814=CARTESIAN_POINT('',(70.61,1.35867816760341E-14,16.5));
#53815=CARTESIAN_POINT('',(70.61,46.0787611019615,19.5));
#53816=CARTESIAN_POINT('Origin',(70.61,46.0787611019615,18.));
#53817=CARTESIAN_POINT('',(70.61,1.35867816760341E-14,19.5));
#53818=CARTESIAN_POINT('',(70.61,46.0787611019615,21.5));
#53819=CARTESIAN_POINT('',(70.61,1.35867816760341E-14,21.5));
#53820=CARTESIAN_POINT('',(70.61,46.0787611019615,24.5));
#53821=CARTESIAN_POINT('Origin',(70.61,46.0787611019615,23.));
#53822=CARTESIAN_POINT('',(70.61,1.35867816760341E-14,24.5));
#53823=CARTESIAN_POINT('',(70.61,46.0787611019615,66.5));
#53824=CARTESIAN_POINT('',(70.61,1.35867816760341E-14,66.5));
#53825=CARTESIAN_POINT('',(70.61,46.0787611019615,69.5));
#53826=CARTESIAN_POINT('Origin',(70.61,46.0787611019615,68.));
#53827=CARTESIAN_POINT('',(70.61,1.35867816760341E-14,69.5));
#53828=CARTESIAN_POINT('',(70.61,18.0787611019615,-66.5));
#53829=CARTESIAN_POINT('',(70.61,1.35867816760341E-14,-66.5));
#53830=CARTESIAN_POINT('',(70.61,18.0787611019615,-69.5));
#53831=CARTESIAN_POINT('',(70.61,1.35867816760341E-14,-69.5));
#53832=CARTESIAN_POINT('Origin',(70.61,18.0787611019615,-68.));
#53833=CARTESIAN_POINT('',(70.61,18.0787611019615,-61.5));
#53834=CARTESIAN_POINT('',(70.61,1.35867816760341E-14,-61.5));
#53835=CARTESIAN_POINT('',(70.61,18.0787611019615,-64.5));
#53836=CARTESIAN_POINT('',(70.61,1.35867816760341E-14,-64.5));
#53837=CARTESIAN_POINT('Origin',(70.61,18.0787611019615,-63.));
#53838=CARTESIAN_POINT('',(70.61,18.0787611019615,-56.5));
#53839=CARTESIAN_POINT('',(70.61,1.35867816760341E-14,-56.5));
#53840=CARTESIAN_POINT('',(70.61,18.0787611019615,-59.5));
#53841=CARTESIAN_POINT('',(70.61,1.35867816760341E-14,-59.5));
#53842=CARTESIAN_POINT('Origin',(70.61,18.0787611019615,-58.));
#53843=CARTESIAN_POINT('',(70.61,18.0787611019615,-36.5));
#53844=CARTESIAN_POINT('',(70.61,1.35867816760341E-14,-36.5));
#53845=CARTESIAN_POINT('',(70.61,18.0787611019615,-39.5));
#53846=CARTESIAN_POINT('',(70.61,1.35867816760341E-14,-39.5));
#53847=CARTESIAN_POINT('Origin',(70.61,18.0787611019615,-38.));
#53848=CARTESIAN_POINT('',(70.61,18.0787611019615,-31.5));
#53849=CARTESIAN_POINT('',(70.61,1.35867816760341E-14,-31.5));
#53850=CARTESIAN_POINT('',(70.61,18.0787611019615,-34.5));
#53851=CARTESIAN_POINT('',(70.61,1.35867816760341E-14,-34.5));
#53852=CARTESIAN_POINT('Origin',(70.61,18.0787611019615,-33.));
#53853=CARTESIAN_POINT('',(70.61,18.0787611019615,-41.5));
#53854=CARTESIAN_POINT('',(70.61,1.35867816760341E-14,-41.5));
#53855=CARTESIAN_POINT('',(70.61,18.0787611019615,-44.5));
#53856=CARTESIAN_POINT('',(70.61,1.35867816760341E-14,-44.5));
#53857=CARTESIAN_POINT('Origin',(70.61,18.0787611019615,-43.));
#53858=CARTESIAN_POINT('',(70.61,18.0787611019615,-46.5));
#53859=CARTESIAN_POINT('',(70.61,1.35867816760341E-14,-46.5));
#53860=CARTESIAN_POINT('',(70.61,18.0787611019615,-49.5));
#53861=CARTESIAN_POINT('',(70.61,1.35867816760341E-14,-49.5));
#53862=CARTESIAN_POINT('Origin',(70.61,18.0787611019615,-48.));
#53863=CARTESIAN_POINT('',(70.61,18.0787611019615,-51.5));
#53864=CARTESIAN_POINT('',(70.61,1.35867816760341E-14,-51.5));
#53865=CARTESIAN_POINT('',(70.61,18.0787611019615,-54.5));
#53866=CARTESIAN_POINT('',(70.61,1.35867816760341E-14,-54.5));
#53867=CARTESIAN_POINT('Origin',(70.61,18.0787611019615,-53.));
#53868=CARTESIAN_POINT('',(70.61,18.0787611019615,-11.5));
#53869=CARTESIAN_POINT('',(70.61,1.35867816760341E-14,-11.5));
#53870=CARTESIAN_POINT('',(70.61,18.0787611019615,-14.5));
#53871=CARTESIAN_POINT('',(70.61,1.35867816760341E-14,-14.5));
#53872=CARTESIAN_POINT('Origin',(70.61,18.0787611019615,-13.));
#53873=CARTESIAN_POINT('',(70.61,18.0787611019615,-26.5));
#53874=CARTESIAN_POINT('',(70.61,1.35867816760341E-14,-26.5));
#53875=CARTESIAN_POINT('',(70.61,18.0787611019615,-29.5));
#53876=CARTESIAN_POINT('',(70.61,1.35867816760341E-14,-29.5));
#53877=CARTESIAN_POINT('Origin',(70.61,18.0787611019615,-28.));
#53878=CARTESIAN_POINT('',(70.61,18.0787611019615,-21.5));
#53879=CARTESIAN_POINT('',(70.61,1.35867816760341E-14,-21.5));
#53880=CARTESIAN_POINT('',(70.61,18.0787611019615,-24.5));
#53881=CARTESIAN_POINT('',(70.61,1.35867816760341E-14,-24.5));
#53882=CARTESIAN_POINT('Origin',(70.61,18.0787611019615,-23.));
#53883=CARTESIAN_POINT('',(70.61,18.0787611019615,-16.5));
#53884=CARTESIAN_POINT('',(70.61,1.35867816760341E-14,-16.5));
#53885=CARTESIAN_POINT('',(70.61,18.0787611019615,-19.5));
#53886=CARTESIAN_POINT('',(70.61,1.35867816760341E-14,-19.5));
#53887=CARTESIAN_POINT('Origin',(70.61,18.0787611019615,-18.));
#53888=CARTESIAN_POINT('Origin',(69.81,91.,80.));
#53889=CARTESIAN_POINT('',(69.81,91.,75.));
#53890=CARTESIAN_POINT('',(69.81,91.,-75.));
#53891=CARTESIAN_POINT('',(69.81,91.,80.));
#53892=CARTESIAN_POINT('',(69.81,86.,-80.));
#53893=CARTESIAN_POINT('',(69.81,86.,-80.));
#53894=CARTESIAN_POINT('',(69.81,-1.84247779607698,-80.));
#53895=CARTESIAN_POINT('',(69.81,91.,-80.));
#53896=CARTESIAN_POINT('',(69.81,-1.84247779607698,-70.));
#53897=CARTESIAN_POINT('',(69.81,-1.84247779607698,-70.));
#53898=CARTESIAN_POINT('',(69.81,-2.4,-68.8330657242578));
#53899=CARTESIAN_POINT('Origin',(69.81,-3.34247779607698,-70.));
#53900=CARTESIAN_POINT('',(69.81,-2.4,68.8330657242578));
#53901=CARTESIAN_POINT('',(69.81,-2.4,80.));
#53902=CARTESIAN_POINT('',(69.81,-1.84247779607698,70.));
#53903=CARTESIAN_POINT('Origin',(69.81,-3.34247779607698,70.));
#53904=CARTESIAN_POINT('',(69.81,-1.84247779607698,80.));
#53905=CARTESIAN_POINT('',(69.81,-1.84247779607698,70.));
#53906=CARTESIAN_POINT('',(69.81,86.,80.));
#53907=CARTESIAN_POINT('',(69.81,91.,80.));
#53908=CARTESIAN_POINT('',(69.81,91.,75.));
#53909=CARTESIAN_POINT('',(69.81,18.0787611019615,-16.5));
#53910=CARTESIAN_POINT('',(69.81,91.,-16.5));
#53911=CARTESIAN_POINT('',(69.81,18.0787611019615,-19.5));
#53912=CARTESIAN_POINT('Origin',(69.81,18.0787611019615,-18.));
#53913=CARTESIAN_POINT('',(69.81,91.,-19.5));
#53914=CARTESIAN_POINT('',(69.81,18.0787611019615,-21.5));
#53915=CARTESIAN_POINT('',(69.81,91.,-21.5));
#53916=CARTESIAN_POINT('',(69.81,18.0787611019615,-24.5));
#53917=CARTESIAN_POINT('Origin',(69.81,18.0787611019615,-23.));
#53918=CARTESIAN_POINT('',(69.81,91.,-24.5));
#53919=CARTESIAN_POINT('',(69.81,46.0787611019615,-21.5));
#53920=CARTESIAN_POINT('',(69.81,91.,-21.5));
#53921=CARTESIAN_POINT('',(69.81,46.0787611019615,-24.5));
#53922=CARTESIAN_POINT('Origin',(69.81,46.0787611019615,-23.));
#53923=CARTESIAN_POINT('',(69.81,91.,-24.5));
#53924=CARTESIAN_POINT('',(69.81,46.0787611019615,-11.5));
#53925=CARTESIAN_POINT('',(69.81,91.,-11.5));
#53926=CARTESIAN_POINT('',(69.81,46.0787611019615,-14.5));
#53927=CARTESIAN_POINT('Origin',(69.81,46.0787611019615,-13.));
#53928=CARTESIAN_POINT('',(69.81,91.,-14.5));
#53929=CARTESIAN_POINT('',(69.81,46.0787611019615,-46.5));
#53930=CARTESIAN_POINT('',(69.81,91.,-46.5));
#53931=CARTESIAN_POINT('',(69.81,46.0787611019615,-49.5));
#53932=CARTESIAN_POINT('Origin',(69.81,46.0787611019615,-48.));
#53933=CARTESIAN_POINT('',(69.81,91.,-49.5));
#53934=CARTESIAN_POINT('',(69.81,46.0787611019615,-56.5));
#53935=CARTESIAN_POINT('',(69.81,91.,-56.5));
#53936=CARTESIAN_POINT('',(69.81,46.0787611019615,-59.5));
#53937=CARTESIAN_POINT('Origin',(69.81,46.0787611019615,-58.));
#53938=CARTESIAN_POINT('',(69.81,91.,-59.5));
#53939=CARTESIAN_POINT('',(69.81,46.0787611019615,-26.5));
#53940=CARTESIAN_POINT('',(69.81,91.,-26.5));
#53941=CARTESIAN_POINT('',(69.81,46.0787611019615,-29.5));
#53942=CARTESIAN_POINT('Origin',(69.81,46.0787611019615,-28.));
#53943=CARTESIAN_POINT('',(69.81,91.,-29.5));
#53944=CARTESIAN_POINT('',(69.81,18.0787611019615,-31.5));
#53945=CARTESIAN_POINT('',(69.81,91.,-31.5));
#53946=CARTESIAN_POINT('',(69.81,18.0787611019615,-34.5));
#53947=CARTESIAN_POINT('Origin',(69.81,18.0787611019615,-33.));
#53948=CARTESIAN_POINT('',(69.81,91.,-34.5));
#53949=CARTESIAN_POINT('',(69.81,18.0787611019615,-36.5));
#53950=CARTESIAN_POINT('',(69.81,91.,-36.5));
#53951=CARTESIAN_POINT('',(69.81,18.0787611019615,-39.5));
#53952=CARTESIAN_POINT('Origin',(69.81,18.0787611019615,-38.));
#53953=CARTESIAN_POINT('',(69.81,91.,-39.5));
#53954=CARTESIAN_POINT('',(69.81,18.0787611019615,-56.5));
#53955=CARTESIAN_POINT('',(69.81,91.,-56.5));
#53956=CARTESIAN_POINT('',(69.81,18.0787611019615,-59.5));
#53957=CARTESIAN_POINT('Origin',(69.81,18.0787611019615,-58.));
#53958=CARTESIAN_POINT('',(69.81,91.,-59.5));
#53959=CARTESIAN_POINT('',(69.81,18.0787611019615,-61.5));
#53960=CARTESIAN_POINT('',(69.81,91.,-61.5));
#53961=CARTESIAN_POINT('',(69.81,18.0787611019615,-64.5));
#53962=CARTESIAN_POINT('Origin',(69.81,18.0787611019615,-63.));
#53963=CARTESIAN_POINT('',(69.81,91.,-64.5));
#53964=CARTESIAN_POINT('',(69.81,18.0787611019615,-66.5));
#53965=CARTESIAN_POINT('',(69.81,91.,-66.5));
#53966=CARTESIAN_POINT('',(69.81,18.0787611019615,-69.5));
#53967=CARTESIAN_POINT('Origin',(69.81,18.0787611019615,-68.));
#53968=CARTESIAN_POINT('',(69.81,91.,-69.5));
#53969=CARTESIAN_POINT('',(69.81,46.0787611019615,-36.5));
#53970=CARTESIAN_POINT('',(69.81,91.,-36.5));
#53971=CARTESIAN_POINT('',(69.81,46.0787611019615,-39.5));
#53972=CARTESIAN_POINT('Origin',(69.81,46.0787611019615,-38.));
#53973=CARTESIAN_POINT('',(69.81,91.,-39.5));
#53974=CARTESIAN_POINT('',(69.81,18.0787611019615,21.5));
#53975=CARTESIAN_POINT('',(69.81,91.,21.5));
#53976=CARTESIAN_POINT('',(69.81,18.0787611019615,24.5));
#53977=CARTESIAN_POINT('',(69.81,91.,24.5));
#53978=CARTESIAN_POINT('Origin',(69.81,18.0787611019615,23.));
#53979=CARTESIAN_POINT('',(69.81,46.0787611019615,16.5));
#53980=CARTESIAN_POINT('',(69.81,91.,16.5));
#53981=CARTESIAN_POINT('',(69.81,46.0787611019615,19.5));
#53982=CARTESIAN_POINT('',(69.81,91.,19.5));
#53983=CARTESIAN_POINT('Origin',(69.81,46.0787611019615,18.));
#53984=CARTESIAN_POINT('',(69.81,46.0787611019615,11.5));
#53985=CARTESIAN_POINT('',(69.81,91.,11.5));
#53986=CARTESIAN_POINT('',(69.81,46.0787611019615,14.5));
#53987=CARTESIAN_POINT('',(69.81,91.,14.5));
#53988=CARTESIAN_POINT('Origin',(69.81,46.0787611019615,13.));
#53989=CARTESIAN_POINT('',(69.81,18.0787611019615,11.5));
#53990=CARTESIAN_POINT('',(69.81,91.,11.5));
#53991=CARTESIAN_POINT('',(69.81,18.0787611019615,14.5));
#53992=CARTESIAN_POINT('',(69.81,91.,14.5));
#53993=CARTESIAN_POINT('Origin',(69.81,18.0787611019615,13.));
#53994=CARTESIAN_POINT('',(69.81,18.0787611019615,46.5));
#53995=CARTESIAN_POINT('',(69.81,91.,46.5));
#53996=CARTESIAN_POINT('',(69.81,18.0787611019615,49.5));
#53997=CARTESIAN_POINT('',(69.81,91.,49.5));
#53998=CARTESIAN_POINT('Origin',(69.81,18.0787611019615,48.));
#53999=CARTESIAN_POINT('',(69.81,46.0787611019615,41.5));
#54000=CARTESIAN_POINT('',(69.81,91.,41.5));
#54001=CARTESIAN_POINT('',(69.81,46.0787611019615,44.5));
#54002=CARTESIAN_POINT('',(69.81,91.,44.5));
#54003=CARTESIAN_POINT('Origin',(69.81,46.0787611019615,43.));
#54004=CARTESIAN_POINT('',(69.81,46.0787611019615,46.5));
#54005=CARTESIAN_POINT('',(69.81,91.,46.5));
#54006=CARTESIAN_POINT('',(69.81,46.0787611019615,49.5));
#54007=CARTESIAN_POINT('',(69.81,91.,49.5));
#54008=CARTESIAN_POINT('Origin',(69.81,46.0787611019615,48.));
#54009=CARTESIAN_POINT('',(69.81,46.0787611019615,51.5));
#54010=CARTESIAN_POINT('',(69.81,91.,51.5));
#54011=CARTESIAN_POINT('',(69.81,46.0787611019615,54.5));
#54012=CARTESIAN_POINT('',(69.81,91.,54.5));
#54013=CARTESIAN_POINT('Origin',(69.81,46.0787611019615,53.));
#54014=CARTESIAN_POINT('',(69.81,46.0787611019615,56.5));
#54015=CARTESIAN_POINT('',(69.81,91.,56.5));
#54016=CARTESIAN_POINT('',(69.81,46.0787611019615,59.5));
#54017=CARTESIAN_POINT('',(69.81,91.,59.5));
#54018=CARTESIAN_POINT('Origin',(69.81,46.0787611019615,58.));
#54019=CARTESIAN_POINT('',(69.81,46.0787611019615,61.5));
#54020=CARTESIAN_POINT('',(69.81,91.,61.5));
#54021=CARTESIAN_POINT('',(69.81,46.0787611019615,64.5));
#54022=CARTESIAN_POINT('',(69.81,91.,64.5));
#54023=CARTESIAN_POINT('Origin',(69.81,46.0787611019615,63.));
#54024=CARTESIAN_POINT('',(69.81,46.0787611019615,26.5));
#54025=CARTESIAN_POINT('',(69.81,91.,26.5));
#54026=CARTESIAN_POINT('',(69.81,46.0787611019615,29.5));
#54027=CARTESIAN_POINT('',(69.81,91.,29.5));
#54028=CARTESIAN_POINT('Origin',(69.81,46.0787611019615,28.));
#54029=CARTESIAN_POINT('',(69.81,46.0787611019615,31.5));
#54030=CARTESIAN_POINT('',(69.81,91.,31.5));
#54031=CARTESIAN_POINT('',(69.81,46.0787611019615,34.5));
#54032=CARTESIAN_POINT('',(69.81,91.,34.5));
#54033=CARTESIAN_POINT('Origin',(69.81,46.0787611019615,33.));
#54034=CARTESIAN_POINT('',(69.81,18.0787611019615,31.5));
#54035=CARTESIAN_POINT('',(69.81,91.,31.5));
#54036=CARTESIAN_POINT('',(69.81,18.0787611019615,34.5));
#54037=CARTESIAN_POINT('',(69.81,91.,34.5));
#54038=CARTESIAN_POINT('Origin',(69.81,18.0787611019615,33.));
#54039=CARTESIAN_POINT('',(69.81,18.0787611019615,56.5));
#54040=CARTESIAN_POINT('',(69.81,91.,56.5));
#54041=CARTESIAN_POINT('',(69.81,18.0787611019615,59.5));
#54042=CARTESIAN_POINT('',(69.81,91.,59.5));
#54043=CARTESIAN_POINT('Origin',(69.81,18.0787611019615,58.));
#54044=CARTESIAN_POINT('',(69.81,18.0787611019615,66.5));
#54045=CARTESIAN_POINT('',(69.81,91.,66.5));
#54046=CARTESIAN_POINT('',(69.81,18.0787611019615,69.5));
#54047=CARTESIAN_POINT('',(69.81,91.,69.5));
#54048=CARTESIAN_POINT('Origin',(69.81,18.0787611019615,68.));
#54049=CARTESIAN_POINT('',(69.81,46.0787611019615,36.5));
#54050=CARTESIAN_POINT('',(69.81,91.,36.5));
#54051=CARTESIAN_POINT('',(69.81,46.0787611019615,39.5));
#54052=CARTESIAN_POINT('',(69.81,91.,39.5));
#54053=CARTESIAN_POINT('Origin',(69.81,46.0787611019615,38.));
#54054=CARTESIAN_POINT('',(69.81,18.0787611019615,61.5));
#54055=CARTESIAN_POINT('',(69.81,91.,61.5));
#54056=CARTESIAN_POINT('',(69.81,18.0787611019615,64.5));
#54057=CARTESIAN_POINT('',(69.81,91.,64.5));
#54058=CARTESIAN_POINT('Origin',(69.81,18.0787611019615,63.));
#54059=CARTESIAN_POINT('',(69.81,18.0787611019615,36.5));
#54060=CARTESIAN_POINT('',(69.81,91.,36.5));
#54061=CARTESIAN_POINT('',(69.81,18.0787611019615,39.5));
#54062=CARTESIAN_POINT('',(69.81,91.,39.5));
#54063=CARTESIAN_POINT('Origin',(69.81,18.0787611019615,38.));
#54064=CARTESIAN_POINT('',(69.81,18.0787611019615,41.5));
#54065=CARTESIAN_POINT('',(69.81,91.,41.5));
#54066=CARTESIAN_POINT('',(69.81,18.0787611019615,44.5));
#54067=CARTESIAN_POINT('',(69.81,91.,44.5));
#54068=CARTESIAN_POINT('Origin',(69.81,18.0787611019615,43.));
#54069=CARTESIAN_POINT('',(69.81,18.0787611019615,51.5));
#54070=CARTESIAN_POINT('',(69.81,91.,51.5));
#54071=CARTESIAN_POINT('',(69.81,18.0787611019615,54.5));
#54072=CARTESIAN_POINT('',(69.81,91.,54.5));
#54073=CARTESIAN_POINT('Origin',(69.81,18.0787611019615,53.));
#54074=CARTESIAN_POINT('',(69.81,18.0787611019615,26.5));
#54075=CARTESIAN_POINT('',(69.81,91.,26.5));
#54076=CARTESIAN_POINT('',(69.81,18.0787611019615,29.5));
#54077=CARTESIAN_POINT('',(69.81,91.,29.5));
#54078=CARTESIAN_POINT('Origin',(69.81,18.0787611019615,28.));
#54079=CARTESIAN_POINT('',(69.81,46.0787611019615,21.5));
#54080=CARTESIAN_POINT('',(69.81,91.,21.5));
#54081=CARTESIAN_POINT('',(69.81,46.0787611019615,24.5));
#54082=CARTESIAN_POINT('',(69.81,91.,24.5));
#54083=CARTESIAN_POINT('Origin',(69.81,46.0787611019615,23.));
#54084=CARTESIAN_POINT('',(69.81,18.0787611019615,16.5));
#54085=CARTESIAN_POINT('',(69.81,91.,16.5));
#54086=CARTESIAN_POINT('',(69.81,18.0787611019615,19.5));
#54087=CARTESIAN_POINT('',(69.81,91.,19.5));
#54088=CARTESIAN_POINT('Origin',(69.81,18.0787611019615,18.));
#54089=CARTESIAN_POINT('',(69.81,46.0787611019615,66.5));
#54090=CARTESIAN_POINT('',(69.81,91.,66.5));
#54091=CARTESIAN_POINT('',(69.81,46.0787611019615,69.5));
#54092=CARTESIAN_POINT('',(69.81,91.,69.5));
#54093=CARTESIAN_POINT('Origin',(69.81,46.0787611019615,68.));
#54094=CARTESIAN_POINT('',(69.81,46.0787611019615,-31.5));
#54095=CARTESIAN_POINT('',(69.81,91.,-31.5));
#54096=CARTESIAN_POINT('',(69.81,46.0787611019615,-34.5));
#54097=CARTESIAN_POINT('Origin',(69.81,46.0787611019615,-33.));
#54098=CARTESIAN_POINT('',(69.81,91.,-34.5));
#54099=CARTESIAN_POINT('',(69.81,46.0787611019615,-61.5));
#54100=CARTESIAN_POINT('',(69.81,91.,-61.5));
#54101=CARTESIAN_POINT('',(69.81,46.0787611019615,-64.5));
#54102=CARTESIAN_POINT('Origin',(69.81,46.0787611019615,-63.));
#54103=CARTESIAN_POINT('',(69.81,91.,-64.5));
#54104=CARTESIAN_POINT('',(69.81,46.0787611019615,-51.5));
#54105=CARTESIAN_POINT('',(69.81,91.,-51.5));
#54106=CARTESIAN_POINT('',(69.81,46.0787611019615,-54.5));
#54107=CARTESIAN_POINT('Origin',(69.81,46.0787611019615,-53.));
#54108=CARTESIAN_POINT('',(69.81,91.,-54.5));
#54109=CARTESIAN_POINT('',(69.81,46.0787611019615,-41.5));
#54110=CARTESIAN_POINT('',(69.81,91.,-41.5));
#54111=CARTESIAN_POINT('',(69.81,46.0787611019615,-44.5));
#54112=CARTESIAN_POINT('Origin',(69.81,46.0787611019615,-43.));
#54113=CARTESIAN_POINT('',(69.81,91.,-44.5));
#54114=CARTESIAN_POINT('',(69.81,18.0787611019615,-41.5));
#54115=CARTESIAN_POINT('',(69.81,91.,-41.5));
#54116=CARTESIAN_POINT('',(69.81,18.0787611019615,-44.5));
#54117=CARTESIAN_POINT('Origin',(69.81,18.0787611019615,-43.));
#54118=CARTESIAN_POINT('',(69.81,91.,-44.5));
#54119=CARTESIAN_POINT('',(69.81,18.0787611019615,-46.5));
#54120=CARTESIAN_POINT('',(69.81,91.,-46.5));
#54121=CARTESIAN_POINT('',(69.81,18.0787611019615,-49.5));
#54122=CARTESIAN_POINT('Origin',(69.81,18.0787611019615,-48.));
#54123=CARTESIAN_POINT('',(69.81,91.,-49.5));
#54124=CARTESIAN_POINT('',(69.81,18.0787611019615,-51.5));
#54125=CARTESIAN_POINT('',(69.81,91.,-51.5));
#54126=CARTESIAN_POINT('',(69.81,18.0787611019615,-54.5));
#54127=CARTESIAN_POINT('Origin',(69.81,18.0787611019615,-53.));
#54128=CARTESIAN_POINT('',(69.81,91.,-54.5));
#54129=CARTESIAN_POINT('',(69.81,18.0787611019615,-11.5));
#54130=CARTESIAN_POINT('',(69.81,91.,-11.5));
#54131=CARTESIAN_POINT('',(69.81,18.0787611019615,-14.5));
#54132=CARTESIAN_POINT('Origin',(69.81,18.0787611019615,-13.));
#54133=CARTESIAN_POINT('',(69.81,91.,-14.5));
#54134=CARTESIAN_POINT('',(69.81,46.0787611019615,-16.5));
#54135=CARTESIAN_POINT('',(69.81,91.,-16.5));
#54136=CARTESIAN_POINT('',(69.81,46.0787611019615,-19.5));
#54137=CARTESIAN_POINT('Origin',(69.81,46.0787611019615,-18.));
#54138=CARTESIAN_POINT('',(69.81,91.,-19.5));
#54139=CARTESIAN_POINT('',(69.81,18.0787611019615,-26.5));
#54140=CARTESIAN_POINT('',(69.81,91.,-26.5));
#54141=CARTESIAN_POINT('',(69.81,18.0787611019615,-29.5));
#54142=CARTESIAN_POINT('Origin',(69.81,18.0787611019615,-28.));
#54143=CARTESIAN_POINT('',(69.81,91.,-29.5));
#54144=CARTESIAN_POINT('',(69.81,46.0787611019615,-66.5));
#54145=CARTESIAN_POINT('',(69.81,91.,-66.5));
#54146=CARTESIAN_POINT('',(69.81,46.0787611019615,-69.5));
#54147=CARTESIAN_POINT('Origin',(69.81,46.0787611019615,-68.));
#54148=CARTESIAN_POINT('',(69.81,91.,-69.5));
#54149=CARTESIAN_POINT('Origin',(913.61,45.8777992076386,-29.25));
#54150=CARTESIAN_POINT('',(-86.39,34.9805523949445,-10.3754148577966));
#54151=CARTESIAN_POINT('',(-86.39,45.8777992076382,-29.25));
#54152=CARTESIAN_POINT('',(-85.5900000000001,34.9805523949445,-10.3754148577966));
#54153=CARTESIAN_POINT('',(-85.5900000000001,45.8777992076382,-29.25));
#54154=CARTESIAN_POINT('',(-86.39,34.9805523949445,-10.3754148577966));
#54155=CARTESIAN_POINT('Origin',(913.61,45.8777992076386,-29.25));
#54156=CARTESIAN_POINT('',(-85.5900000000001,59.7971840033556,-53.3590816762843));
#54157=CARTESIAN_POINT('',(-85.5900000000001,45.8777992076382,-29.25));
#54158=CARTESIAN_POINT('',(-86.39,59.7971840033556,-53.3590816762843));
#54159=CARTESIAN_POINT('',(-86.3899999999996,59.7971840033556,-53.3590816762843));
#54160=CARTESIAN_POINT('',(-86.39,45.8777992076382,-29.25));
#54161=CARTESIAN_POINT('Origin',(913.61,43.2797229962853,-30.75));
#54162=CARTESIAN_POINT('',(-86.39,57.199123585184,-54.8591090308774));
#54163=CARTESIAN_POINT('',(-86.39,54.1769698089785,-49.6245851422034));
#54164=CARTESIAN_POINT('',(-86.39,43.2797229962849,-30.75));
#54165=CARTESIAN_POINT('',(-85.5900000000001,57.199123585184,-54.8591090308774));
#54166=CARTESIAN_POINT('',(-85.5899999999993,57.1991235851839,-54.8591090308774));
#54167=CARTESIAN_POINT('',(-85.5900000000001,54.1769698089785,-49.6245851422034));
#54168=CARTESIAN_POINT('',(-85.5900000000001,43.2797229962849,-30.75));
#54169=CARTESIAN_POINT('',(-86.39,54.1769698089785,-49.6245851422034));
#54170=CARTESIAN_POINT('Origin',(913.61,45.8777992076386,-30.75));
#54171=CARTESIAN_POINT('',(-85.5900000000001,34.9805523949445,-49.6245851422034));
#54172=CARTESIAN_POINT('',(-85.5900000000001,45.8777992076382,-30.75));
#54173=CARTESIAN_POINT('',(-86.39,34.9805523949445,-49.6245851422034));
#54174=CARTESIAN_POINT('',(-86.39,45.8777992076382,-30.75));
#54175=CARTESIAN_POINT('',(-85.5899999999994,34.9805523949445,-49.6245851422034));
#54176=CARTESIAN_POINT('Origin',(913.61,43.2797229962853,-29.25));
#54177=CARTESIAN_POINT('',(-86.39,29.3603382005674,-53.3590816762843));
#54178=CARTESIAN_POINT('',(-86.39,32.3825102482842,-48.1245261404244));
#54179=CARTESIAN_POINT('',(-86.39,43.2797229962849,-29.25));
#54180=CARTESIAN_POINT('',(-85.5900000000001,29.3603382005674,-53.3590816762843));
#54181=CARTESIAN_POINT('',(-85.5899999999992,29.3603382005674,-53.3590816762843));
#54182=CARTESIAN_POINT('',(-85.5900000000001,32.3825102482842,-48.1245261404244));
#54183=CARTESIAN_POINT('',(-85.5900000000001,43.2797229962849,-29.25));
#54184=CARTESIAN_POINT('',(-86.3900000000001,32.3825102482842,-48.1245261404244));
#54185=CARTESIAN_POINT('Origin',(913.61,4.00385864813601E-13,-31.5));
#54186=CARTESIAN_POINT('',(-85.5900000000001,22.7843241379305,-31.5));
#54187=CARTESIAN_POINT('',(-85.5900000000001,-3.75094692148686E-14,-31.5));
#54188=CARTESIAN_POINT('',(-86.39,22.7843241379305,-31.5));
#54189=CARTESIAN_POINT('',(-86.39,-3.78600659594871E-14,-31.5));
#54190=CARTESIAN_POINT('',(-85.5899999999993,22.7843241379305,-31.5));
#54191=CARTESIAN_POINT('Origin',(913.61,4.00385864813601E-13,-28.5));
#54192=CARTESIAN_POINT('',(-86.39,22.7843241379304,-28.5));
#54193=CARTESIAN_POINT('',(-86.39,-3.78600659594871E-14,-28.5));
#54194=CARTESIAN_POINT('',(-85.5900000000001,22.7843241379304,-28.5));
#54195=CARTESIAN_POINT('',(-85.5900000000001,-3.75094692148686E-14,-28.5));
#54196=CARTESIAN_POINT('',(-86.3899999999997,22.7843241379304,-28.5));
#54197=CARTESIAN_POINT('Origin',(913.61,43.2797229962853,-30.75));
#54198=CARTESIAN_POINT('',(-85.5900000000001,29.3603382005675,-6.64091832371568));
#54199=CARTESIAN_POINT('',(-85.5900000000001,32.3825102482842,-11.8754738595756));
#54200=CARTESIAN_POINT('',(-85.5900000000001,43.2797229962849,-30.75));
#54201=CARTESIAN_POINT('',(-86.39,29.3603382005675,-6.64091832371568));
#54202=CARTESIAN_POINT('',(-86.3899999999997,29.3603382005675,-6.64091832371568));
#54203=CARTESIAN_POINT('',(-86.39,32.3825102482842,-11.8754738595756));
#54204=CARTESIAN_POINT('',(-86.39,43.2797229962849,-30.75));
#54205=CARTESIAN_POINT('',(-85.5899999999993,32.3825102482842,-11.8754738595756));
#54206=CARTESIAN_POINT('Origin',(913.61,43.2797229962853,-29.25));
#54207=CARTESIAN_POINT('',(-85.5900000000001,57.199123585184,-5.14089096912262));
#54208=CARTESIAN_POINT('',(-85.5900000000001,54.1769698089785,-10.3754148577966));
#54209=CARTESIAN_POINT('',(-85.5900000000001,43.2797229962849,-29.25));
#54210=CARTESIAN_POINT('',(-86.39,57.199123585184,-5.14089096912262));
#54211=CARTESIAN_POINT('',(-86.3899999999997,57.199123585184,-5.14089096912262));
#54212=CARTESIAN_POINT('',(-86.39,54.1769698089785,-10.3754148577966));
#54213=CARTESIAN_POINT('',(-86.39,43.2797229962849,-29.25));
#54214=CARTESIAN_POINT('',(-85.5899999999995,54.1769698089785,-10.3754148577966));
#54215=CARTESIAN_POINT('Origin',(913.61,45.8777992076386,-30.75));
#54216=CARTESIAN_POINT('',(-86.39,59.7971840033556,-6.6409183237157));
#54217=CARTESIAN_POINT('',(-86.39,45.8777992076382,-30.75));
#54218=CARTESIAN_POINT('',(-85.5900000000001,59.7971840033556,-6.6409183237157));
#54219=CARTESIAN_POINT('',(-85.5899999999992,59.7971840033556,-6.64091832371569));
#54220=CARTESIAN_POINT('',(-85.5900000000001,45.8777992076382,-30.75));
#54221=CARTESIAN_POINT('Origin',(913.61,4.00385864813601E-13,-28.5));
#54222=CARTESIAN_POINT('',(-85.5900000000001,72.4174689786827,-28.5));
#54223=CARTESIAN_POINT('',(-85.5900000000001,66.3731980659926,-28.5));
#54224=CARTESIAN_POINT('',(-85.5900000000001,-3.75094692148686E-14,-28.5));
#54225=CARTESIAN_POINT('',(-86.39,72.4174689786827,-28.5));
#54226=CARTESIAN_POINT('',(-86.3899999999997,72.4174689786827,-28.5));
#54227=CARTESIAN_POINT('',(-86.39,66.3731980659926,-28.5));
#54228=CARTESIAN_POINT('',(-86.39,-3.78600659594871E-14,-28.5));
#54229=CARTESIAN_POINT('',(-85.5899999999993,66.3731980659926,-28.5));
#54230=CARTESIAN_POINT('Origin',(913.61,4.00385864813601E-13,-31.5));
#54231=CARTESIAN_POINT('',(-85.5900000000001,66.3731980659926,-31.5));
#54232=CARTESIAN_POINT('',(-85.5900000000001,72.4174689786827,-31.5));
#54233=CARTESIAN_POINT('',(-85.5900000000001,-3.75094692148686E-14,-31.5));
#54234=CARTESIAN_POINT('',(-86.39,66.3731980659926,-31.5));
#54235=CARTESIAN_POINT('',(-86.39,66.3731980659926,-31.5));
#54236=CARTESIAN_POINT('',(-86.39,72.4174689786827,-31.5));
#54237=CARTESIAN_POINT('',(-86.39,-3.78600659594871E-14,-31.5));
#54238=CARTESIAN_POINT('',(-85.5900000000001,72.4174689786827,-31.5));
#54239=CARTESIAN_POINT('Origin',(913.61,45.8777992076386,-29.25));
#54240=CARTESIAN_POINT('',(-86.39,28.9441343457475,0.0799678991386249));
#54241=CARTESIAN_POINT('',(-86.39,45.8777992076382,-29.25));
#54242=CARTESIAN_POINT('',(-85.59,28.9441343457475,0.0799678991386249));
#54243=CARTESIAN_POINT('',(-85.5900000000001,45.8777992076382,-29.25));
#54244=CARTESIAN_POINT('',(-86.3900000000001,28.9441343457475,0.0799678991386144));
#54245=CARTESIAN_POINT('Origin',(913.61,45.8777992076386,-29.25));
#54246=CARTESIAN_POINT('',(-85.5900000000001,65.0692781609549,-62.4906166195334));
#54247=CARTESIAN_POINT('',(-85.5900000000001,45.8777992076382,-29.25));
#54248=CARTESIAN_POINT('',(-86.39,65.0692781609549,-62.4906166195334));
#54249=CARTESIAN_POINT('',(913.61,65.0692781609553,-62.4906166195334));
#54250=CARTESIAN_POINT('',(-86.39,45.8777992076382,-29.25));
#54251=CARTESIAN_POINT('Origin',(913.61,43.2797229962853,-30.75));
#54252=CARTESIAN_POINT('',(-86.39,62.471318048616,-63.990817708925));
#54253=CARTESIAN_POINT('',(-86.39,60.2133878581756,-60.0799678991386));
#54254=CARTESIAN_POINT('',(-86.39,43.2797229962849,-30.75));
#54255=CARTESIAN_POINT('',(-85.5900000000001,62.471318048616,-63.990817708925));
#54256=CARTESIAN_POINT('',(913.61,62.4713180486164,-63.990817708925));
#54257=CARTESIAN_POINT('',(-85.5900000000001,60.2133878581756,-60.0799678991386));
#54258=CARTESIAN_POINT('',(-85.5900000000001,43.2797229962849,-30.75));
#54259=CARTESIAN_POINT('',(-86.39,60.2133878581756,-60.0799678991386));
#54260=CARTESIAN_POINT('Origin',(913.61,45.8777992076386,-30.75));
#54261=CARTESIAN_POINT('',(-85.59,28.9441343457474,-60.0799678991386));
#54262=CARTESIAN_POINT('',(-85.5900000000001,45.8777992076382,-30.75));
#54263=CARTESIAN_POINT('',(-86.39,28.9441343457474,-60.0799678991386));
#54264=CARTESIAN_POINT('',(-86.39,45.8777992076382,-30.75));
#54265=CARTESIAN_POINT('',(-85.5899999999991,28.9441343457474,-60.0799678991386));
#54266=CARTESIAN_POINT('Origin',(913.61,43.2797229962853,-29.25));
#54267=CARTESIAN_POINT('',(-86.39,24.0882440265733,-62.49061664793));
#54268=CARTESIAN_POINT('',(-86.39,26.3460395813141,-58.5800000340158));
#54269=CARTESIAN_POINT('',(-86.39,43.2797229962849,-29.25));
#54270=CARTESIAN_POINT('',(-85.59,24.0882440265733,-62.49061664793));
#54271=CARTESIAN_POINT('',(913.61,24.0882440265737,-62.49061664793));
#54272=CARTESIAN_POINT('',(-85.59,26.3460395813141,-58.5800000340159));
#54273=CARTESIAN_POINT('',(-85.5900000000001,43.2797229962849,-29.25));
#54274=CARTESIAN_POINT('',(-86.3899999999997,26.3460395813141,-58.5800000340158));
#54275=CARTESIAN_POINT('Origin',(913.61,4.00385864813601E-13,-31.5));
#54276=CARTESIAN_POINT('',(-85.5900000000001,10.7114976242099,-31.5));
#54277=CARTESIAN_POINT('',(-85.5900000000001,-3.75094692148686E-14,-31.5));
#54278=CARTESIAN_POINT('',(-86.39,10.7114976242099,-31.5));
#54279=CARTESIAN_POINT('',(-86.39,-3.78600659594871E-14,-31.5));
#54280=CARTESIAN_POINT('',(-85.5899999999991,10.7114976242099,-31.5));
#54281=CARTESIAN_POINT('Origin',(913.61,4.00385864813601E-13,-28.5));
#54282=CARTESIAN_POINT('',(-86.39,10.7114976242099,-28.5));
#54283=CARTESIAN_POINT('',(-86.39,-3.78600659594871E-14,-28.5));
#54284=CARTESIAN_POINT('',(-85.5900000000001,10.7114976242099,-28.5));
#54285=CARTESIAN_POINT('',(-85.5900000000001,-3.75094692148686E-14,-28.5));
#54286=CARTESIAN_POINT('',(-86.39,10.7114976242099,-28.5));
#54287=CARTESIAN_POINT('Origin',(913.61,43.2797229962853,-30.75));
#54288=CARTESIAN_POINT('',(-85.59,24.0882440453297,2.49061661544304));
#54289=CARTESIAN_POINT('',(-85.59,26.3460395813141,-1.41999996598413));
#54290=CARTESIAN_POINT('',(-85.5900000000001,43.2797229962849,-30.75));
#54291=CARTESIAN_POINT('',(-86.39,24.0882440453297,2.49061661544304));
#54292=CARTESIAN_POINT('',(913.61,24.0882440453301,2.49061661544304));
#54293=CARTESIAN_POINT('',(-86.39,26.3460395813141,-1.41999996598413));
#54294=CARTESIAN_POINT('',(-86.39,43.2797229962849,-30.75));
#54295=CARTESIAN_POINT('',(-85.5899999999992,26.3460395813141,-1.41999996598414));
#54296=CARTESIAN_POINT('Origin',(913.61,43.2797229962853,-29.25));
#54297=CARTESIAN_POINT('',(-85.5900000000001,62.4713181477978,3.99081788071295));
#54298=CARTESIAN_POINT('',(-85.5900000000001,60.2133878581756,0.0799678991385971));
#54299=CARTESIAN_POINT('',(-85.5900000000001,43.2797229962849,-29.25));
#54300=CARTESIAN_POINT('',(-86.39,62.4713181477978,3.99081788071295));
#54301=CARTESIAN_POINT('',(913.61,62.4713181477983,3.99081788071295));
#54302=CARTESIAN_POINT('',(-86.39,60.2133878581756,0.0799678991385971));
#54303=CARTESIAN_POINT('',(-86.39,43.2797229962849,-29.25));
#54304=CARTESIAN_POINT('',(-85.5899999999993,60.2133878581756,0.079967899138597));
#54305=CARTESIAN_POINT('Origin',(913.61,45.8777992076386,-30.75));
#54306=CARTESIAN_POINT('',(-86.39,65.0692781797092,2.49061665201677));
#54307=CARTESIAN_POINT('',(-86.39,45.8777992076382,-30.75));
#54308=CARTESIAN_POINT('',(-85.5900000000001,65.0692781797092,2.49061665201677));
#54309=CARTESIAN_POINT('',(913.61,65.0692781797097,2.49061665201678));
#54310=CARTESIAN_POINT('',(-85.5900000000001,45.8777992076382,-30.75));
#54311=CARTESIAN_POINT('Origin',(913.61,4.00385864813601E-13,-28.5));
#54312=CARTESIAN_POINT('',(-85.5900000000001,82.9621121574678,-28.5));
#54313=CARTESIAN_POINT('',(-85.5900000000001,78.4460245797131,-28.5));
#54314=CARTESIAN_POINT('',(-85.5900000000001,-3.75094692148686E-14,-28.5));
#54315=CARTESIAN_POINT('',(-86.39,82.9621121574678,-28.5));
#54316=CARTESIAN_POINT('',(913.61,82.9621121574682,-28.5));
#54317=CARTESIAN_POINT('',(-86.39,78.4460245797131,-28.5));
#54318=CARTESIAN_POINT('',(-86.39,-3.78600659594871E-14,-28.5));
#54319=CARTESIAN_POINT('',(-85.5899999999993,78.4460245797131,-28.5));
#54320=CARTESIAN_POINT('Origin',(913.61,4.00385864813601E-13,-31.5));
#54321=CARTESIAN_POINT('',(-85.5900000000001,78.4460245797131,-31.5));
#54322=CARTESIAN_POINT('',(-85.5900000000001,82.9621122252415,-31.5));
#54323=CARTESIAN_POINT('',(-85.5900000000001,-3.75094692148686E-14,-31.5));
#54324=CARTESIAN_POINT('',(-86.39,78.4460245797131,-31.5));
#54325=CARTESIAN_POINT('',(-86.39,78.4460245797131,-31.5));
#54326=CARTESIAN_POINT('',(-86.39,82.9621122252415,-31.5));
#54327=CARTESIAN_POINT('',(-86.39,-3.78600659594871E-14,-31.5));
#54328=CARTESIAN_POINT('',(913.61,82.962112225242,-31.5));
#54329=CARTESIAN_POINT('Ctrl Pts',(-85.5899999999994,67.2171660490139,2.97732764444334));
#54330=CARTESIAN_POINT('Ctrl Pts',(-86.5499999999997,67.2171660490139,2.97732764444334));
#54331=CARTESIAN_POINT('Ctrl Pts',(-85.5899999999994,68.1584024122484,2.33128481848304));
#54332=CARTESIAN_POINT('Ctrl Pts',(-86.5499999999997,68.1584024122484,2.33128481848304));
#54333=CARTESIAN_POINT('Ctrl Pts',(-85.5899999999996,70.1198842128573,0.858367843285162));
#54334=CARTESIAN_POINT('Ctrl Pts',(-86.5499999999999,70.1198842128573,0.858367843285162));
#54335=CARTESIAN_POINT('Ctrl Pts',(-85.5899999999993,72.908047301324,-1.67045379084889));
#54336=CARTESIAN_POINT('Ctrl Pts',(-86.5499999999996,72.908047301324,-1.67045379084889));
#54337=CARTESIAN_POINT('Ctrl Pts',(-85.5899999999995,75.549548273606,-4.58281161933925));
#54338=CARTESIAN_POINT('Ctrl Pts',(-86.5499999999998,75.549548273606,-4.58281161933925));
#54339=CARTESIAN_POINT('Ctrl Pts',(-85.5899999999994,77.890528302476,-7.7415676465901));
#54340=CARTESIAN_POINT('Ctrl Pts',(-86.5499999999997,77.890528302476,-7.7415676465901));
#54341=CARTESIAN_POINT('Ctrl Pts',(-85.5899999999993,79.9131007484785,-11.1132966089213));
#54342=CARTESIAN_POINT('Ctrl Pts',(-86.5499999999996,79.9131007484785,-11.1132966089213));
#54343=CARTESIAN_POINT('Ctrl Pts',(-85.5899999999992,81.5928567717819,-14.6680605730953));
#54344=CARTESIAN_POINT('Ctrl Pts',(-86.5499999999995,81.5928567717819,-14.6680605730953));
#54345=CARTESIAN_POINT('Ctrl Pts',(-85.5899999999995,82.9187743664602,-18.3695870184804));
#54346=CARTESIAN_POINT('Ctrl Pts',(-86.5499999999998,82.9187743664602,-18.3695870184804));
#54347=CARTESIAN_POINT('Ctrl Pts',(-85.5899999999994,83.8727543022822,-22.1837513334676));
#54348=CARTESIAN_POINT('Ctrl Pts',(-86.5499999999997,83.8727543022822,-22.1837513334676));
#54349=CARTESIAN_POINT('Ctrl Pts',(-85.5899999999993,84.2979204495417,-25.0429582798392));
#54350=CARTESIAN_POINT('Ctrl Pts',(-86.5499999999996,84.2979204495417,-25.0429582798392));
#54351=CARTESIAN_POINT('Ctrl Pts',(-85.5899999999994,84.4366282617325,-26.6149733080415));
#54352=CARTESIAN_POINT('Ctrl Pts',(-86.5499999999997,84.4366282617325,-26.6149733080415));
#54353=CARTESIAN_POINT('Ctrl Pts',(-85.5899999999994,84.4575664621194,-26.8833105716064));
#54354=CARTESIAN_POINT('Ctrl Pts',(-86.5499999999997,84.4575664621194,-26.8833105716064));
#54355=CARTESIAN_POINT('',(-85.5899999999998,84.45756646212,-26.8833105716133));
#54356=CARTESIAN_POINT('',(-85.5899999999998,67.2171660490092,2.97732764444655));
#54357=CARTESIAN_POINT('Ctrl Pts',(-85.5899999999998,84.45756646212,-26.8833105716133));
#54358=CARTESIAN_POINT('Ctrl Pts',(-85.5899999999998,84.4366282617329,-26.6149733080461));
#54359=CARTESIAN_POINT('Ctrl Pts',(-85.5899999999997,84.297920449542,-25.0429582798415));
#54360=CARTESIAN_POINT('Ctrl Pts',(-85.5899999999998,83.8727543022822,-22.1837513334676));
#54361=CARTESIAN_POINT('Ctrl Pts',(-85.59,82.9187743664602,-18.3695870184804));
#54362=CARTESIAN_POINT('Ctrl Pts',(-85.5899999999996,81.5928567717819,-14.6680605730953));
#54363=CARTESIAN_POINT('Ctrl Pts',(-85.5899999999997,79.9131007484785,-11.1132966089213));
#54364=CARTESIAN_POINT('Ctrl Pts',(-85.5899999999998,77.890528302476,-7.7415676465901));
#54365=CARTESIAN_POINT('Ctrl Pts',(-85.59,75.549548273606,-4.58281161933925));
#54366=CARTESIAN_POINT('Ctrl Pts',(-85.5899999999997,72.908047301324,-1.67045379084889));
#54367=CARTESIAN_POINT('Ctrl Pts',(-85.59,70.1198842128559,0.858367843286441));
#54368=CARTESIAN_POINT('Ctrl Pts',(-85.5899999999999,68.1584024122454,2.33128481848532));
#54369=CARTESIAN_POINT('Ctrl Pts',(-85.5899999999998,67.2171660490092,2.97732764444655));
#54370=CARTESIAN_POINT('',(-86.3899999999999,67.2171660490092,2.97732764444655));
#54371=CARTESIAN_POINT('',(-85.5899999999998,67.2171660490092,2.97732764444655));
#54372=CARTESIAN_POINT('',(-86.3899999999998,84.45756646212,-26.8833105716133));
#54373=CARTESIAN_POINT('Ctrl Pts',(-86.3899999999998,84.45756646212,-26.8833105716133));
#54374=CARTESIAN_POINT('Ctrl Pts',(-86.3899999999998,84.4366282617329,-26.6149733080461));
#54375=CARTESIAN_POINT('Ctrl Pts',(-86.3899999999998,84.297920449542,-25.0429582798415));
#54376=CARTESIAN_POINT('Ctrl Pts',(-86.3899999999999,83.8727543022822,-22.1837513334676));
#54377=CARTESIAN_POINT('Ctrl Pts',(-86.39,82.9187743664602,-18.3695870184804));
#54378=CARTESIAN_POINT('Ctrl Pts',(-86.3899999999996,81.5928567717819,-14.6680605730953));
#54379=CARTESIAN_POINT('Ctrl Pts',(-86.3899999999997,79.9131007484785,-11.1132966089213));
#54380=CARTESIAN_POINT('Ctrl Pts',(-86.3899999999999,77.890528302476,-7.7415676465901));
#54381=CARTESIAN_POINT('Ctrl Pts',(-86.39,75.549548273606,-4.58281161933925));
#54382=CARTESIAN_POINT('Ctrl Pts',(-86.3899999999997,72.908047301324,-1.67045379084889));
#54383=CARTESIAN_POINT('Ctrl Pts',(-86.3900000000001,70.1198842128559,0.858367843286441));
#54384=CARTESIAN_POINT('Ctrl Pts',(-86.3899999999999,68.1584024122454,2.33128481848532));
#54385=CARTESIAN_POINT('Ctrl Pts',(-86.3899999999999,67.2171660490092,2.97732764444655));
#54386=CARTESIAN_POINT('',(-86.39,84.45756646212,-26.8833105716133));
#54387=CARTESIAN_POINT('Origin',(-85.59,44.5787611019615,-30.));
#54388=CARTESIAN_POINT('Origin',(-85.59,55.9000854795073,-4.39089096912261));
#54389=CARTESIAN_POINT('',(-85.5900000000002,52.3121016227476,-11.0146003457498));
#54390=CARTESIAN_POINT('Origin',(-85.59,52.8779317033019,-9.62541485779658));
#54391=CARTESIAN_POINT('Ctrl Pts',(-85.5900000000002,52.3121016227476,-11.0146003457498));
#54392=CARTESIAN_POINT('Ctrl Pts',(-85.5900000000002,51.1067797000298,-10.5236598582919));
#54393=CARTESIAN_POINT('Ctrl Pts',(-85.59,48.5636521071369,-9.76033053440373));
#54394=CARTESIAN_POINT('Ctrl Pts',(-85.5900000000001,45.9204718342386,-9.5));
#54395=CARTESIAN_POINT('Ctrl Pts',(-85.5900000000001,44.5787611019615,-9.5));
#54396=CARTESIAN_POINT('Origin',(-85.59,36.2795905006212,-9.62541485779656));
#54397=CARTESIAN_POINT('Ctrl Pts',(-85.5900000000003,44.5787611019615,-0.5));
#54398=CARTESIAN_POINT('Ctrl Pts',(-85.5900000000003,42.6480066335628,-0.5));
#54399=CARTESIAN_POINT('Ctrl Pts',(-85.5899999999998,38.7864976967653,-0.880325434261422));
#54400=CARTESIAN_POINT('Ctrl Pts',(-85.59,34.8506764348827,-2.07424376132475));
#54401=CARTESIAN_POINT('Ctrl Pts',(-85.59,32.8626902557764,-2.92534739713371));
#54402=CARTESIAN_POINT('Ctrl Pts',(-85.59,32.6508629759237,-3.01900602947195));
#54403=CARTESIAN_POINT('',(-85.5900000000001,51.1378158375422,-15.6393839483491));
#54404=CARTESIAN_POINT('Origin',(-85.59,49.8387777318655,-14.8893839483491));
#54405=CARTESIAN_POINT('',(-85.5900000000001,47.7866618629516,-21.4437528963263));
#54406=CARTESIAN_POINT('',(-85.5900000000001,43.2797229962849,-29.25));
#54407=CARTESIAN_POINT('',(-85.5900000000003,46.1862026525626,-22.1631559443816));
#54408=CARTESIAN_POINT('Origin',(-85.59,46.487623757275,-20.6937528963263));
#54409=CARTESIAN_POINT('Ctrl Pts',(-85.5900000000003,46.1862026525626,-22.1631559443815));
#54410=CARTESIAN_POINT('Ctrl Pts',(-85.5900000000003,46.1706391043624,-22.1599633677104));
#54411=CARTESIAN_POINT('Ctrl Pts',(-85.5900000000003,46.1550660227809,-22.1568172778458));
#54412=CARTESIAN_POINT('Ctrl Pts',(-85.5900000000003,46.1394836780905,-22.1537177567742));
#54413=CARTESIAN_POINT('Ctrl Pts',(-85.5900000000004,45.6259499661778,-22.0515695504083));
#54414=CARTESIAN_POINT('Ctrl Pts',(-85.5900000000005,45.1023555340697,-22.));
#54415=CARTESIAN_POINT('Ctrl Pts',(-85.5900000000004,44.5787611019615,-22.));
#54416=CARTESIAN_POINT('',(-85.5900000000001,41.3708603409714,-21.4437528963263));
#54417=CARTESIAN_POINT('Origin',(-85.59,42.6698984466481,-20.6937528963263));
#54418=CARTESIAN_POINT('',(-85.5900000000001,45.8777992076382,-29.25));
#54419=CARTESIAN_POINT('Ctrl Pts',(-85.5899999999998,44.5787611019615,-12.5));
#54420=CARTESIAN_POINT('Ctrl Pts',(-85.5899999999998,43.433398281725,-12.5));
#54421=CARTESIAN_POINT('Ctrl Pts',(-85.5900000000001,41.4793849628696,-12.6924535139527));
#54422=CARTESIAN_POINT('Ctrl Pts',(-85.59,39.5894256076692,-13.2069280490151));
#54423=CARTESIAN_POINT('Ctrl Pts',(-85.59,38.8257009268133,-13.4727301224294));
#54424=CARTESIAN_POINT('',(-85.5900000000001,60.2949931567668,-28.5));
#54425=CARTESIAN_POINT('',(-85.5900000000001,53.5926110635042,-28.5));
#54426=CARTESIAN_POINT('',(-85.5900000000001,-3.75094692148686E-14,-28.5));
#54427=CARTESIAN_POINT('',(-85.5900000000001,52.1693515320421,-27.4736373149388));
#54428=CARTESIAN_POINT('Origin',(-85.59,53.5926110635042,-27.));
#54429=CARTESIAN_POINT('Ctrl Pts',(-85.5900000000001,52.1693515320421,-27.4736373149388));
#54430=CARTESIAN_POINT('Ctrl Pts',(-85.5900000000001,52.1092282262333,-27.2929693959288));
#54431=CARTESIAN_POINT('Ctrl Pts',(-85.5900000000001,51.8596181813086,-26.6235312275074));
#54432=CARTESIAN_POINT('Ctrl Pts',(-85.5900000000001,51.3485297861122,-25.6673520933024));
#54433=CARTESIAN_POINT('Ctrl Pts',(-85.5900000000002,50.8041422375675,-24.9624237973926));
#54434=CARTESIAN_POINT('Ctrl Pts',(-85.5900000000003,50.5618748736031,-24.689445144648));
#54435=CARTESIAN_POINT('',(-85.5900000000001,53.7358855886589,-17.139395137807));
#54436=CARTESIAN_POINT('',(-85.5900000000001,45.8777992076382,-30.75));
#54437=CARTESIAN_POINT('',(-85.5900000000001,56.0151454704897,-16.7539809977007));
#54438=CARTESIAN_POINT('Origin',(-85.59,55.0349236943356,-17.889395137807));
#54439=CARTESIAN_POINT('',(-85.5900000000001,61.7683968689589,-26.7187856673305));
#54440=CARTESIAN_POINT('Ctrl Pts',(-85.5900000000001,61.7683968689589,-26.7187856673305));
#54441=CARTESIAN_POINT('Ctrl Pts',(-85.5900000000001,61.7599375519114,-26.6744636407038));
#54442=CARTESIAN_POINT('Ctrl Pts',(-85.5900000000001,61.5322159292861,-25.5059524219445));
#54443=CARTESIAN_POINT('Ctrl Pts',(-85.5900000000002,60.8508742849282,-23.2598700311452));
#54444=CARTESIAN_POINT('Ctrl Pts',(-85.5900000000001,59.2232760668162,-20.2148479377946));
#54445=CARTESIAN_POINT('Ctrl Pts',(-85.59,57.4908812316918,-18.1039187234852));
#54446=CARTESIAN_POINT('Ctrl Pts',(-85.5900000000001,56.3382988733575,-17.0329646666021));
#54447=CARTESIAN_POINT('Ctrl Pts',(-85.5900000000001,56.0151454704897,-16.7539809977007));
#54448=CARTESIAN_POINT('Origin',(-85.59,60.2949931567668,-27.));
#54449=CARTESIAN_POINT('',(-85.5900000000001,53.7358855886589,-42.860604862193));
#54450=CARTESIAN_POINT('',(-85.5900000000001,45.8777992076382,-29.25));
#54451=CARTESIAN_POINT('',(-85.5900000000003,52.1693515320421,-32.5263626850612));
#54452=CARTESIAN_POINT('Ctrl Pts',(-85.5900000000003,50.5618748736031,-35.310554855352));
#54453=CARTESIAN_POINT('Ctrl Pts',(-85.5900000000003,50.8041422375675,-35.0375762026074));
#54454=CARTESIAN_POINT('Ctrl Pts',(-85.5900000000005,51.3485297861122,-34.3326479066976));
#54455=CARTESIAN_POINT('Ctrl Pts',(-85.5900000000003,51.8596181813085,-33.3764687724926));
#54456=CARTESIAN_POINT('Ctrl Pts',(-85.5900000000003,52.1092282262332,-32.7070306040712));
#54457=CARTESIAN_POINT('Ctrl Pts',(-85.5900000000003,52.1693515320421,-32.5263626850612));
#54458=CARTESIAN_POINT('',(-85.5900000000001,53.5926110635042,-31.5));
#54459=CARTESIAN_POINT('Origin',(-85.59,53.5926110635042,-32.9999999999999));
#54460=CARTESIAN_POINT('',(-85.5900000000001,60.2949931567668,-31.5));
#54461=CARTESIAN_POINT('',(-85.5900000000001,-3.75094692148686E-14,-31.5));
#54462=CARTESIAN_POINT('',(-85.5900000000002,61.7683968689589,-33.2812143326695));
#54463=CARTESIAN_POINT('Origin',(-85.59,60.2949931567668,-33.));
#54464=CARTESIAN_POINT('',(-85.5900000000001,56.0151454704896,-43.2460190022993));
#54465=CARTESIAN_POINT('Ctrl Pts',(-85.5900000000001,56.0151454704896,-43.2460190022993));
#54466=CARTESIAN_POINT('Ctrl Pts',(-85.5900000000001,56.3382988733575,-42.9670353333979));
#54467=CARTESIAN_POINT('Ctrl Pts',(-85.59,57.4908812316918,-41.8960812765148));
#54468=CARTESIAN_POINT('Ctrl Pts',(-85.59,59.2232760668162,-39.7851520622054));
#54469=CARTESIAN_POINT('Ctrl Pts',(-85.59,60.8508742849283,-36.7401299688548));
#54470=CARTESIAN_POINT('Ctrl Pts',(-85.5900000000002,61.5322159292861,-34.4940475780555));
#54471=CARTESIAN_POINT('Ctrl Pts',(-85.5900000000002,61.7599375519113,-33.3255363592962));
#54472=CARTESIAN_POINT('Ctrl Pts',(-85.5900000000002,61.7683968689589,-33.2812143326695));
#54473=CARTESIAN_POINT('Origin',(-85.59,55.0349236943356,-42.110604862193));
#54474=CARTESIAN_POINT('',(-85.5900000000001,41.3708603409714,-38.5562471036737));
#54475=CARTESIAN_POINT('',(-85.5900000000001,45.8777992076382,-30.75));
#54476=CARTESIAN_POINT('',(-85.5900000000002,42.9713195513605,-37.8368440556185));
#54477=CARTESIAN_POINT('Origin',(-85.59,42.6698984466481,-39.3062471036737));
#54478=CARTESIAN_POINT('',(-85.5900000000002,46.1862026525626,-37.8368440556185));
#54479=CARTESIAN_POINT('Ctrl Pts',(-85.5900000000002,42.9713195513605,-37.8368440556185));
#54480=CARTESIAN_POINT('Ctrl Pts',(-85.5900000000002,42.9868830995607,-37.8400366322896));
#54481=CARTESIAN_POINT('Ctrl Pts',(-85.5900000000001,43.5156846168748,-37.9468656555161));
#54482=CARTESIAN_POINT('Ctrl Pts',(-85.5900000000003,44.5787611019615,-38.0515695504083));
#54483=CARTESIAN_POINT('Ctrl Pts',(-85.5900000000001,45.6418375870482,-37.9468656555161));
#54484=CARTESIAN_POINT('Ctrl Pts',(-85.5900000000002,46.1706391043624,-37.8400366322896));
#54485=CARTESIAN_POINT('Ctrl Pts',(-85.5900000000002,46.1862026525626,-37.8368440556185));
#54486=CARTESIAN_POINT('',(-85.5900000000001,47.7866618629516,-38.5562471036737));
#54487=CARTESIAN_POINT('Origin',(-85.59,46.4876237572749,-39.3062471036737));
#54488=CARTESIAN_POINT('',(-85.5900000000001,51.1378158375422,-44.3606160516509));
#54489=CARTESIAN_POINT('',(-85.5900000000001,43.2797229962849,-30.75));
#54490=CARTESIAN_POINT('',(-85.59,50.3318212771098,-46.5272698775706));
#54491=CARTESIAN_POINT('Origin',(-85.59,49.8387777318655,-45.1106160516509));
#54492=CARTESIAN_POINT('Ctrl Pts',(-85.59,38.8257009268133,-46.5272698775706));
#54493=CARTESIAN_POINT('Ctrl Pts',(-85.5900000000001,39.5894256076692,-46.793071950985));
#54494=CARTESIAN_POINT('Ctrl Pts',(-85.5900000000001,41.4793849628696,-47.3075464860474));
#54495=CARTESIAN_POINT('Ctrl Pts',(-85.59,44.5787611019615,-47.6128083915182));
#54496=CARTESIAN_POINT('Ctrl Pts',(-85.5900000000002,47.6781372410534,-47.3075464860473));
#54497=CARTESIAN_POINT('Ctrl Pts',(-85.5900000000001,49.5680965962538,-46.793071950985));
#54498=CARTESIAN_POINT('Ctrl Pts',(-85.59,50.3318212771098,-46.5272698775706));
#54499=CARTESIAN_POINT('',(-85.5900000000001,35.5649111404189,-31.5));
#54500=CARTESIAN_POINT('',(-85.5900000000001,-3.75094692148686E-14,-31.5));
#54501=CARTESIAN_POINT('',(-85.5900000000004,36.988170671881,-32.5263626850613));
#54502=CARTESIAN_POINT('Origin',(-85.59,35.5649111404189,-33.));
#54503=CARTESIAN_POINT('',(-85.5900000000003,38.5956473303199,-35.3105548553519));
#54504=CARTESIAN_POINT('Ctrl Pts',(-85.5900000000004,36.988170671881,-32.5263626850613));
#54505=CARTESIAN_POINT('Ctrl Pts',(-85.5900000000004,37.0482939776898,-32.7070306040712));
#54506=CARTESIAN_POINT('Ctrl Pts',(-85.5900000000004,37.2979040226145,-33.3764687724926));
#54507=CARTESIAN_POINT('Ctrl Pts',(-85.5900000000002,37.8089924178108,-34.3326479066976));
#54508=CARTESIAN_POINT('Ctrl Pts',(-85.5900000000003,38.3533799663555,-35.0375762026073));
#54509=CARTESIAN_POINT('Ctrl Pts',(-85.5900000000003,38.5956473303199,-35.3105548553519));
#54510=CARTESIAN_POINT('',(-85.5900000000001,38.7727956517265,-37.0562271467965));
#54511=CARTESIAN_POINT('Origin',(-85.59,37.4737575460498,-36.3062271467965));
#54512=CARTESIAN_POINT('',(-85.5900000000001,35.4216366152641,-42.860604862193));
#54513=CARTESIAN_POINT('',(-85.5900000000001,43.2797229962849,-29.25));
#54514=CARTESIAN_POINT('',(-85.5900000000001,33.1423767334334,-43.2460190022993));
#54515=CARTESIAN_POINT('Origin',(-85.59,34.1225985095874,-42.110604862193));
#54516=CARTESIAN_POINT('Ctrl Pts',(-85.5900000000001,27.3891253349642,-33.2812143326694));
#54517=CARTESIAN_POINT('Ctrl Pts',(-85.5900000000001,27.3975846520117,-33.3255363592962));
#54518=CARTESIAN_POINT('Ctrl Pts',(-85.59,27.625306274637,-34.4940475780555));
#54519=CARTESIAN_POINT('Ctrl Pts',(-85.59,28.3066479189948,-36.7401299688549));
#54520=CARTESIAN_POINT('Ctrl Pts',(-85.59,29.9342461371069,-39.7851520622054));
#54521=CARTESIAN_POINT('Ctrl Pts',(-85.59,31.6666409722312,-41.8960812765148));
#54522=CARTESIAN_POINT('Ctrl Pts',(-85.5900000000001,32.8192233305655,-42.9670353333979));
#54523=CARTESIAN_POINT('Ctrl Pts',(-85.5900000000001,33.1423767334334,-43.2460190022993));
#54524=CARTESIAN_POINT('',(-85.5900000000001,35.4216366152641,-17.139395137807));
#54525=CARTESIAN_POINT('',(-85.5900000000001,38.7727956517265,-22.9437728532035));
#54526=CARTESIAN_POINT('',(-85.5900000000001,43.2797229962849,-30.75));
#54527=CARTESIAN_POINT('',(-85.5900000000003,38.5956473303199,-24.6894451446481));
#54528=CARTESIAN_POINT('Origin',(-85.59,37.4737575460499,-23.6937728532035));
#54529=CARTESIAN_POINT('',(-85.5900000000003,36.988170671881,-27.4736373149387));
#54530=CARTESIAN_POINT('Ctrl Pts',(-85.5900000000003,38.5956473303199,-24.6894451446481));
#54531=CARTESIAN_POINT('Ctrl Pts',(-85.5900000000003,38.3533799663555,-24.9624237973927));
#54532=CARTESIAN_POINT('Ctrl Pts',(-85.5900000000002,37.8089924178108,-25.6673520933024));
#54533=CARTESIAN_POINT('Ctrl Pts',(-85.5900000000004,37.2979040226145,-26.6235312275074));
#54534=CARTESIAN_POINT('Ctrl Pts',(-85.5900000000003,37.0482939776898,-27.2929693959288));
#54535=CARTESIAN_POINT('Ctrl Pts',(-85.5900000000003,36.988170671881,-27.4736373149387));
#54536=CARTESIAN_POINT('',(-85.5900000000001,35.5649111404189,-28.5));
#54537=CARTESIAN_POINT('Origin',(-85.59,35.5649111404189,-27.));
#54538=CARTESIAN_POINT('',(-85.5900000000001,-3.75094692148686E-14,-28.5));
#54539=CARTESIAN_POINT('',(-85.5900000000001,33.1423767334334,-16.7539809977007));
#54540=CARTESIAN_POINT('Ctrl Pts',(-85.5900000000001,33.1423767334334,-16.7539809977007));
#54541=CARTESIAN_POINT('Ctrl Pts',(-85.5900000000001,32.8192233305655,-17.0329646666021));
#54542=CARTESIAN_POINT('Ctrl Pts',(-85.5900000000001,31.6666409722312,-18.1039187234852));
#54543=CARTESIAN_POINT('Ctrl Pts',(-85.59,29.9342461371069,-20.2148479377946));
#54544=CARTESIAN_POINT('Ctrl Pts',(-85.5900000000004,28.3066479189948,-23.2598700311452));
#54545=CARTESIAN_POINT('Ctrl Pts',(-85.5900000000002,27.625306274637,-25.5059524219445));
#54546=CARTESIAN_POINT('Ctrl Pts',(-85.5900000000002,27.3975846520117,-26.6744636407038));
#54547=CARTESIAN_POINT('Ctrl Pts',(-85.5900000000002,27.3891253349642,-26.7187856673305));
#54548=CARTESIAN_POINT('Origin',(-85.59,34.1225985095875,-17.889395137807));
#54549=CARTESIAN_POINT('',(-85.59,64.8871997650542,-27.204472613345));
#54550=CARTESIAN_POINT('Origin',(-85.59,66.3731980659926,-27.));
#54551=CARTESIAN_POINT('Ctrl Pts',(-85.59,64.8871997650542,-27.204472613345));
#54552=CARTESIAN_POINT('Ctrl Pts',(-85.59,64.8317241956999,-26.8013056539391));
#54553=CARTESIAN_POINT('Ctrl Pts',(-85.59,64.5418111191102,-25.0760413061512));
#54554=CARTESIAN_POINT('Ctrl Pts',(-85.59,63.6403794020083,-22.1044191793415));
#54555=CARTESIAN_POINT('Ctrl Pts',(-85.5900000000001,61.7337643465056,-18.5373932985594));
#54556=CARTESIAN_POINT('Ctrl Pts',(-85.5900000000001,59.4786368856789,-15.7895125368918));
#54557=CARTESIAN_POINT('Ctrl Pts',(-85.5900000000001,57.8284952042271,-14.334111510217));
#54558=CARTESIAN_POINT('Ctrl Pts',(-85.5900000000001,57.1538693431447,-13.8100697594109));
#54559=CARTESIAN_POINT('',(-85.5900000000001,61.9811659354668,-6.17977241010521));
#54560=CARTESIAN_POINT('Origin',(-85.59,61.0962221090323,-7.39091832371568));
#54561=CARTESIAN_POINT('',(-85.59,73.9088368640223,-26.8393082747068));
#54562=CARTESIAN_POINT('Ctrl Pts',(-85.59,73.9088368640223,-26.8393082747068));
#54563=CARTESIAN_POINT('Ctrl Pts',(-85.59,73.81508077238,-25.9691649995929));
#54564=CARTESIAN_POINT('Ctrl Pts',(-85.5900000000001,73.3905329456488,-23.1927173488711));
#54565=CARTESIAN_POINT('Ctrl Pts',(-85.59,72.0088947532483,-18.6380666239304));
#54566=CARTESIAN_POINT('Ctrl Pts',(-85.59,69.2652291855737,-13.5050293808538));
#54567=CARTESIAN_POINT('Ctrl Pts',(-85.5900000000002,65.8355371052187,-9.32593748926008));
#54568=CARTESIAN_POINT('Ctrl Pts',(-85.5900000000001,63.2074283898593,-7.07576138749285));
#54569=CARTESIAN_POINT('Ctrl Pts',(-85.5900000000001,61.9811659354668,-6.17977241010521));
#54570=CARTESIAN_POINT('Origin',(-85.59,72.4174689786827,-27.));
#54571=CARTESIAN_POINT('',(-85.5900000000001,64.8871997650542,-32.795527386655));
#54572=CARTESIAN_POINT('Ctrl Pts',(-85.59,57.1538693431447,-46.1899302405891));
#54573=CARTESIAN_POINT('Ctrl Pts',(-85.59,57.8284952042271,-45.665888489783));
#54574=CARTESIAN_POINT('Ctrl Pts',(-85.5900000000001,59.4786368856789,-44.2104874631082));
#54575=CARTESIAN_POINT('Ctrl Pts',(-85.5900000000001,61.7337643465056,-41.4626067014406));
#54576=CARTESIAN_POINT('Ctrl Pts',(-85.59,63.6403794020083,-37.8955808206585));
#54577=CARTESIAN_POINT('Ctrl Pts',(-85.59,64.5418111191102,-34.9239586938488));
#54578=CARTESIAN_POINT('Ctrl Pts',(-85.5900000000001,64.8317241956999,-33.1986943460608));
#54579=CARTESIAN_POINT('Ctrl Pts',(-85.5900000000001,64.8871997650542,-32.795527386655));
#54580=CARTESIAN_POINT('Origin',(-85.59,66.3731980659926,-33.));
#54581=CARTESIAN_POINT('',(-85.5899999999999,73.9088368640223,-33.1606917252932));
#54582=CARTESIAN_POINT('Origin',(-85.59,72.4174689786827,-33.));
#54583=CARTESIAN_POINT('',(-85.5900000000001,61.9811659354668,-53.8202275898948));
#54584=CARTESIAN_POINT('Ctrl Pts',(-85.5900000000001,61.9811659354668,-53.8202275898948));
#54585=CARTESIAN_POINT('Ctrl Pts',(-85.5900000000001,63.2074283898592,-52.9242386125072));
#54586=CARTESIAN_POINT('Ctrl Pts',(-85.5900000000001,65.8355371052187,-50.6740625107399));
#54587=CARTESIAN_POINT('Ctrl Pts',(-85.5900000000001,69.2652291855737,-46.4949706191462));
#54588=CARTESIAN_POINT('Ctrl Pts',(-85.5900000000003,72.0088947532483,-41.3619333760696));
#54589=CARTESIAN_POINT('Ctrl Pts',(-85.59,73.3905329456488,-36.8072826511288));
#54590=CARTESIAN_POINT('Ctrl Pts',(-85.5899999999999,73.81508077238,-34.0308350004071));
#54591=CARTESIAN_POINT('Ctrl Pts',(-85.5899999999999,73.9088368640223,-33.1606917252932));
#54592=CARTESIAN_POINT('Origin',(-85.59,61.0962221090322,-52.6090816762843));
#54593=CARTESIAN_POINT('',(-85.59,36.8454205811755,-48.9853996542502));
#54594=CARTESIAN_POINT('Origin',(-85.59,36.2795905006212,-50.3745851422034));
#54595=CARTESIAN_POINT('',(-85.59,52.3121016227475,-48.9853996542502));
#54596=CARTESIAN_POINT('Ctrl Pts',(-85.59,36.8454205811755,-48.9853996542502));
#54597=CARTESIAN_POINT('Ctrl Pts',(-85.59,38.0507425038933,-49.4763401417081));
#54598=CARTESIAN_POINT('Ctrl Pts',(-85.5900000000002,40.5938700967861,-50.2396694655963));
#54599=CARTESIAN_POINT('Ctrl Pts',(-85.59,44.5787611019615,-50.6321469729213));
#54600=CARTESIAN_POINT('Ctrl Pts',(-85.5900000000001,48.563652107137,-50.2396694655963));
#54601=CARTESIAN_POINT('Ctrl Pts',(-85.5900000000001,51.1067797000298,-49.4763401417081));
#54602=CARTESIAN_POINT('Ctrl Pts',(-85.59,52.3121016227475,-48.9853996542502));
#54603=CARTESIAN_POINT('Origin',(-85.59,52.8779317033019,-50.3745851422034));
#54604=CARTESIAN_POINT('',(-85.5900000000001,56.5066592279994,-56.980993970528));
#54605=CARTESIAN_POINT('Origin',(-85.59,55.9000854795073,-55.6091090308774));
#54606=CARTESIAN_POINT('Ctrl Pts',(-85.59,32.6508629759236,-56.980993970528));
#54607=CARTESIAN_POINT('Ctrl Pts',(-85.59,32.8626902557763,-57.0746526028663));
#54608=CARTESIAN_POINT('Ctrl Pts',(-85.59,34.8506764348827,-57.9257562386752));
#54609=CARTESIAN_POINT('Ctrl Pts',(-85.5900000000003,38.7864976967653,-59.1196745657386));
#54610=CARTESIAN_POINT('Ctrl Pts',(-85.59,44.5787611019615,-59.6901627171307));
#54611=CARTESIAN_POINT('Ctrl Pts',(-85.5900000000001,50.3710245071578,-59.1196745657386));
#54612=CARTESIAN_POINT('Ctrl Pts',(-85.5900000000001,54.3068457690403,-57.9257562386753));
#54613=CARTESIAN_POINT('Ctrl Pts',(-85.5900000000001,56.2948319481467,-57.0746526028663));
#54614=CARTESIAN_POINT('Ctrl Pts',(-85.5900000000001,56.5066592279994,-56.980993970528));
#54615=CARTESIAN_POINT('',(-85.5900000000001,24.2703224388689,-32.7955273866549));
#54616=CARTESIAN_POINT('Origin',(-85.59,22.7843241379305,-33.));
#54617=CARTESIAN_POINT('',(-85.5900000000001,32.0036528607783,-46.189930240589));
#54618=CARTESIAN_POINT('Ctrl Pts',(-85.5900000000001,24.2703224388689,-32.7955273866549));
#54619=CARTESIAN_POINT('Ctrl Pts',(-85.5900000000001,24.3257980082232,-33.1986943460608));
#54620=CARTESIAN_POINT('Ctrl Pts',(-85.5900000000001,24.6157110848129,-34.9239586938488));
#54621=CARTESIAN_POINT('Ctrl Pts',(-85.5899999999997,25.5171428019148,-37.8955808206585));
#54622=CARTESIAN_POINT('Ctrl Pts',(-85.5900000000001,27.4237578574175,-41.4626067014406));
#54623=CARTESIAN_POINT('Ctrl Pts',(-85.5899999999999,29.6788853182442,-44.2104874631082));
#54624=CARTESIAN_POINT('Ctrl Pts',(-85.5900000000001,31.3290269996959,-45.665888489783));
#54625=CARTESIAN_POINT('Ctrl Pts',(-85.5900000000001,32.0036528607783,-46.189930240589));
#54626=CARTESIAN_POINT('Origin',(-85.59,31.0834721426076,-47.3745261404244));
#54627=CARTESIAN_POINT('',(-85.5900000000001,27.1763562684562,-53.8202275898948));
#54628=CARTESIAN_POINT('Origin',(-85.59,28.0613000948908,-52.6090816762843));
#54629=CARTESIAN_POINT('Ctrl Pts',(-85.59,15.2486853399007,-33.1606917252932));
#54630=CARTESIAN_POINT('Ctrl Pts',(-85.59,15.3424414315431,-34.0308350004071));
#54631=CARTESIAN_POINT('Ctrl Pts',(-85.59,15.7669892582742,-36.8072826511289));
#54632=CARTESIAN_POINT('Ctrl Pts',(-85.5900000000001,17.1486274506748,-41.3619333760696));
#54633=CARTESIAN_POINT('Ctrl Pts',(-85.59,19.8922930183494,-46.4949706191462));
#54634=CARTESIAN_POINT('Ctrl Pts',(-85.5900000000001,23.3219850987043,-50.6740625107399));
#54635=CARTESIAN_POINT('Ctrl Pts',(-85.5900000000001,25.9500938140638,-52.9242386125072));
#54636=CARTESIAN_POINT('Ctrl Pts',(-85.5900000000001,27.1763562684562,-53.8202275898948));
#54637=CARTESIAN_POINT('',(-85.59,32.0036528607784,-13.8100697594109));
#54638=CARTESIAN_POINT('Origin',(-85.59,31.0834721426076,-12.6254738595756));
#54639=CARTESIAN_POINT('',(-85.59,24.2703224388689,-27.2044726133451));
#54640=CARTESIAN_POINT('Ctrl Pts',(-85.59,32.0036528607784,-13.8100697594109));
#54641=CARTESIAN_POINT('Ctrl Pts',(-85.59,31.3290269996959,-14.334111510217));
#54642=CARTESIAN_POINT('Ctrl Pts',(-85.59,29.6788853182442,-15.7895125368918));
#54643=CARTESIAN_POINT('Ctrl Pts',(-85.59,27.4237578574175,-18.5373932985594));
#54644=CARTESIAN_POINT('Ctrl Pts',(-85.5900000000001,25.5171428019148,-22.1044191793415));
#54645=CARTESIAN_POINT('Ctrl Pts',(-85.59,24.6157110848129,-25.0760413061512));
#54646=CARTESIAN_POINT('Ctrl Pts',(-85.59,24.3257980082232,-26.8013056539392));
#54647=CARTESIAN_POINT('Ctrl Pts',(-85.59,24.2703224388689,-27.2044726133451));
#54648=CARTESIAN_POINT('Origin',(-85.59,22.7843241379304,-27.));
#54649=CARTESIAN_POINT('',(-85.5900000000001,27.1763562684563,-6.17977241010519));
#54650=CARTESIAN_POINT('Ctrl Pts',(-85.5900000000001,27.1763562684563,-6.17977241010519));
#54651=CARTESIAN_POINT('Ctrl Pts',(-85.5900000000001,25.9500938140638,-7.07576138749284));
#54652=CARTESIAN_POINT('Ctrl Pts',(-85.5900000000001,23.3219850987044,-9.32593748926008));
#54653=CARTESIAN_POINT('Ctrl Pts',(-85.5900000000001,19.8922930183494,-13.5050293808538));
#54654=CARTESIAN_POINT('Ctrl Pts',(-85.59,17.1486274506748,-18.6380666239304));
#54655=CARTESIAN_POINT('Ctrl Pts',(-85.59,15.7669892582742,-23.1927173488712));
#54656=CARTESIAN_POINT('Ctrl Pts',(-85.5900000000001,15.3424414315431,-25.9691649995929));
#54657=CARTESIAN_POINT('Ctrl Pts',(-85.59,15.2486853399007,-26.8393082747068));
#54658=CARTESIAN_POINT('Origin',(-85.59,28.0613000948908,-7.39091832371568));
#54659=CARTESIAN_POINT('',(-85.59,76.9518771315568,-27.1323759916595));
#54660=CARTESIAN_POINT('Origin',(-85.59,78.4460245797131,-27.));
#54661=CARTESIAN_POINT('Ctrl Pts',(-85.59,76.9518771315568,-27.1323759916595));
#54662=CARTESIAN_POINT('Ctrl Pts',(-85.59,76.8486238665202,-25.9669410775617));
#54663=CARTESIAN_POINT('Ctrl Pts',(-85.5900000000001,76.3805781139122,-22.6983584490168));
#54664=CARTESIAN_POINT('Ctrl Pts',(-85.5899999999998,74.7983998703283,-17.4826157721267));
#54665=CARTESIAN_POINT('Ctrl Pts',(-85.5900000000003,71.775717465263,-11.8275747416186));
#54666=CARTESIAN_POINT('Ctrl Pts',(-85.5900000000001,67.8660024791103,-7.06357324694729));
#54667=CARTESIAN_POINT('Ctrl Pts',(-85.5899999999999,64.7867667693647,-4.47726951084222));
#54668=CARTESIAN_POINT('Ctrl Pts',(-85.5899999999999,63.2487659305948,-3.39775347082817));
#54669=CARTESIAN_POINT('Origin',(-85.59,66.3683162853859,1.74061665201678));
#54670=CARTESIAN_POINT('Origin',(-85.59,82.9621121574678,-27.));
#54671=CARTESIAN_POINT('',(-85.5900000000001,76.9518771315568,-32.8676240083405));
#54672=CARTESIAN_POINT('Ctrl Pts',(-85.5900000000001,63.2487659305946,-56.6022465291719));
#54673=CARTESIAN_POINT('Ctrl Pts',(-85.5900000000001,64.7867667693646,-55.5227304891579));
#54674=CARTESIAN_POINT('Ctrl Pts',(-85.5900000000001,67.8660024791103,-52.9364267530528));
#54675=CARTESIAN_POINT('Ctrl Pts',(-85.59,71.7757174652631,-48.1724252583814));
#54676=CARTESIAN_POINT('Ctrl Pts',(-85.59,74.7983998703283,-42.5173842278733));
#54677=CARTESIAN_POINT('Ctrl Pts',(-85.5900000000002,76.3805781139122,-37.3016415509832));
#54678=CARTESIAN_POINT('Ctrl Pts',(-85.5900000000001,76.8486238665201,-34.0330589224383));
#54679=CARTESIAN_POINT('Ctrl Pts',(-85.5900000000001,76.9518771315568,-32.8676240083405));
#54680=CARTESIAN_POINT('Origin',(-85.59,78.4460245797131,-33.));
#54681=CARTESIAN_POINT('',(-85.5899999999998,84.4575665229983,-33.1166895167565));
#54682=CARTESIAN_POINT('Origin',(-85.59,82.9621122252415,-33.));
#54683=CARTESIAN_POINT('',(-85.5899999999999,67.2171661194344,-62.9773275507524));
#54684=CARTESIAN_POINT('Ctrl Pts',(-85.5899999999999,67.2171661194344,-62.9773275507524));
#54685=CARTESIAN_POINT('Ctrl Pts',(-85.59,68.1585542512634,-62.3311804544817));
#54686=CARTESIAN_POINT('Ctrl Pts',(-85.59,70.120027043277,-60.8582491474625));
#54687=CARTESIAN_POINT('Ctrl Pts',(-85.5899999999998,72.9083073089528,-58.329286199092));
#54688=CARTESIAN_POINT('Ctrl Pts',(-85.5899999999998,75.5496661779346,-55.41704471446));
#54689=CARTESIAN_POINT('Ctrl Pts',(-85.5900000000001,77.8907325893732,-52.2581266162731));
#54690=CARTESIAN_POINT('Ctrl Pts',(-85.5899999999996,79.9131883593013,-48.8865394828812));
#54691=CARTESIAN_POINT('Ctrl Pts',(-85.5899999999997,81.5929974870803,-45.3315997101041));
#54692=CARTESIAN_POINT('Ctrl Pts',(-85.59,82.9188283169055,-41.6302351306666));
#54693=CARTESIAN_POINT('Ctrl Pts',(-85.5899999999998,83.8728260383109,-37.8158880252114));
#54694=CARTESIAN_POINT('Ctrl Pts',(-85.5899999999997,84.2979456369875,-34.9568586727847));
#54695=CARTESIAN_POINT('Ctrl Pts',(-85.5899999999998,84.4366426410887,-33.3848430749953));
#54696=CARTESIAN_POINT('Ctrl Pts',(-85.5899999999998,84.4575665229983,-33.1166895167565));
#54697=CARTESIAN_POINT('Origin',(-85.59,66.3683162666315,-61.7406166195334));
#54698=CARTESIAN_POINT('',(-85.5899999999999,30.8757056257995,-59.4698569539159));
#54699=CARTESIAN_POINT('Origin',(-85.59,30.2431724514241,-60.8299678991386));
#54700=CARTESIAN_POINT('',(-85.5900000000001,58.2818165781235,-59.469856953916));
#54701=CARTESIAN_POINT('Ctrl Pts',(-85.5899999999999,30.8757056257995,-59.4698569539159));
#54702=CARTESIAN_POINT('Ctrl Pts',(-85.59,31.2936434644635,-59.6642231184655));
#54703=CARTESIAN_POINT('Ctrl Pts',(-85.59,33.6635280544172,-60.7056460155572));
#54704=CARTESIAN_POINT('Ctrl Pts',(-85.5900000000002,38.1974539606436,-62.0809974029323));
#54705=CARTESIAN_POINT('Ctrl Pts',(-85.5900000000001,44.5787611019615,-62.7095012985338));
#54706=CARTESIAN_POINT('Ctrl Pts',(-85.59,50.9600682432795,-62.0809974029323));
#54707=CARTESIAN_POINT('Ctrl Pts',(-85.5900000000001,55.4939941495058,-60.7056460155572));
#54708=CARTESIAN_POINT('Ctrl Pts',(-85.5900000000001,57.8638787394595,-59.6642231184655));
#54709=CARTESIAN_POINT('Ctrl Pts',(-85.5900000000001,58.2818165781235,-59.469856953916));
#54710=CARTESIAN_POINT('Origin',(-85.59,58.9143497524989,-60.8299678991386));
#54711=CARTESIAN_POINT('',(-85.5899999999997,61.8185254276963,-66.0944671367427));
#54712=CARTESIAN_POINT('Origin',(-85.59,61.1722799429393,-64.740817708925));
#54713=CARTESIAN_POINT('Ctrl Pts',(-85.5899999999997,27.338996733446,-66.0944672200995));
#54714=CARTESIAN_POINT('Ctrl Pts',(-85.5899999999998,27.9754117244437,-66.3982979628585));
#54715=CARTESIAN_POINT('Ctrl Pts',(-85.59,29.8161761061956,-67.2180577690146));
#54716=CARTESIAN_POINT('Ctrl Pts',(-85.5899999999995,32.9485259712089,-68.3400672149224));
#54717=CARTESIAN_POINT('Ctrl Pts',(-85.5900000000001,36.7628730766652,-69.2940649363253));
#54718=CARTESIAN_POINT('Ctrl Pts',(-85.5899999999996,40.6517737371936,-69.8723198908768));
#54719=CARTESIAN_POINT('Ctrl Pts',(-85.5900000000001,44.5789449552911,-70.0638446084523));
#54720=CARTESIAN_POINT('Ctrl Pts',(-85.5899999999997,48.5059334253501,-69.8723016740253));
#54721=CARTESIAN_POINT('Ctrl Pts',(-85.5900000000001,52.3950097685034,-69.2939932003241));
#54722=CARTESIAN_POINT('Ctrl Pts',(-85.5899999999998,56.2091740834478,-68.3400132644924));
#54723=CARTESIAN_POINT('Ctrl Pts',(-85.5899999999997,59.3415140239783,-67.2179830153801));
#54724=CARTESIAN_POINT('Ctrl Pts',(-85.5899999999997,61.1821104057502,-66.398297896696));
#54725=CARTESIAN_POINT('Ctrl Pts',(-85.5899999999997,61.8185254276963,-66.0944671367427));
#54726=CARTESIAN_POINT('',(-85.59,12.2056450723663,-32.8676240083405));
#54727=CARTESIAN_POINT('Origin',(-85.59,10.7114976242099,-33.));
#54728=CARTESIAN_POINT('',(-85.5899999999998,25.9087562733282,-56.6022465291718));
#54729=CARTESIAN_POINT('Ctrl Pts',(-85.59,12.2056450723663,-32.8676240083405));
#54730=CARTESIAN_POINT('Ctrl Pts',(-85.59,12.3088983374029,-34.0330589224383));
#54731=CARTESIAN_POINT('Ctrl Pts',(-85.59,12.7769440900109,-37.3016415509832));
#54732=CARTESIAN_POINT('Ctrl Pts',(-85.5900000000001,14.3591223335948,-42.5173842278733));
#54733=CARTESIAN_POINT('Ctrl Pts',(-85.5900000000002,17.38180473866,-48.1724252583814));
#54734=CARTESIAN_POINT('Ctrl Pts',(-85.5899999999998,21.2915197248128,-52.9364267530527));
#54735=CARTESIAN_POINT('Ctrl Pts',(-85.5899999999998,24.3707554345583,-55.5227304891578));
#54736=CARTESIAN_POINT('Ctrl Pts',(-85.5899999999998,25.9087562733282,-56.6022465291718));
#54737=CARTESIAN_POINT('Origin',(-85.59,25.0470014756374,-57.8300000340158));
#54738=CARTESIAN_POINT('',(-85.5899999999999,21.9403561483044,-62.9773276342038));
#54739=CARTESIAN_POINT('Origin',(-85.59,22.7892059208967,-61.7406166479301));
#54740=CARTESIAN_POINT('Ctrl Pts',(-85.5899999999999,4.69995574181559,-33.1166894283889));
#54741=CARTESIAN_POINT('Ctrl Pts',(-85.5899999999999,4.72089394220625,-33.3850266919971));
#54742=CARTESIAN_POINT('Ctrl Pts',(-85.5899999999999,4.85960175440013,-34.9570417202001));
#54743=CARTESIAN_POINT('Ctrl Pts',(-85.5899999999997,5.28476790164041,-37.8162486665527));
#54744=CARTESIAN_POINT('Ctrl Pts',(-85.5900000000001,6.23874783746636,-41.6304129814993));
#54745=CARTESIAN_POINT('Ctrl Pts',(-85.5899999999996,7.56466543214173,-45.3319394268853));
#54746=CARTESIAN_POINT('Ctrl Pts',(-85.59,9.2444214554221,-48.8867033911447));
#54747=CARTESIAN_POINT('Ctrl Pts',(-85.5899999999996,11.2669939014917,-52.2584323532902));
#54748=CARTESIAN_POINT('Ctrl Pts',(-85.59,13.6079739302738,-55.4171883812443));
#54749=CARTESIAN_POINT('Ctrl Pts',(-85.59,16.2494749028876,-58.3295462070146));
#54750=CARTESIAN_POINT('Ctrl Pts',(-85.59,19.0376379878578,-60.8583678488589));
#54751=CARTESIAN_POINT('Ctrl Pts',(-85.59,20.9991197888157,-62.3312848007728));
#54752=CARTESIAN_POINT('Ctrl Pts',(-85.5899999999999,21.9403561483044,-62.9773276342038));
#54753=CARTESIAN_POINT('',(-85.5900000000001,25.9087562733283,-3.39775347082815));
#54754=CARTESIAN_POINT('Origin',(-85.59,25.0470014756374,-2.16999996598413));
#54755=CARTESIAN_POINT('',(-85.59,12.2056450723663,-27.1323759916595));
#54756=CARTESIAN_POINT('Ctrl Pts',(-85.5900000000001,25.9087562733283,-3.39775347082815));
#54757=CARTESIAN_POINT('Ctrl Pts',(-85.5900000000001,24.3707554345584,-4.4772695108422));
#54758=CARTESIAN_POINT('Ctrl Pts',(-85.5900000000001,21.2915197248128,-7.06357324694729));
#54759=CARTESIAN_POINT('Ctrl Pts',(-85.59,17.38180473866,-11.8275747416186));
#54760=CARTESIAN_POINT('Ctrl Pts',(-85.5900000000001,14.3591223335948,-17.4826157721267));
#54761=CARTESIAN_POINT('Ctrl Pts',(-85.59,12.7769440900109,-22.6983584490168));
#54762=CARTESIAN_POINT('Ctrl Pts',(-85.59,12.3088983374029,-25.9669410775617));
#54763=CARTESIAN_POINT('Ctrl Pts',(-85.59,12.2056450723663,-27.1323759916595));
#54764=CARTESIAN_POINT('Origin',(-85.59,10.7114976242099,-27.));
#54765=CARTESIAN_POINT('',(-85.59,21.9403560778721,2.9773275404997));
#54766=CARTESIAN_POINT('Ctrl Pts',(-85.59,21.9403560778721,2.9773275404997));
#54767=CARTESIAN_POINT('Ctrl Pts',(-85.59,20.9989679497993,2.33118043675338));
#54768=CARTESIAN_POINT('Ctrl Pts',(-85.5899999999998,19.0374951574427,0.85824915302959));
#54769=CARTESIAN_POINT('Ctrl Pts',(-85.5899999999997,16.2492148952407,-1.67071380306776));
#54770=CARTESIAN_POINT('Ctrl Pts',(-85.5900000000001,13.607856025903,-4.58295528496318));
#54771=CARTESIAN_POINT('Ctrl Pts',(-85.59,11.2667896145647,-7.74187338388924));
#54772=CARTESIAN_POINT('Ctrl Pts',(-85.5899999999998,9.24433384462075,-11.1134605170863));
#54773=CARTESIAN_POINT('Ctrl Pts',(-85.59,7.56452471684338,-14.6684002899082));
#54774=CARTESIAN_POINT('Ctrl Pts',(-85.5899999999997,6.23869388701356,-18.3697648693255));
#54775=CARTESIAN_POINT('Ctrl Pts',(-85.59,5.284696165608,-22.1841119748295));
#54776=CARTESIAN_POINT('Ctrl Pts',(-85.59,4.85957656691687,-25.0431413272591));
#54777=CARTESIAN_POINT('Ctrl Pts',(-85.59,4.72087956281877,-26.6151569250498));
#54778=CARTESIAN_POINT('Ctrl Pts',(-85.59,4.69995568091292,-26.8833104832455));
#54779=CARTESIAN_POINT('Origin',(-85.59,22.789205939653,1.74061661544304));
#54780=CARTESIAN_POINT('Origin',(-85.59,61.1722800421212,4.74081788071294));
#54781=CARTESIAN_POINT('',(-85.59,58.2818165781235,-0.530143046084078));
#54782=CARTESIAN_POINT('Origin',(-85.59,58.914349752499,0.829967899138591));
#54783=CARTESIAN_POINT('Ctrl Pts',(-85.59,58.2818165781235,-0.530143046084078));
#54784=CARTESIAN_POINT('Ctrl Pts',(-85.5900000000001,57.8638787394595,-0.335776881534524));
#54785=CARTESIAN_POINT('Ctrl Pts',(-85.5900000000001,55.4939941495058,0.70564601555715));
#54786=CARTESIAN_POINT('Ctrl Pts',(-85.59,50.9600682432795,2.08099740293233));
#54787=CARTESIAN_POINT('Ctrl Pts',(-85.59,46.7058634824008,2.5));
#54788=CARTESIAN_POINT('Ctrl Pts',(-85.59,44.5787611019615,2.5));
#54789=CARTESIAN_POINT('Origin',(-85.59,30.2431724514241,0.829967899138609));
#54790=CARTESIAN_POINT('Ctrl Pts',(-85.5899999999999,44.5787611019615,10.));
#54791=CARTESIAN_POINT('Ctrl Pts',(-85.5899999999999,43.2696882485426,10.0000072420571));
#54792=CARTESIAN_POINT('Ctrl Pts',(-85.5899999999996,40.651632580144,9.87232797964218));
#54793=CARTESIAN_POINT('Ctrl Pts',(-85.5899999999998,36.7625581228083,9.29399863504675));
#54794=CARTESIAN_POINT('Ctrl Pts',(-85.5899999999998,32.9483479139013,8.34001481829751));
#54795=CARTESIAN_POINT('Ctrl Pts',(-85.5899999999998,29.8160082284385,7.21798291392161));
#54796=CARTESIAN_POINT('Ctrl Pts',(-85.5899999999998,27.9754118813548,6.39829778738203));
#54797=CARTESIAN_POINT('Ctrl Pts',(-85.5899999999998,27.3389968866617,6.09446707403308));
#54798=CARTESIAN_POINT('Ctrl Pts',(-85.5899999999998,27.3389968866527,6.0944670740288));
#54799=CARTESIAN_POINT('Ctrl Pts',(-86.5500000000004,27.3389968866527,6.0944670740288));
#54800=CARTESIAN_POINT('Ctrl Pts',(-85.5899999999998,27.9754118813487,6.39829778737934));
#54801=CARTESIAN_POINT('Ctrl Pts',(-86.5500000000004,27.9754118813487,6.39829778737934));
#54802=CARTESIAN_POINT('Ctrl Pts',(-85.5899999999998,29.8160082284354,7.21798291392049));
#54803=CARTESIAN_POINT('Ctrl Pts',(-86.5500000000004,29.8160082284354,7.21798291392049));
#54804=CARTESIAN_POINT('Ctrl Pts',(-85.5899999999998,32.9483479139013,8.34001481829751));
#54805=CARTESIAN_POINT('Ctrl Pts',(-86.5500000000004,32.9483479139013,8.34001481829751));
#54806=CARTESIAN_POINT('Ctrl Pts',(-85.5899999999998,36.7625581228083,9.29399863504675));
#54807=CARTESIAN_POINT('Ctrl Pts',(-86.5500000000004,36.7625581228083,9.29399863504675));
#54808=CARTESIAN_POINT('Ctrl Pts',(-85.5899999999996,40.651632580144,9.87232797964218));
#54809=CARTESIAN_POINT('Ctrl Pts',(-86.5500000000002,40.651632580144,9.87232797964218));
#54810=CARTESIAN_POINT('Ctrl Pts',(-85.59,43.2696882485426,10.0000072420571));
#54811=CARTESIAN_POINT('Ctrl Pts',(-86.5500000000005,43.2696882485426,10.0000072420571));
#54812=CARTESIAN_POINT('Ctrl Pts',(-85.5899999999998,44.5787611019615,10.));
#54813=CARTESIAN_POINT('Ctrl Pts',(-86.5500000000004,44.5787611019615,10.));
#54814=CARTESIAN_POINT('Ctrl Pts',(-86.3899999999999,44.5787611019615,10.));
#54815=CARTESIAN_POINT('Ctrl Pts',(-86.3899999999999,43.2696882485426,10.0000072420571));
#54816=CARTESIAN_POINT('Ctrl Pts',(-86.3899999999996,40.6516325801439,9.87232797964218));
#54817=CARTESIAN_POINT('Ctrl Pts',(-86.3899999999999,36.7625581228083,9.29399863504675));
#54818=CARTESIAN_POINT('Ctrl Pts',(-86.3899999999999,32.9483479139013,8.34001481829751));
#54819=CARTESIAN_POINT('Ctrl Pts',(-86.3899999999999,29.8160082284385,7.21798291392161));
#54820=CARTESIAN_POINT('Ctrl Pts',(-86.3899999999999,27.9754118813548,6.39829778738203));
#54821=CARTESIAN_POINT('Ctrl Pts',(-86.3899999999999,27.3389968866617,6.09446707403308));
#54822=CARTESIAN_POINT('Origin',(913.61,45.8777992076386,-29.25));
#54823=CARTESIAN_POINT('',(-86.39,41.3708603409714,-21.4437528963263));
#54824=CARTESIAN_POINT('',(-86.39,45.8777992076382,-29.25));
#54825=CARTESIAN_POINT('',(-86.3899999999997,41.3708603409714,-21.4437528963263));
#54826=CARTESIAN_POINT('Ctrl Pts',(-85.59,4.69995568091346,-26.8833104832386));
#54827=CARTESIAN_POINT('Ctrl Pts',(-86.5500000000002,4.69995568091346,-26.8833104832386));
#54828=CARTESIAN_POINT('Ctrl Pts',(-85.59,4.72087956281917,-26.6151569250452));
#54829=CARTESIAN_POINT('Ctrl Pts',(-86.5500000000002,4.72087956281917,-26.6151569250452));
#54830=CARTESIAN_POINT('Ctrl Pts',(-85.59,4.85957656691721,-25.0431413272568));
#54831=CARTESIAN_POINT('Ctrl Pts',(-86.5500000000003,4.85957656691721,-25.0431413272568));
#54832=CARTESIAN_POINT('Ctrl Pts',(-85.59,5.284696165608,-22.1841119748295));
#54833=CARTESIAN_POINT('Ctrl Pts',(-86.5500000000002,5.284696165608,-22.1841119748295));
#54834=CARTESIAN_POINT('Ctrl Pts',(-85.5899999999997,6.23869388701356,-18.3697648693255));
#54835=CARTESIAN_POINT('Ctrl Pts',(-86.55,6.23869388701356,-18.3697648693255));
#54836=CARTESIAN_POINT('Ctrl Pts',(-85.59,7.56452471684338,-14.6684002899082));
#54837=CARTESIAN_POINT('Ctrl Pts',(-86.5500000000002,7.56452471684338,-14.6684002899082));
#54838=CARTESIAN_POINT('Ctrl Pts',(-85.5899999999998,9.24433384462075,-11.1134605170863));
#54839=CARTESIAN_POINT('Ctrl Pts',(-86.5500000000001,9.24433384462075,-11.1134605170863));
#54840=CARTESIAN_POINT('Ctrl Pts',(-85.59,11.2667896145647,-7.74187338388924));
#54841=CARTESIAN_POINT('Ctrl Pts',(-86.5500000000002,11.2667896145647,-7.74187338388924));
#54842=CARTESIAN_POINT('Ctrl Pts',(-85.5900000000001,13.607856025903,-4.58295528496318));
#54843=CARTESIAN_POINT('Ctrl Pts',(-86.5500000000003,13.607856025903,-4.58295528496318));
#54844=CARTESIAN_POINT('Ctrl Pts',(-85.5899999999997,16.2492148952407,-1.67071380306776));
#54845=CARTESIAN_POINT('Ctrl Pts',(-86.55,16.2492148952407,-1.67071380306776));
#54846=CARTESIAN_POINT('Ctrl Pts',(-85.5899999999998,19.0374951574414,0.858249153028345));
#54847=CARTESIAN_POINT('Ctrl Pts',(-86.5500000000001,19.0374951574414,0.858249153028345));
#54848=CARTESIAN_POINT('Ctrl Pts',(-85.59,20.9989679497964,2.33118043675116));
#54849=CARTESIAN_POINT('Ctrl Pts',(-86.5500000000002,20.9989679497964,2.33118043675116));
#54850=CARTESIAN_POINT('Ctrl Pts',(-85.59,21.9403560778675,2.97732754049656));
#54851=CARTESIAN_POINT('Ctrl Pts',(-86.5500000000002,21.9403560778675,2.97732754049656));
#54852=CARTESIAN_POINT('',(-86.39,21.9403560778721,2.9773275404997));
#54853=CARTESIAN_POINT('Ctrl Pts',(-86.39,21.9403560778721,2.9773275404997));
#54854=CARTESIAN_POINT('Ctrl Pts',(-86.39,20.9989679497993,2.33118043675338));
#54855=CARTESIAN_POINT('Ctrl Pts',(-86.3899999999999,19.0374951574427,0.85824915302959));
#54856=CARTESIAN_POINT('Ctrl Pts',(-86.3899999999997,16.2492148952407,-1.67071380306776));
#54857=CARTESIAN_POINT('Ctrl Pts',(-86.3900000000001,13.607856025903,-4.58295528496318));
#54858=CARTESIAN_POINT('Ctrl Pts',(-86.39,11.2667896145647,-7.74187338388924));
#54859=CARTESIAN_POINT('Ctrl Pts',(-86.3899999999999,9.24433384462075,-11.1134605170863));
#54860=CARTESIAN_POINT('Ctrl Pts',(-86.39,7.56452471684338,-14.6684002899082));
#54861=CARTESIAN_POINT('Ctrl Pts',(-86.3899999999997,6.23869388701356,-18.3697648693255));
#54862=CARTESIAN_POINT('Ctrl Pts',(-86.39,5.284696165608,-22.1841119748295));
#54863=CARTESIAN_POINT('Ctrl Pts',(-86.39,4.85957656691687,-25.0431413272591));
#54864=CARTESIAN_POINT('Ctrl Pts',(-86.39,4.72087956281877,-26.6151569250498));
#54865=CARTESIAN_POINT('Ctrl Pts',(-86.39,4.69995568091292,-26.8833104832455));
#54866=CARTESIAN_POINT('',(-86.39,21.9403560778721,2.9773275404997));
#54867=CARTESIAN_POINT('Ctrl Pts',(-85.5899999999998,21.9403561482997,-62.9773276342005));
#54868=CARTESIAN_POINT('Ctrl Pts',(-86.55,21.9403561482997,-62.9773276342005));
#54869=CARTESIAN_POINT('Ctrl Pts',(-85.5899999999998,20.9991197888127,-62.3312848007705));
#54870=CARTESIAN_POINT('Ctrl Pts',(-86.55,20.9991197888127,-62.3312848007705));
#54871=CARTESIAN_POINT('Ctrl Pts',(-85.5899999999998,19.0376379878564,-60.8583678488576));
#54872=CARTESIAN_POINT('Ctrl Pts',(-86.55,19.0376379878564,-60.8583678488576));
#54873=CARTESIAN_POINT('Ctrl Pts',(-85.5899999999998,16.2494749028876,-58.3295462070146));
#54874=CARTESIAN_POINT('Ctrl Pts',(-86.55,16.2494749028876,-58.3295462070146));
#54875=CARTESIAN_POINT('Ctrl Pts',(-85.5899999999998,13.6079739302738,-55.4171883812443));
#54876=CARTESIAN_POINT('Ctrl Pts',(-86.55,13.6079739302738,-55.4171883812443));
#54877=CARTESIAN_POINT('Ctrl Pts',(-85.5899999999995,11.2669939014917,-52.2584323532902));
#54878=CARTESIAN_POINT('Ctrl Pts',(-86.5499999999997,11.2669939014917,-52.2584323532902));
#54879=CARTESIAN_POINT('Ctrl Pts',(-85.5899999999998,9.2444214554221,-48.8867033911447));
#54880=CARTESIAN_POINT('Ctrl Pts',(-86.55,9.2444214554221,-48.8867033911447));
#54881=CARTESIAN_POINT('Ctrl Pts',(-85.5899999999995,7.56466543214173,-45.3319394268853));
#54882=CARTESIAN_POINT('Ctrl Pts',(-86.5499999999997,7.56466543214173,-45.3319394268853));
#54883=CARTESIAN_POINT('Ctrl Pts',(-85.59,6.23874783746636,-41.6304129814993));
#54884=CARTESIAN_POINT('Ctrl Pts',(-86.5500000000002,6.23874783746636,-41.6304129814993));
#54885=CARTESIAN_POINT('Ctrl Pts',(-85.5899999999996,5.28476790164041,-37.8162486665527));
#54886=CARTESIAN_POINT('Ctrl Pts',(-86.5499999999998,5.28476790164041,-37.8162486665527));
#54887=CARTESIAN_POINT('Ctrl Pts',(-85.5899999999998,4.85960175440047,-34.9570417202024));
#54888=CARTESIAN_POINT('Ctrl Pts',(-86.55,4.85960175440047,-34.9570417202024));
#54889=CARTESIAN_POINT('Ctrl Pts',(-85.5899999999997,4.72089394220665,-33.3850266920016));
#54890=CARTESIAN_POINT('Ctrl Pts',(-86.55,4.72089394220665,-33.3850266920016));
#54891=CARTESIAN_POINT('Ctrl Pts',(-85.5899999999997,4.69995574181612,-33.1166894283958));
#54892=CARTESIAN_POINT('Ctrl Pts',(-86.55,4.69995574181612,-33.1166894283958));
#54893=CARTESIAN_POINT('',(-86.3899999999999,21.9403561483044,-62.9773276342038));
#54894=CARTESIAN_POINT('',(-85.5899999999997,21.9403561483044,-62.9773276342038));
#54895=CARTESIAN_POINT('Ctrl Pts',(-86.3899999999999,4.69995574181559,-33.1166894283889));
#54896=CARTESIAN_POINT('Ctrl Pts',(-86.3899999999999,4.72089394220625,-33.3850266919971));
#54897=CARTESIAN_POINT('Ctrl Pts',(-86.3899999999999,4.85960175440013,-34.9570417202001));
#54898=CARTESIAN_POINT('Ctrl Pts',(-86.3899999999997,5.28476790164041,-37.8162486665527));
#54899=CARTESIAN_POINT('Ctrl Pts',(-86.3900000000001,6.23874783746636,-41.6304129814993));
#54900=CARTESIAN_POINT('Ctrl Pts',(-86.3899999999996,7.56466543214173,-45.3319394268853));
#54901=CARTESIAN_POINT('Ctrl Pts',(-86.39,9.2444214554221,-48.8867033911447));
#54902=CARTESIAN_POINT('Ctrl Pts',(-86.3899999999996,11.2669939014917,-52.2584323532902));
#54903=CARTESIAN_POINT('Ctrl Pts',(-86.39,13.6079739302738,-55.4171883812443));
#54904=CARTESIAN_POINT('Ctrl Pts',(-86.39,16.2494749028876,-58.3295462070146));
#54905=CARTESIAN_POINT('Ctrl Pts',(-86.39,19.0376379878578,-60.8583678488589));
#54906=CARTESIAN_POINT('Ctrl Pts',(-86.39,20.9991197888157,-62.3312848007728));
#54907=CARTESIAN_POINT('Ctrl Pts',(-86.3899999999999,21.9403561483044,-62.9773276342038));
#54908=CARTESIAN_POINT('Ctrl Pts',(-85.5899999999997,61.8185254277052,-66.0944671367384));
#54909=CARTESIAN_POINT('Ctrl Pts',(-86.55,61.8185254277052,-66.0944671367384));
#54910=CARTESIAN_POINT('Ctrl Pts',(-85.5899999999997,61.1821104057562,-66.3982978966933));
#54911=CARTESIAN_POINT('Ctrl Pts',(-86.55,61.1821104057562,-66.3982978966933));
#54912=CARTESIAN_POINT('Ctrl Pts',(-85.5899999999997,59.3415140239815,-67.217983015379));
#54913=CARTESIAN_POINT('Ctrl Pts',(-86.55,59.3415140239815,-67.217983015379));
#54914=CARTESIAN_POINT('Ctrl Pts',(-85.5899999999998,56.2091740834478,-68.3400132644924));
#54915=CARTESIAN_POINT('Ctrl Pts',(-86.5500000000001,56.2091740834478,-68.3400132644924));
#54916=CARTESIAN_POINT('Ctrl Pts',(-85.5900000000001,52.3950097685034,-69.2939932003241));
#54917=CARTESIAN_POINT('Ctrl Pts',(-86.5500000000004,52.3950097685034,-69.2939932003241));
#54918=CARTESIAN_POINT('Ctrl Pts',(-85.5899999999997,48.5059334253501,-69.8723016740253));
#54919=CARTESIAN_POINT('Ctrl Pts',(-86.55,48.5059334253501,-69.8723016740253));
#54920=CARTESIAN_POINT('Ctrl Pts',(-85.5900000000001,44.5789449552911,-70.0638446084523));
#54921=CARTESIAN_POINT('Ctrl Pts',(-86.5500000000004,44.5789449552911,-70.0638446084523));
#54922=CARTESIAN_POINT('Ctrl Pts',(-85.5899999999996,40.6517737371936,-69.8723198908768));
#54923=CARTESIAN_POINT('Ctrl Pts',(-86.5499999999999,40.6517737371936,-69.8723198908768));
#54924=CARTESIAN_POINT('Ctrl Pts',(-85.5900000000001,36.7628730766652,-69.2940649363253));
#54925=CARTESIAN_POINT('Ctrl Pts',(-86.5500000000004,36.7628730766652,-69.2940649363253));
#54926=CARTESIAN_POINT('Ctrl Pts',(-85.5899999999995,32.9485259712089,-68.3400672149224));
#54927=CARTESIAN_POINT('Ctrl Pts',(-86.5499999999998,32.9485259712089,-68.3400672149224));
#54928=CARTESIAN_POINT('Ctrl Pts',(-85.59,29.8161761061925,-67.2180577690135));
#54929=CARTESIAN_POINT('Ctrl Pts',(-86.5500000000003,29.8161761061925,-67.2180577690135));
#54930=CARTESIAN_POINT('Ctrl Pts',(-85.5899999999998,27.9754117244376,-66.3982979628559));
#54931=CARTESIAN_POINT('Ctrl Pts',(-86.5500000000001,27.9754117244376,-66.3982979628559));
#54932=CARTESIAN_POINT('Ctrl Pts',(-85.5899999999998,27.3389967334371,-66.0944672200952));
#54933=CARTESIAN_POINT('Ctrl Pts',(-86.5500000000001,27.3389967334371,-66.0944672200952));
#54934=CARTESIAN_POINT('',(-86.3899999999997,61.8185254276963,-66.0944671367427));
#54935=CARTESIAN_POINT('',(-85.5899999999998,61.8185254276963,-66.0944671367427));
#54936=CARTESIAN_POINT('Ctrl Pts',(-86.3899999999998,27.338996733446,-66.0944672200995));
#54937=CARTESIAN_POINT('Ctrl Pts',(-86.3899999999998,27.9754117244437,-66.3982979628585));
#54938=CARTESIAN_POINT('Ctrl Pts',(-86.39,29.8161761061956,-67.2180577690146));
#54939=CARTESIAN_POINT('Ctrl Pts',(-86.3899999999995,32.9485259712089,-68.3400672149224));
#54940=CARTESIAN_POINT('Ctrl Pts',(-86.3900000000001,36.7628730766652,-69.2940649363253));
#54941=CARTESIAN_POINT('Ctrl Pts',(-86.3899999999996,40.6517737371936,-69.8723198908768));
#54942=CARTESIAN_POINT('Ctrl Pts',(-86.3900000000001,44.5789449552911,-70.0638446084523));
#54943=CARTESIAN_POINT('Ctrl Pts',(-86.3899999999997,48.50593342535,-69.8723016740253));
#54944=CARTESIAN_POINT('Ctrl Pts',(-86.3900000000001,52.3950097685034,-69.2939932003241));
#54945=CARTESIAN_POINT('Ctrl Pts',(-86.3899999999999,56.2091740834477,-68.3400132644924));
#54946=CARTESIAN_POINT('Ctrl Pts',(-86.3899999999998,59.3415140239783,-67.2179830153801));
#54947=CARTESIAN_POINT('Ctrl Pts',(-86.3899999999998,61.1821104057502,-66.398297896696));
#54948=CARTESIAN_POINT('Ctrl Pts',(-86.3899999999997,61.8185254276963,-66.0944671367427));
#54949=CARTESIAN_POINT('Origin',(-84.39,91.,80.));
#54950=CARTESIAN_POINT('',(-84.39,91.,75.));
#54951=CARTESIAN_POINT('',(-84.39,91.,-75.));
#54952=CARTESIAN_POINT('',(-84.39,91.,80.));
#54953=CARTESIAN_POINT('',(-84.39,86.,-80.));
#54954=CARTESIAN_POINT('',(-84.3900000000001,168.5,2.50000000000003));
#54955=CARTESIAN_POINT('',(-84.39,-1.84247779607695,-80.));
#54956=CARTESIAN_POINT('',(-84.39,91.,-80.));
#54957=CARTESIAN_POINT('',(-84.39,-1.84247779607695,-70.));
#54958=CARTESIAN_POINT('',(-84.39,-1.84247779607695,80.));
#54959=CARTESIAN_POINT('',(-84.39,-2.4,-68.8330657242578));
#54960=CARTESIAN_POINT('Origin',(-84.39,-3.34247779607695,-70.));
#54961=CARTESIAN_POINT('',(-84.39,-2.40000000000001,68.8330657242578));
#54962=CARTESIAN_POINT('',(-84.39,-2.40000000000001,80.));
#54963=CARTESIAN_POINT('',(-84.39,-1.84247779607695,70.));
#54964=CARTESIAN_POINT('Origin',(-84.39,-3.34247779607695,70.));
#54965=CARTESIAN_POINT('',(-84.39,-1.84247779607695,80.));
#54966=CARTESIAN_POINT('',(-84.39,-1.84247779607695,80.));
#54967=CARTESIAN_POINT('',(-84.39,86.,80.));
#54968=CARTESIAN_POINT('',(-84.39,91.,80.));
#54969=CARTESIAN_POINT('',(-84.39,88.5,77.5));
#54970=CARTESIAN_POINT('',(-84.39,64.417,65.));
#54971=CARTESIAN_POINT('',(-84.39,64.417,75.));
#54972=CARTESIAN_POINT('',(-84.39,64.417,65.));
#54973=CARTESIAN_POINT('',(-84.39,78.6669999999999,65.));
#54974=CARTESIAN_POINT('',(-84.39,64.6169999999999,65.));
#54975=CARTESIAN_POINT('',(-84.39,78.667,75.));
#54976=CARTESIAN_POINT('',(-84.39,78.667,75.));
#54977=CARTESIAN_POINT('',(-84.39,78.467,75.));
#54978=CARTESIAN_POINT('',(-84.39,76.,47.667));
#54979=CARTESIAN_POINT('',(-84.39,78.667,45.));
#54980=CARTESIAN_POINT('Origin',(-84.39,76.,45.));
#54981=CARTESIAN_POINT('',(-84.39,70.792807570849,47.667));
#54982=CARTESIAN_POINT('',(-84.39,70.792807570849,47.667));
#54983=CARTESIAN_POINT('',(-84.39,68.9069537854245,46.8858537854245));
#54984=CARTESIAN_POINT('Origin',(-84.39,70.792807570849,45.));
#54985=CARTESIAN_POINT('',(-84.39,66.0242462145755,44.0031462145755));
#54986=CARTESIAN_POINT('',(-84.39,66.0242462145755,44.0031462145755));
#54987=CARTESIAN_POINT('',(-84.39,65.2431,42.117292429151));
#54988=CARTESIAN_POINT('Origin',(-84.39,67.9101,42.117292429151));
#54989=CARTESIAN_POINT('',(-84.39,65.2431,34.547707570849));
#54990=CARTESIAN_POINT('',(-84.39,65.2431,34.547707570849));
#54991=CARTESIAN_POINT('',(-84.39,66.0242462145755,32.6618537854245));
#54992=CARTESIAN_POINT('Origin',(-84.39,67.9101,34.547707570849));
#54993=CARTESIAN_POINT('',(-84.39,68.9069537854245,29.7791462145755));
#54994=CARTESIAN_POINT('',(-84.39,68.9069537854245,29.7791462145755));
#54995=CARTESIAN_POINT('',(-84.39,70.792807570849,28.998));
#54996=CARTESIAN_POINT('Origin',(-84.39,70.792807570849,31.665));
#54997=CARTESIAN_POINT('',(-84.39,76.,28.998));
#54998=CARTESIAN_POINT('',(-84.39,76.,28.998));
#54999=CARTESIAN_POINT('',(-84.39,78.667,31.665));
#55000=CARTESIAN_POINT('Origin',(-84.39,76.,31.665));
#55001=CARTESIAN_POINT('',(-84.39,78.667,45.));
#55002=CARTESIAN_POINT('Origin',(-83.59,91.,80.));
#55003=CARTESIAN_POINT('',(-83.59,-1.84247779607695,-80.));
#55004=CARTESIAN_POINT('',(-83.59,86.,-80.));
#55005=CARTESIAN_POINT('',(-83.59,91.,-80.));
#55006=CARTESIAN_POINT('',(-83.59,91.,-75.));
#55007=CARTESIAN_POINT('',(-83.59,86.,-80.));
#55008=CARTESIAN_POINT('',(-83.59,91.,75.));
#55009=CARTESIAN_POINT('',(-83.59,91.,80.));
#55010=CARTESIAN_POINT('',(-83.59,86.,80.));
#55011=CARTESIAN_POINT('',(-83.59,91.,75.));
#55012=CARTESIAN_POINT('',(-83.59,-1.84247779607695,80.));
#55013=CARTESIAN_POINT('',(-83.59,91.,80.));
#55014=CARTESIAN_POINT('',(-83.59,-1.84247779607695,70.));
#55015=CARTESIAN_POINT('',(-83.59,-1.84247779607695,70.));
#55016=CARTESIAN_POINT('',(-83.59,-2.40000000000001,68.8330657242578));
#55017=CARTESIAN_POINT('Origin',(-83.59,-3.34247779607695,70.));
#55018=CARTESIAN_POINT('',(-83.59,-2.40000000000001,-68.8330657242578));
#55019=CARTESIAN_POINT('',(-83.59,-2.40000000000001,80.));
#55020=CARTESIAN_POINT('',(-83.59,-1.84247779607695,-70.));
#55021=CARTESIAN_POINT('Origin',(-83.59,-3.34247779607695,-70.));
#55022=CARTESIAN_POINT('',(-83.59,-1.84247779607695,-70.));
#55023=CARTESIAN_POINT('',(-83.59,78.6669999999999,65.));
#55024=CARTESIAN_POINT('',(-83.59,64.417,65.));
#55025=CARTESIAN_POINT('',(-83.59,91.,65.));
#55026=CARTESIAN_POINT('',(-83.59,64.417,75.));
#55027=CARTESIAN_POINT('',(-83.59,64.417,80.0000000000001));
#55028=CARTESIAN_POINT('',(-83.59,78.667,75.));
#55029=CARTESIAN_POINT('',(-83.59,91.,75.));
#55030=CARTESIAN_POINT('',(-83.59,78.667,80.0000000000001));
#55031=CARTESIAN_POINT('',(-83.59,70.792807570849,47.667));
#55032=CARTESIAN_POINT('',(-83.59,76.,47.667));
#55033=CARTESIAN_POINT('',(-83.59,91.,47.667));
#55034=CARTESIAN_POINT('',(-83.59,78.667,45.));
#55035=CARTESIAN_POINT('Origin',(-83.59,76.,45.));
#55036=CARTESIAN_POINT('',(-83.59,78.667,31.665));
#55037=CARTESIAN_POINT('',(-83.59,78.667,80.));
#55038=CARTESIAN_POINT('',(-83.59,76.,28.998));
#55039=CARTESIAN_POINT('Origin',(-83.59,76.,31.665));
#55040=CARTESIAN_POINT('',(-83.59,70.792807570849,28.998));
#55041=CARTESIAN_POINT('',(-83.59,91.0000000000001,28.998));
#55042=CARTESIAN_POINT('',(-83.59,68.9069537854245,29.7791462145755));
#55043=CARTESIAN_POINT('Origin',(-83.59,70.792807570849,31.665));
#55044=CARTESIAN_POINT('',(-83.59,66.0242462145755,32.6618537854245));
#55045=CARTESIAN_POINT('',(-83.59,54.8430500000001,43.8430499999998));
#55046=CARTESIAN_POINT('',(-83.59,65.2431,34.547707570849));
#55047=CARTESIAN_POINT('Origin',(-83.59,67.9101,34.547707570849));
#55048=CARTESIAN_POINT('',(-83.59,65.2431,42.117292429151));
#55049=CARTESIAN_POINT('',(-83.59,65.2431000000001,80.0000000000001));
#55050=CARTESIAN_POINT('',(-83.59,66.0242462145755,44.0031462145755));
#55051=CARTESIAN_POINT('Origin',(-83.59,67.9101,42.117292429151));
#55052=CARTESIAN_POINT('',(-83.59,68.9069537854245,46.8858537854245));
#55053=CARTESIAN_POINT('',(-83.59,96.5105500000001,74.4894499999998));
#55054=CARTESIAN_POINT('Origin',(-83.59,70.792807570849,45.));
#55055=CARTESIAN_POINT('Origin',(69.9524777960769,-13.2,70.));
#55056=CARTESIAN_POINT('',(69.01,-3.24056285356845,68.8330657242578));
#55057=CARTESIAN_POINT('',(69.01,-3.2,68.8330657242578));
#55058=CARTESIAN_POINT('',(68.4524777960769,-13.2,70.));
#55059=CARTESIAN_POINT('',(69.01,-3.2,68.8330657242578));
#55060=CARTESIAN_POINT('Origin',(68.4524777960769,-13.2,70.));
#55061=CARTESIAN_POINT('Origin',(69.9524777960769,-13.2,-70.));
#55062=CARTESIAN_POINT('',(69.01,-3.36366990003729,-68.8330657242578));
#55063=CARTESIAN_POINT('',(69.01,-4.,-68.8330657242578));
#55064=CARTESIAN_POINT('',(68.4524777960769,-13.2,-70.));
#55065=CARTESIAN_POINT('',(69.01,-4.,-68.8330657242578));
#55066=CARTESIAN_POINT('Origin',(68.4524777960769,-13.2,-70.));
#55067=CARTESIAN_POINT('Origin',(-83.7324777960769,-13.2,-70.));
#55068=CARTESIAN_POINT('',(-82.79,-3.24056285356836,-68.8330657242578));
#55069=CARTESIAN_POINT('',(-82.79,-3.2,-68.8330657242578));
#55070=CARTESIAN_POINT('',(-82.2324777960769,-13.2,-70.));
#55071=CARTESIAN_POINT('',(-82.79,-3.2,-68.8330657242578));
#55072=CARTESIAN_POINT('Origin',(-82.2324777960769,-13.2,-70.));
#55073=CARTESIAN_POINT('Origin',(-83.7324777960769,-13.2,70.));
#55074=CARTESIAN_POINT('',(-82.79,-3.36366990003701,68.8330657242578));
#55075=CARTESIAN_POINT('',(-82.79,-4.,68.8330657242578));
#55076=CARTESIAN_POINT('',(-82.2324777960769,-13.2,70.));
#55077=CARTESIAN_POINT('',(-82.79,-4.,68.8330657242578));
#55078=CARTESIAN_POINT('Origin',(-82.2324777960769,-13.2,70.));
#55079=CARTESIAN_POINT('Ctrl Pts',(-82.79,-4.,68.8330657242578));
#55080=CARTESIAN_POINT('Ctrl Pts',(-83.0279413156566,-4.,68.7173110465017));
#55081=CARTESIAN_POINT('Ctrl Pts',(-83.2497639817604,-3.94677923887688,
68.6312955463483));
#55082=CARTESIAN_POINT('Ctrl Pts',(-83.5368725214139,-3.81885822756997,
68.5460136539507));
#55083=CARTESIAN_POINT('Ctrl Pts',(-83.6251250918969,-3.76825636386172,
68.5249247721554));
#55084=CARTESIAN_POINT('Ctrl Pts',(-83.7454145055013,-3.6843570265968,68.5042990729681));
#55085=CARTESIAN_POINT('Ctrl Pts',(-83.783508253167,-3.65505504190423,68.4992584438234));
#55086=CARTESIAN_POINT('Ctrl Pts',(-83.8376288357695,-3.60955747043879,
68.4944494059826));
#55087=CARTESIAN_POINT('Ctrl Pts',(-83.8551663111009,-3.59413389138064,
68.4933050443484));
#55088=CARTESIAN_POINT('Ctrl Pts',(-83.8807216791802,-3.57066646564186,
68.4922764783663));
#55089=CARTESIAN_POINT('Ctrl Pts',(-83.8891150287393,-3.56278862689171,
68.4920482857838));
#55090=CARTESIAN_POINT('Ctrl Pts',(-83.9015180955293,-3.55089544816994,
68.4918779910273));
#55091=CARTESIAN_POINT('Ctrl Pts',(-83.9056212935433,-3.54691831714174,
68.4918498917946));
#55092=CARTESIAN_POINT('Ctrl Pts',(-83.9137655150753,-3.53893966650135,
68.4918510247018));
#55093=CARTESIAN_POINT('Ctrl Pts',(-83.918406027794,-3.53433818508778,68.4918889124519));
#55094=CARTESIAN_POINT('Ctrl Pts',(-84.0309533559687,-3.4217021285415,68.4935139055717));
#55095=CARTESIAN_POINT('Ctrl Pts',(-84.1449446474647,-3.27632522988999,
68.5227290784896));
#55096=CARTESIAN_POINT('Ctrl Pts',(-84.3247858753762,-2.89825016104428,
68.636438268353));
#55097=CARTESIAN_POINT('Ctrl Pts',(-84.39,-2.66511752285694,68.7205706579524));
#55098=CARTESIAN_POINT('Ctrl Pts',(-84.39,-2.4,68.8330657242578));
#55099=CARTESIAN_POINT('Ctrl Pts',(-82.79,-3.2,68.8330657242578));
#55100=CARTESIAN_POINT('Ctrl Pts',(-82.9088984009137,-3.2,68.7173813501885));
#55101=CARTESIAN_POINT('Ctrl Pts',(-83.0198819908802,-3.17338961943844,
68.6312955463483));
#55102=CARTESIAN_POINT('Ctrl Pts',(-83.163436260707,-3.10942911378499,68.5460136539507));
#55103=CARTESIAN_POINT('Ctrl Pts',(-83.2075625459484,-3.08412818193086,
68.5249247721554));
#55104=CARTESIAN_POINT('Ctrl Pts',(-83.2677072527507,-3.0421785132984,68.5042990729681));
#55105=CARTESIAN_POINT('Ctrl Pts',(-83.2867541265835,-3.02752752095212,
68.4992584438234));
#55106=CARTESIAN_POINT('Ctrl Pts',(-83.3138144178847,-3.0047787352194,68.4944494059826));
#55107=CARTESIAN_POINT('Ctrl Pts',(-83.3225831555504,-2.99706694569032,
68.4933050443484));
#55108=CARTESIAN_POINT('Ctrl Pts',(-83.3353608395901,-2.98533323282093,
68.4922764783663));
#55109=CARTESIAN_POINT('Ctrl Pts',(-83.3395575143696,-2.98139431344585,
68.4920482857838));
#55110=CARTESIAN_POINT('Ctrl Pts',(-83.3457590477646,-2.97544772408497,
68.4918779910273));
#55111=CARTESIAN_POINT('Ctrl Pts',(-83.3478106467717,-2.97345915857087,
68.4918498917946));
#55112=CARTESIAN_POINT('Ctrl Pts',(-83.3518827575376,-2.96946983325068,
68.4918510247018));
#55113=CARTESIAN_POINT('Ctrl Pts',(-83.354203013897,-2.96716909254389,68.4918889124519));
#55114=CARTESIAN_POINT('Ctrl Pts',(-83.4104766779843,-2.91085106427075,
68.4935139055717));
#55115=CARTESIAN_POINT('Ctrl Pts',(-83.4674723237323,-2.838162614945,68.5227290784896));
#55116=CARTESIAN_POINT('Ctrl Pts',(-83.5573929376881,-2.64912508052214,
68.636438268353));
#55117=CARTESIAN_POINT('Ctrl Pts',(-83.59,-2.53242495718233,68.7206842099906));
#55118=CARTESIAN_POINT('Ctrl Pts',(-83.59,-2.4,68.8330657242578));
#55119=CARTESIAN_POINT('Ctrl Pts',(-82.79,-3.2,68.8330657242578));
#55120=CARTESIAN_POINT('Ctrl Pts',(-82.9088984009137,-3.2,68.7173813501885));
#55121=CARTESIAN_POINT('Ctrl Pts',(-83.0198819908802,-3.17338961943844,
68.6312955463483));
#55122=CARTESIAN_POINT('Ctrl Pts',(-83.163436260707,-3.10942911378499,68.5460136539507));
#55123=CARTESIAN_POINT('Ctrl Pts',(-83.2075625459484,-3.08412818193086,
68.5249247721554));
#55124=CARTESIAN_POINT('Ctrl Pts',(-83.2677072527507,-3.0421785132984,68.5042990729681));
#55125=CARTESIAN_POINT('Ctrl Pts',(-83.2867541265835,-3.02752752095212,
68.4992584438234));
#55126=CARTESIAN_POINT('Ctrl Pts',(-83.3138144178847,-3.0047787352194,68.4944494059826));
#55127=CARTESIAN_POINT('Ctrl Pts',(-83.3225831555504,-2.99706694569032,
68.4933050443484));
#55128=CARTESIAN_POINT('Ctrl Pts',(-83.3353608395901,-2.98533323282093,
68.4922764783663));
#55129=CARTESIAN_POINT('Ctrl Pts',(-83.3395575143696,-2.98139431344585,
68.4920482857838));
#55130=CARTESIAN_POINT('Ctrl Pts',(-83.3457590477646,-2.97544772408497,
68.4918779910273));
#55131=CARTESIAN_POINT('Ctrl Pts',(-83.3478106467717,-2.97345915857087,
68.4918498917946));
#55132=CARTESIAN_POINT('Ctrl Pts',(-83.3518827575376,-2.96946983325068,
68.4918510247018));
#55133=CARTESIAN_POINT('Ctrl Pts',(-83.354203013897,-2.96716909254389,68.4918889124519));
#55134=CARTESIAN_POINT('Ctrl Pts',(-83.4104766779843,-2.91085106427075,
68.4935139055717));
#55135=CARTESIAN_POINT('Ctrl Pts',(-83.4674723237323,-2.838162614945,68.5227290784896));
#55136=CARTESIAN_POINT('Ctrl Pts',(-83.5573929376881,-2.64912508052214,
68.636438268353));
#55137=CARTESIAN_POINT('Ctrl Pts',(-83.59,-2.53242495718233,68.7206842099906));
#55138=CARTESIAN_POINT('Ctrl Pts',(-83.59,-2.40000000000001,68.8330657242578));
#55139=CARTESIAN_POINT('',(-83.6305628535685,-2.40000000000001,68.8330657242578));
#55140=CARTESIAN_POINT('',(-83.59,-2.40000000000001,68.8330657242578));
#55141=CARTESIAN_POINT('',(-83.59,-2.40000000000001,68.8330657242578));
#55142=CARTESIAN_POINT('Ctrl Pts',(-82.79,-4.,68.8330657242578));
#55143=CARTESIAN_POINT('Ctrl Pts',(-82.8781350353569,-4.,68.7901894268455));
#55144=CARTESIAN_POINT('Ctrl Pts',(-82.9641672156171,-3.99269386732363,
68.7513422007487));
#55145=CARTESIAN_POINT('Ctrl Pts',(-83.047294945123,-3.97912863028611,68.7165431137518));
#55146=CARTESIAN_POINT('Ctrl Pts',(-83.1352801201528,-3.9647707287512,68.6797105937432));
#55147=CARTESIAN_POINT('Ctrl Pts',(-83.2200105423739,-3.94340160709907,
68.6474133539507));
#55148=CARTESIAN_POINT('Ctrl Pts',(-83.3005498664581,-3.91631302891331,
68.6196465072808));
#55149=CARTESIAN_POINT('Ctrl Pts',(-83.3490063626748,-3.90001518185163,
68.6029405798855));
#55150=CARTESIAN_POINT('Ctrl Pts',(-83.3959460898563,-3.88164790169975,
68.5878740346506));
#55151=CARTESIAN_POINT('Ctrl Pts',(-83.4411696748627,-3.86149856467227,
68.5744409514166));
#55152=CARTESIAN_POINT('Ctrl Pts',(-83.5368725214139,-3.81885822756997,
68.5460136539507));
#55153=CARTESIAN_POINT('Ctrl Pts',(-83.6251250918968,-3.76825636386172,
68.5249247721554));
#55154=CARTESIAN_POINT('Ctrl Pts',(-83.7053180342998,-3.71232347235178,
68.5111743060306));
#55155=CARTESIAN_POINT('Ctrl Pts',(-83.7454145055013,-3.6843570265968,68.5042990729681));
#55156=CARTESIAN_POINT('Ctrl Pts',(-83.783508253167,-3.65505504190423,68.4992584438234));
#55157=CARTESIAN_POINT('Ctrl Pts',(-83.8195886415687,-3.62472332759394,
68.4960524185962));
#55158=CARTESIAN_POINT('Ctrl Pts',(-83.8376288312364,-3.60955747424959,
68.4944494063854));
#55159=CARTESIAN_POINT('Ctrl Pts',(-83.8551663023162,-3.59413389910499,
68.4933050446952));
#55160=CARTESIAN_POINT('Ctrl Pts',(-83.8722032230969,-3.57848894082617,
68.4926193336937));
#55161=CARTESIAN_POINT('Ctrl Pts',(-83.8807216899086,-3.57066645578996,
68.4922764779345));
#55162=CARTESIAN_POINT('Ctrl Pts',(-83.8891150245838,-3.56278863087633,
68.4920482858408));
#55163=CARTESIAN_POINT('Ctrl Pts',(-83.8973837399326,-3.5548598410772,68.4919347559461));
#55164=CARTESIAN_POINT('Ctrl Pts',(-83.9015180955293,-3.55089544816994,
68.4918779910273));
#55165=CARTESIAN_POINT('Ctrl Pts',(-83.9056212935433,-3.54691831714174,
68.4918498917946));
#55166=CARTESIAN_POINT('Ctrl Pts',(-83.9096934043093,-3.54292899182155,
68.4918504582482));
#55167=CARTESIAN_POINT('Ctrl Pts',(-83.9137655150753,-3.53893966650135,
68.4918510247018));
#55168=CARTESIAN_POINT('Ctrl Pts',(-83.918406027794,-3.53433818508778,68.4918889124519));
#55169=CARTESIAN_POINT('Ctrl Pts',(-83.9218165528902,-3.53092497125305,
68.4919381546676));
#55170=CARTESIAN_POINT('Ctrl Pts',(-84.0309533559686,-3.42170212854153,
68.4935139055717));
#55171=CARTESIAN_POINT('Ctrl Pts',(-84.1449446474647,-3.27632522988999,
68.5227290784896));
#55172=CARTESIAN_POINT('Ctrl Pts',(-84.2348652614204,-3.08728769546713,
68.5795836734213));
#55173=CARTESIAN_POINT('Ctrl Pts',(-84.2643083303775,-3.02539037385596,
68.5981998025318));
#55174=CARTESIAN_POINT('Ctrl Pts',(-84.2911322238605,-2.95869691731586,
68.6197620638144));
#55175=CARTESIAN_POINT('Ctrl Pts',(-84.3138741189653,-2.88768751153503,
68.6442957957497));
#55176=CARTESIAN_POINT('Ctrl Pts',(-84.3355816359095,-2.81990785323989,
68.6677136507366));
#55177=CARTESIAN_POINT('Ctrl Pts',(-84.3535685888622,-2.7481966656002,68.6938386980911));
#55178=CARTESIAN_POINT('Ctrl Pts',(-84.3665908505951,-2.67300199653487,
68.7226721477159));
#55179=CARTESIAN_POINT('Ctrl Pts',(-84.3786851920698,-2.603165433317,68.7494510278218));
#55180=CARTESIAN_POINT('Ctrl Pts',(-84.3864964753952,-2.5303247318545,68.7785659004214));
#55181=CARTESIAN_POINT('Ctrl Pts',(-84.3890669981752,-2.45485641144071,
68.8100015749531));
#55182=CARTESIAN_POINT('Ctrl Pts',(-84.3896847131035,-2.43672083664923,
68.8175557913908));
#55183=CARTESIAN_POINT('Ctrl Pts',(-84.39,-2.41843358706486,68.8252439568516));
#55184=CARTESIAN_POINT('Ctrl Pts',(-84.39,-2.40000000000001,68.8330657242578));
#55185=CARTESIAN_POINT('Ctrl Pts',(-84.39,-2.4,-68.8330657242578));
#55186=CARTESIAN_POINT('Ctrl Pts',(-84.39,-2.63794131567597,-68.7173110464923));
#55187=CARTESIAN_POINT('Ctrl Pts',(-84.3367792388686,-2.85976398178808,
-68.6312955463343));
#55188=CARTESIAN_POINT('Ctrl Pts',(-84.2088582275566,-3.14687252143927,
-68.5460136539367));
#55189=CARTESIAN_POINT('Ctrl Pts',(-84.1582563638478,-3.23512509191915,
-68.5249247721426));
#55190=CARTESIAN_POINT('Ctrl Pts',(-84.0743570265853,-3.35541450551661,
-68.5042990729588));
#55191=CARTESIAN_POINT('Ctrl Pts',(-84.0450550418941,-3.39350825317956,
-68.4992584438155));
#55192=CARTESIAN_POINT('Ctrl Pts',(-83.9995574704317,-3.44762883577759,
-68.4944494059773));
#55193=CARTESIAN_POINT('Ctrl Pts',(-83.9841338913747,-3.46516631110745,
-68.4933050443442));
#55194=CARTESIAN_POINT('Ctrl Pts',(-83.960666465638,-3.49072167918432,-68.4922764783636));
#55195=CARTESIAN_POINT('Ctrl Pts',(-83.9527886268885,-3.49911502874262,
-68.4920482857816));
#55196=CARTESIAN_POINT('Ctrl Pts',(-83.9408954481679,-3.51151809553136,
-68.4918779910258));
#55197=CARTESIAN_POINT('Ctrl Pts',(-83.9369183171401,-3.51562129354503,
-68.4918498917935));
#55198=CARTESIAN_POINT('Ctrl Pts',(-83.9289396665005,-3.52376551507611,
-68.4918510247012));
#55199=CARTESIAN_POINT('Ctrl Pts',(-83.9243381850882,-3.52840602779358,
-68.4918889124516));
#55200=CARTESIAN_POINT('Ctrl Pts',(-83.8117021285277,-3.64095335598249,
-68.49351390558));
#55201=CARTESIAN_POINT('Ctrl Pts',(-83.6663252298652,-3.7549446474807,-68.522729078502));
#55202=CARTESIAN_POINT('Ctrl Pts',(-83.2882501610162,-3.9347858753853,-68.6364382683655));
#55203=CARTESIAN_POINT('Ctrl Pts',(-83.055117522837,-4.,-68.7205706579609));
#55204=CARTESIAN_POINT('Ctrl Pts',(-82.79,-4.,-68.8330657242578));
#55205=CARTESIAN_POINT('Ctrl Pts',(-83.59,-2.4,-68.8330657242578));
#55206=CARTESIAN_POINT('Ctrl Pts',(-83.59,-2.51889840092331,-68.7173813501791));
#55207=CARTESIAN_POINT('Ctrl Pts',(-83.5633896194343,-2.62988199089404,
-68.6312955463343));
#55208=CARTESIAN_POINT('Ctrl Pts',(-83.4994291137783,-2.77343626071964,
-68.5460136539367));
#55209=CARTESIAN_POINT('Ctrl Pts',(-83.4741281819239,-2.81756254595958,
-68.5249247721426));
#55210=CARTESIAN_POINT('Ctrl Pts',(-83.4321785132927,-2.87770725275831,
-68.5042990729588));
#55211=CARTESIAN_POINT('Ctrl Pts',(-83.4175275209471,-2.89675412658978,
-68.4992584438155));
#55212=CARTESIAN_POINT('Ctrl Pts',(-83.3947787352159,-2.92381441788879,
-68.4944494059773));
#55213=CARTESIAN_POINT('Ctrl Pts',(-83.3870669456874,-2.93258315555372,
-68.4933050443442));
#55214=CARTESIAN_POINT('Ctrl Pts',(-83.375333232819,-2.94536083959216,-68.4922764783636));
#55215=CARTESIAN_POINT('Ctrl Pts',(-83.3713943134443,-2.94955751437131,
-68.4920482857816));
#55216=CARTESIAN_POINT('Ctrl Pts',(-83.3654477240839,-2.95575904776568,
-68.4918779910258));
#55217=CARTESIAN_POINT('Ctrl Pts',(-83.3634591585701,-2.95781064677251,
-68.4918498917935));
#55218=CARTESIAN_POINT('Ctrl Pts',(-83.3594698332502,-2.96188275753805,
-68.4918510247012));
#55219=CARTESIAN_POINT('Ctrl Pts',(-83.3571690925441,-2.96420301389679,
-68.4918889124516));
#55220=CARTESIAN_POINT('Ctrl Pts',(-83.3008510642638,-3.02047667799125,
-68.49351390558));
#55221=CARTESIAN_POINT('Ctrl Pts',(-83.2281626149326,-3.07747232374035,
-68.522729078502));
#55222=CARTESIAN_POINT('Ctrl Pts',(-83.0391250805081,-3.16739293769265,
-68.6364382683655));
#55223=CARTESIAN_POINT('Ctrl Pts',(-82.9224249571724,-3.2,-68.720684209999));
#55224=CARTESIAN_POINT('Ctrl Pts',(-82.79,-3.2,-68.8330657242578));
#55225=CARTESIAN_POINT('',(-83.7536699000375,-2.40000000000001,-68.8330657242578));
#55226=CARTESIAN_POINT('',(-84.39,-2.4,-68.8330657242578));
#55227=CARTESIAN_POINT('',(-84.39,-2.4,-68.8330657242578));
#55228=CARTESIAN_POINT('Ctrl Pts',(-83.59,-2.40000000000001,-68.8330657242578));
#55229=CARTESIAN_POINT('Ctrl Pts',(-83.59,-2.51889840092331,-68.7173813501791));
#55230=CARTESIAN_POINT('Ctrl Pts',(-83.5633896194343,-2.62988199089404,
-68.6312955463343));
#55231=CARTESIAN_POINT('Ctrl Pts',(-83.4994291137783,-2.77343626071964,
-68.5460136539367));
#55232=CARTESIAN_POINT('Ctrl Pts',(-83.4741281819239,-2.81756254595958,
-68.5249247721426));
#55233=CARTESIAN_POINT('Ctrl Pts',(-83.4321785132927,-2.87770725275831,
-68.5042990729588));
#55234=CARTESIAN_POINT('Ctrl Pts',(-83.4175275209471,-2.89675412658978,
-68.4992584438155));
#55235=CARTESIAN_POINT('Ctrl Pts',(-83.3947787352159,-2.92381441788879,
-68.4944494059773));
#55236=CARTESIAN_POINT('Ctrl Pts',(-83.3870669456874,-2.93258315555372,
-68.4933050443442));
#55237=CARTESIAN_POINT('Ctrl Pts',(-83.375333232819,-2.94536083959216,-68.4922764783636));
#55238=CARTESIAN_POINT('Ctrl Pts',(-83.3713943134443,-2.94955751437131,
-68.4920482857816));
#55239=CARTESIAN_POINT('Ctrl Pts',(-83.3654477240839,-2.95575904776568,
-68.4918779910258));
#55240=CARTESIAN_POINT('Ctrl Pts',(-83.3634591585701,-2.95781064677251,
-68.4918498917935));
#55241=CARTESIAN_POINT('Ctrl Pts',(-83.3594698332502,-2.96188275753805,
-68.4918510247012));
#55242=CARTESIAN_POINT('Ctrl Pts',(-83.3571690925441,-2.96420301389679,
-68.4918889124516));
#55243=CARTESIAN_POINT('Ctrl Pts',(-83.3008510642638,-3.02047667799125,
-68.49351390558));
#55244=CARTESIAN_POINT('Ctrl Pts',(-83.2281626149326,-3.07747232374035,
-68.522729078502));
#55245=CARTESIAN_POINT('Ctrl Pts',(-83.0391250805081,-3.16739293769265,
-68.6364382683655));
#55246=CARTESIAN_POINT('Ctrl Pts',(-82.9224249571724,-3.2,-68.720684209999));
#55247=CARTESIAN_POINT('Ctrl Pts',(-82.79,-3.2,-68.8330657242578));
#55248=CARTESIAN_POINT('Ctrl Pts',(-84.39,-2.4,-68.8330657242578));
#55249=CARTESIAN_POINT('Ctrl Pts',(-84.39,-2.48813503534456,-68.7901894268515));
#55250=CARTESIAN_POINT('Ctrl Pts',(-84.3826938673257,-2.57416721559184,
-68.7513422007595));
#55251=CARTESIAN_POINT('Ctrl Pts',(-84.3691286302924,-2.65729494508488,
-68.7165431137664));
#55252=CARTESIAN_POINT('Ctrl Pts',(-84.3547707287616,-2.74528012010299,
-68.6797105937609));
#55253=CARTESIAN_POINT('Ctrl Pts',(-84.3334016071155,-2.83001054231243,
-68.6474133539704));
#55254=CARTESIAN_POINT('Ctrl Pts',(-84.3063130289378,-2.91054986638528,
-68.6196465073015));
#55255=CARTESIAN_POINT('Ctrl Pts',(-84.2900151818667,-2.9590063626376,-68.6029405798922));
#55256=CARTESIAN_POINT('Ctrl Pts',(-84.2716479017026,-3.00594608985223,
-68.5878740346456));
#55257=CARTESIAN_POINT('Ctrl Pts',(-84.2514985646606,-3.05116967488887,
-68.5744409514026));
#55258=CARTESIAN_POINT('Ctrl Pts',(-84.2088582275566,-3.14687252143927,
-68.5460136539367));
#55259=CARTESIAN_POINT('Ctrl Pts',(-84.1582563638478,-3.23512509191915,
-68.5249247721426));
#55260=CARTESIAN_POINT('Ctrl Pts',(-84.1023234723395,-3.31531803431746,
-68.5111743060201));
#55261=CARTESIAN_POINT('Ctrl Pts',(-84.0743570265853,-3.35541450551661,
-68.5042990729588));
#55262=CARTESIAN_POINT('Ctrl Pts',(-84.0450550418941,-3.39350825317956,
-68.4992584438155));
#55263=CARTESIAN_POINT('Ctrl Pts',(-84.0147233275859,-3.42958864157825,
-68.4960524185901));
#55264=CARTESIAN_POINT('Ctrl Pts',(-83.9995574742425,-3.44762883124453,
-68.4944494063801));
#55265=CARTESIAN_POINT('Ctrl Pts',(-83.9841338990991,-3.46516630232284,
-68.4933050446909));
#55266=CARTESIAN_POINT('Ctrl Pts',(-83.9684889408216,-3.48220322310181,
-68.4926193336904));
#55267=CARTESIAN_POINT('Ctrl Pts',(-83.9606664557861,-3.49072168991274,
-68.4922764779317));
#55268=CARTESIAN_POINT('Ctrl Pts',(-83.9527886308731,-3.49911502458717,
-68.4920482858386));
#55269=CARTESIAN_POINT('Ctrl Pts',(-83.9448598410748,-3.50738373993511,
-68.4919347559444));
#55270=CARTESIAN_POINT('Ctrl Pts',(-83.9408954481679,-3.51151809553136,
-68.4918779910258));
#55271=CARTESIAN_POINT('Ctrl Pts',(-83.9369183171401,-3.51562129354502,
-68.4918498917935));
#55272=CARTESIAN_POINT('Ctrl Pts',(-83.9329289918203,-3.51969340431057,
-68.4918504582473));
#55273=CARTESIAN_POINT('Ctrl Pts',(-83.9289396665005,-3.5237655150761,-68.4918510247012));
#55274=CARTESIAN_POINT('Ctrl Pts',(-83.9243381850882,-3.52840602779357,
-68.4918889124516));
#55275=CARTESIAN_POINT('Ctrl Pts',(-83.920924971253,-3.5318165528902,-68.4919381546676));
#55276=CARTESIAN_POINT('Ctrl Pts',(-83.8117021285274,-3.64095335598243,
-68.49351390558));
#55277=CARTESIAN_POINT('Ctrl Pts',(-83.6663252298652,-3.75494464748069,
-68.522729078502));
#55278=CARTESIAN_POINT('Ctrl Pts',(-83.4772876954407,-3.84486526143299,
-68.5795836734338));
#55279=CARTESIAN_POINT('Ctrl Pts',(-83.4153903738218,-3.87430833039238,
-68.5981998025465));
#55280=CARTESIAN_POINT('Ctrl Pts',(-83.3486969172739,-3.90113222387641,
-68.6197620638315));
#55281=CARTESIAN_POINT('Ctrl Pts',(-83.2776875114855,-3.92387411898109,
-68.6442957957694));
#55282=CARTESIAN_POINT('Ctrl Pts',(-83.2099078531827,-3.94558163592534,
-68.667713650759));
#55283=CARTESIAN_POINT('Ctrl Pts',(-83.1381966655355,-3.96356858887681,
-68.6938386981164));
#55284=CARTESIAN_POINT('Ctrl Pts',(-83.063001996463,-3.97659085060749,-68.7226721477443));
#55285=CARTESIAN_POINT('Ctrl Pts',(-82.9931654332377,-3.9886851920802,-68.7494510278535));
#55286=CARTESIAN_POINT('Ctrl Pts',(-82.920324731768,-3.99649647540249,-68.7785659004566));
#55287=CARTESIAN_POINT('Ctrl Pts',(-82.8448564113475,-3.99906699817842,
-68.810001574992));
#55288=CARTESIAN_POINT('Ctrl Pts',(-82.8267208365865,-3.9996847131046,-68.8175557914172));
#55289=CARTESIAN_POINT('Ctrl Pts',(-82.8084335870332,-4.,-68.825243956865));
#55290=CARTESIAN_POINT('Ctrl Pts',(-82.79,-4.,-68.8330657242578));
#55291=CARTESIAN_POINT('Origin',(-82.79,-2.4,137.681359688174));
#55292=CARTESIAN_POINT('Origin',(-82.79,-2.4,137.681359688174));
#55293=CARTESIAN_POINT('Origin',(-93.59,-1.84247779607695,-70.));
#55294=CARTESIAN_POINT('',(-82.79,-1.84247779607695,-80.));
#55295=CARTESIAN_POINT('',(-93.59,-1.84247779607695,-70.));
#55296=CARTESIAN_POINT('Origin',(-82.79,-2.40000000000001,-80.));
#55297=CARTESIAN_POINT('',(-82.79,86.,-80.));
#55298=CARTESIAN_POINT('Origin',(-84.39,91.,80.));
#55299=CARTESIAN_POINT('',(-84.39,91.,-75.));
#55300=CARTESIAN_POINT('',(-84.39,91.,75.));
#55301=CARTESIAN_POINT('Origin',(-82.79,-3.20000000000001,80.));
#55302=CARTESIAN_POINT('',(-82.79,86.,80.));
#55303=CARTESIAN_POINT('',(-82.79,-1.84247779607695,80.));
#55304=CARTESIAN_POINT('Origin',(-93.59,-1.84247779607695,70.));
#55305=CARTESIAN_POINT('',(-93.59,-1.84247779607695,70.));
#55306=CARTESIAN_POINT('Origin',(-93.59,-3.34247779607695,70.));
#55307=CARTESIAN_POINT('Origin',(-93.59,-3.34247779607695,-70.));
#55308=CARTESIAN_POINT('Ctrl Pts',(70.61,-2.4,68.8330657242578));
#55309=CARTESIAN_POINT('Ctrl Pts',(70.61,-2.63794131567576,68.7173110464924));
#55310=CARTESIAN_POINT('Ctrl Pts',(70.5567792388688,-2.8597639817878,68.6312955463345));
#55311=CARTESIAN_POINT('Ctrl Pts',(70.4288582275568,-3.146872521439,68.5460136539369));
#55312=CARTESIAN_POINT('Ctrl Pts',(70.378256363848,-3.23512509191891,68.5249247721427));
#55313=CARTESIAN_POINT('Ctrl Pts',(70.2943570265855,-3.35541450551644,68.5042990729589));
#55314=CARTESIAN_POINT('Ctrl Pts',(70.2650550418943,-3.39350825317942,68.4992584438156));
#55315=CARTESIAN_POINT('Ctrl Pts',(70.2195574704318,-3.44762883577749,68.4944494059775));
#55316=CARTESIAN_POINT('Ctrl Pts',(70.2041338913749,-3.46516631110737,68.4933050443442));
#55317=CARTESIAN_POINT('Ctrl Pts',(70.1806664656381,-3.49072167918427,68.4922764783636));
#55318=CARTESIAN_POINT('Ctrl Pts',(70.1727886268886,-3.49911502874257,68.4920482857815));
#55319=CARTESIAN_POINT('Ctrl Pts',(70.160895448168,-3.51151809553133,68.4918779910258));
#55320=CARTESIAN_POINT('Ctrl Pts',(70.1569183171401,-3.515621293545,68.4918498917935));
#55321=CARTESIAN_POINT('Ctrl Pts',(70.1489396665006,-3.52376551507609,68.4918510247012));
#55322=CARTESIAN_POINT('Ctrl Pts',(70.1443381850882,-3.52840602779357,68.4918889124516));
#55323=CARTESIAN_POINT('Ctrl Pts',(70.0317021285279,-3.64095335598228,68.4935139055799));
#55324=CARTESIAN_POINT('Ctrl Pts',(69.8863252298656,-3.75494464748045,68.5227290785018));
#55325=CARTESIAN_POINT('Ctrl Pts',(69.5082501610166,-3.93478587538516,68.6364382683652));
#55326=CARTESIAN_POINT('Ctrl Pts',(69.2751175228373,-4.,68.7205706579607));
#55327=CARTESIAN_POINT('Ctrl Pts',(69.01,-4.,68.8330657242578));
#55328=CARTESIAN_POINT('Ctrl Pts',(69.81,-2.4,68.8330657242578));
#55329=CARTESIAN_POINT('Ctrl Pts',(69.81,-2.51889840092321,68.7173813501793));
#55330=CARTESIAN_POINT('Ctrl Pts',(69.7833896194344,-2.6298819908939,68.6312955463345));
#55331=CARTESIAN_POINT('Ctrl Pts',(69.7194291137784,-2.7734362607195,68.5460136539369));
#55332=CARTESIAN_POINT('Ctrl Pts',(69.694128181924,-2.81756254595946,68.5249247721427));
#55333=CARTESIAN_POINT('Ctrl Pts',(69.6521785132928,-2.87770725275822,68.5042990729589));
#55334=CARTESIAN_POINT('Ctrl Pts',(69.6375275209471,-2.89675412658971,68.4992584438156));
#55335=CARTESIAN_POINT('Ctrl Pts',(69.6147787352159,-2.92381441788875,68.4944494059775));
#55336=CARTESIAN_POINT('Ctrl Pts',(69.6070669456874,-2.93258315555369,68.4933050443442));
#55337=CARTESIAN_POINT('Ctrl Pts',(69.595333232819,-2.94536083959214,68.4922764783636));
#55338=CARTESIAN_POINT('Ctrl Pts',(69.5913943134443,-2.94955751437128,68.4920482857815));
#55339=CARTESIAN_POINT('Ctrl Pts',(69.585447724084,-2.95575904776566,68.4918779910258));
#55340=CARTESIAN_POINT('Ctrl Pts',(69.5834591585701,-2.9578106467725,68.4918498917935));
#55341=CARTESIAN_POINT('Ctrl Pts',(69.5794698332503,-2.96188275753804,68.4918510247012));
#55342=CARTESIAN_POINT('Ctrl Pts',(69.5771690925441,-2.96420301389679,68.4918889124516));
#55343=CARTESIAN_POINT('Ctrl Pts',(69.520851064264,-3.02047667799114,68.4935139055799));
#55344=CARTESIAN_POINT('Ctrl Pts',(69.4481626149328,-3.07747232374023,68.5227290785018));
#55345=CARTESIAN_POINT('Ctrl Pts',(69.2591250805083,-3.16739293769258,68.6364382683652));
#55346=CARTESIAN_POINT('Ctrl Pts',(69.1424249571726,-3.2,68.7206842099989));
#55347=CARTESIAN_POINT('Ctrl Pts',(69.01,-3.2,68.8330657242578));
#55348=CARTESIAN_POINT('',(69.9736699000372,-2.4,68.8330657242578));
#55349=CARTESIAN_POINT('',(70.61,-2.4,68.8330657242578));
#55350=CARTESIAN_POINT('',(70.61,-2.4,68.8330657242578));
#55351=CARTESIAN_POINT('Ctrl Pts',(69.81,-2.4,68.8330657242578));
#55352=CARTESIAN_POINT('Ctrl Pts',(69.81,-2.51889840092321,68.7173813501793));
#55353=CARTESIAN_POINT('Ctrl Pts',(69.7833896194344,-2.6298819908939,68.6312955463345));
#55354=CARTESIAN_POINT('Ctrl Pts',(69.7194291137784,-2.7734362607195,68.5460136539369));
#55355=CARTESIAN_POINT('Ctrl Pts',(69.694128181924,-2.81756254595946,68.5249247721427));
#55356=CARTESIAN_POINT('Ctrl Pts',(69.6521785132928,-2.87770725275822,68.5042990729589));
#55357=CARTESIAN_POINT('Ctrl Pts',(69.6375275209471,-2.89675412658971,68.4992584438156));
#55358=CARTESIAN_POINT('Ctrl Pts',(69.6147787352159,-2.92381441788875,68.4944494059775));
#55359=CARTESIAN_POINT('Ctrl Pts',(69.6070669456874,-2.93258315555369,68.4933050443442));
#55360=CARTESIAN_POINT('Ctrl Pts',(69.595333232819,-2.94536083959214,68.4922764783636));
#55361=CARTESIAN_POINT('Ctrl Pts',(69.5913943134443,-2.94955751437128,68.4920482857815));
#55362=CARTESIAN_POINT('Ctrl Pts',(69.585447724084,-2.95575904776566,68.4918779910258));
#55363=CARTESIAN_POINT('Ctrl Pts',(69.5834591585701,-2.9578106467725,68.4918498917935));
#55364=CARTESIAN_POINT('Ctrl Pts',(69.5794698332503,-2.96188275753804,68.4918510247012));
#55365=CARTESIAN_POINT('Ctrl Pts',(69.5771690925441,-2.96420301389679,68.4918889124516));
#55366=CARTESIAN_POINT('Ctrl Pts',(69.520851064264,-3.02047667799114,68.4935139055799));
#55367=CARTESIAN_POINT('Ctrl Pts',(69.4481626149328,-3.07747232374023,68.5227290785018));
#55368=CARTESIAN_POINT('Ctrl Pts',(69.2591250805083,-3.16739293769258,68.6364382683652));
#55369=CARTESIAN_POINT('Ctrl Pts',(69.1424249571726,-3.2,68.7206842099989));
#55370=CARTESIAN_POINT('Ctrl Pts',(69.01,-3.2,68.8330657242578));
#55371=CARTESIAN_POINT('Ctrl Pts',(70.61,-2.4,68.8330657242578));
#55372=CARTESIAN_POINT('Ctrl Pts',(70.61,-2.48813503534593,68.7901894268509));
#55373=CARTESIAN_POINT('Ctrl Pts',(70.6026938673255,-2.57416721559453,68.7513422007584));
#55374=CARTESIAN_POINT('Ctrl Pts',(70.5891286302918,-2.65729494508879,68.7165431137648));
#55375=CARTESIAN_POINT('Ctrl Pts',(70.5747707287605,-2.7452801201082,68.6797105937589));
#55376=CARTESIAN_POINT('Ctrl Pts',(70.5534016071138,-2.83001054231882,68.6474133539681));
#55377=CARTESIAN_POINT('Ctrl Pts',(70.5263130289353,-2.91054986639271,68.619646507299));
#55378=CARTESIAN_POINT('Ctrl Pts',(70.5100151818649,-2.9590063626423,68.6029405798908));
#55379=CARTESIAN_POINT('Ctrl Pts',(70.4916479017016,-3.00594608985435,68.5878740346451));
#55380=CARTESIAN_POINT('Ctrl Pts',(70.4714985646607,-3.0511696748886,68.5744409514028));
#55381=CARTESIAN_POINT('Ctrl Pts',(70.4288582275567,-3.14687252143901,68.5460136539369));
#55382=CARTESIAN_POINT('Ctrl Pts',(70.3782563638479,-3.23512509191891,68.5249247721427));
#55383=CARTESIAN_POINT('Ctrl Pts',(70.3223234723396,-3.31531803431726,68.5111743060202));
#55384=CARTESIAN_POINT('Ctrl Pts',(70.2943570265855,-3.35541450551644,68.5042990729589));
#55385=CARTESIAN_POINT('Ctrl Pts',(70.2650550418943,-3.39350825317941,68.4992584438156));
#55386=CARTESIAN_POINT('Ctrl Pts',(70.234723327586,-3.42958864157812,68.4960524185902));
#55387=CARTESIAN_POINT('Ctrl Pts',(70.2195574742427,-3.44762883124441,68.4944494063803));
#55388=CARTESIAN_POINT('Ctrl Pts',(70.2041338990992,-3.46516630232275,68.4933050446909));
#55389=CARTESIAN_POINT('Ctrl Pts',(70.1884889408217,-3.48220322310175,68.4926193336904));
#55390=CARTESIAN_POINT('Ctrl Pts',(70.1806664557862,-3.4907216899127,68.4922764779317));
#55391=CARTESIAN_POINT('Ctrl Pts',(70.1727886308732,-3.49911502458712,68.4920482858386));
#55392=CARTESIAN_POINT('Ctrl Pts',(70.1648598410748,-3.50738373993507,68.4919347559444));
#55393=CARTESIAN_POINT('Ctrl Pts',(70.160895448168,-3.51151809553132,68.4918779910258));
#55394=CARTESIAN_POINT('Ctrl Pts',(70.1569183171401,-3.51562129354499,68.4918498917935));
#55395=CARTESIAN_POINT('Ctrl Pts',(70.1529289918203,-3.51969340431054,68.4918504582473));
#55396=CARTESIAN_POINT('Ctrl Pts',(70.1489396665006,-3.52376551507608,68.4918510247012));
#55397=CARTESIAN_POINT('Ctrl Pts',(70.1443381850882,-3.52840602779357,68.4918889124516));
#55398=CARTESIAN_POINT('Ctrl Pts',(70.1409249712531,-3.5318165528902,68.4919381546676));
#55399=CARTESIAN_POINT('Ctrl Pts',(70.0317021285278,-3.64095335598229,68.4935139055799));
#55400=CARTESIAN_POINT('Ctrl Pts',(69.8863252298656,-3.75494464748044,68.5227290785018));
#55401=CARTESIAN_POINT('Ctrl Pts',(69.6972876954411,-3.8448652614328,68.5795836734335));
#55402=CARTESIAN_POINT('Ctrl Pts',(69.6353903738228,-3.87430833039194,68.5981998025461));
#55403=CARTESIAN_POINT('Ctrl Pts',(69.5686969172756,-3.90113222387577,68.6197620638309));
#55404=CARTESIAN_POINT('Ctrl Pts',(69.4976875114879,-3.92387411898034,68.6442957957685));
#55405=CARTESIAN_POINT('Ctrl Pts',(69.4299078531858,-3.94558163592449,68.6677136507578));
#55406=CARTESIAN_POINT('Ctrl Pts',(69.3581966655392,-3.96356858887595,68.693838698115));
#55407=CARTESIAN_POINT('Ctrl Pts',(69.2830019964674,-3.97659085060672,68.7226721477426));
#55408=CARTESIAN_POINT('Ctrl Pts',(69.2131654332428,-3.98868519207953,68.7494510278515));
#55409=CARTESIAN_POINT('Ctrl Pts',(69.1403247317738,-3.99649647540199,68.7785659004542));
#55410=CARTESIAN_POINT('Ctrl Pts',(69.0648564113539,-3.9990669981782,68.8100015749893));
#55411=CARTESIAN_POINT('Ctrl Pts',(69.0467208365909,-3.99968471310452,68.8175557914153));
#55412=CARTESIAN_POINT('Ctrl Pts',(69.0284335870354,-4.,68.825243956864));
#55413=CARTESIAN_POINT('Ctrl Pts',(69.01,-4.,68.8330657242578));
#55414=CARTESIAN_POINT('Ctrl Pts',(69.01,-4.,-68.8330657242578));
#55415=CARTESIAN_POINT('Ctrl Pts',(69.2479413156758,-4.,-68.7173110464924));
#55416=CARTESIAN_POINT('Ctrl Pts',(69.4697639817879,-3.94677923886873,-68.6312955463344));
#55417=CARTESIAN_POINT('Ctrl Pts',(69.7568725214391,-3.81885822755673,-68.5460136539369));
#55418=CARTESIAN_POINT('Ctrl Pts',(69.845125091919,-3.76825636384791,-68.5249247721427));
#55419=CARTESIAN_POINT('Ctrl Pts',(69.9654145055165,-3.68435702658545,-68.5042990729589));
#55420=CARTESIAN_POINT('Ctrl Pts',(70.0035082531795,-3.65505504189424,-68.4992584438156));
#55421=CARTESIAN_POINT('Ctrl Pts',(70.0576288357775,-3.6095574704318,-68.4944494059774));
#55422=CARTESIAN_POINT('Ctrl Pts',(70.0751663111074,-3.59413389137481,-68.4933050443442));
#55423=CARTESIAN_POINT('Ctrl Pts',(70.1007216791843,-3.57066646563801,-68.4922764783636));
#55424=CARTESIAN_POINT('Ctrl Pts',(70.1091150287426,-3.56278862688857,-68.4920482857816));
#55425=CARTESIAN_POINT('Ctrl Pts',(70.1215180955314,-3.55089544816793,-68.4918779910258));
#55426=CARTESIAN_POINT('Ctrl Pts',(70.125621293545,-3.54691831714011,-68.4918498917935));
#55427=CARTESIAN_POINT('Ctrl Pts',(70.1337655150761,-3.53893966650051,-68.4918510247012));
#55428=CARTESIAN_POINT('Ctrl Pts',(70.1384060277936,-3.5343381850882,-68.4918889124516));
#55429=CARTESIAN_POINT('Ctrl Pts',(70.2509533559824,-3.42170212852781,-68.4935139055799));
#55430=CARTESIAN_POINT('Ctrl Pts',(70.3649446474806,-3.27632522986542,-68.5227290785019));
#55431=CARTESIAN_POINT('Ctrl Pts',(70.5447858753852,-2.89825016101646,-68.6364382683653));
#55432=CARTESIAN_POINT('Ctrl Pts',(70.61,-2.66511752283727,-68.7205706579607));
#55433=CARTESIAN_POINT('Ctrl Pts',(70.61,-2.4,-68.8330657242578));
#55434=CARTESIAN_POINT('Ctrl Pts',(69.01,-3.2,-68.8330657242578));
#55435=CARTESIAN_POINT('Ctrl Pts',(69.1288984009232,-3.2,-68.7173813501792));
#55436=CARTESIAN_POINT('Ctrl Pts',(69.2398819908939,-3.17338961943437,-68.6312955463344));
#55437=CARTESIAN_POINT('Ctrl Pts',(69.3834362607195,-3.10942911377837,-68.5460136539369));
#55438=CARTESIAN_POINT('Ctrl Pts',(69.4275625459595,-3.08412818192396,-68.5249247721427));
#55439=CARTESIAN_POINT('Ctrl Pts',(69.4877072527583,-3.04217851329272,-68.5042990729589));
#55440=CARTESIAN_POINT('Ctrl Pts',(69.5067541265897,-3.02752752094712,-68.4992584438156));
#55441=CARTESIAN_POINT('Ctrl Pts',(69.5338144178888,-3.0047787352159,-68.4944494059774));
#55442=CARTESIAN_POINT('Ctrl Pts',(69.5425831555537,-2.99706694568741,-68.4933050443442));
#55443=CARTESIAN_POINT('Ctrl Pts',(69.5553608395922,-2.98533323281901,-68.4922764783636));
#55444=CARTESIAN_POINT('Ctrl Pts',(69.5595575143713,-2.98139431344429,-68.4920482857816));
#55445=CARTESIAN_POINT('Ctrl Pts',(69.5657590477657,-2.97544772408396,-68.4918779910258));
#55446=CARTESIAN_POINT('Ctrl Pts',(69.5678106467725,-2.97345915857006,-68.4918498917935));
#55447=CARTESIAN_POINT('Ctrl Pts',(69.5718827575381,-2.96946983325026,-68.4918510247012));
#55448=CARTESIAN_POINT('Ctrl Pts',(69.5742030138968,-2.9671690925441,-68.4918889124516));
#55449=CARTESIAN_POINT('Ctrl Pts',(69.6304766779912,-2.9108510642639,-68.4935139055799));
#55450=CARTESIAN_POINT('Ctrl Pts',(69.6874723237403,-2.83816261493271,-68.5227290785019));
#55451=CARTESIAN_POINT('Ctrl Pts',(69.7773929376926,-2.64912508050823,-68.6364382683653));
#55452=CARTESIAN_POINT('Ctrl Pts',(69.81,-2.53242495717256,-68.7206842099989));
#55453=CARTESIAN_POINT('Ctrl Pts',(69.81,-2.4,-68.8330657242578));
#55454=CARTESIAN_POINT('Ctrl Pts',(69.01,-3.2,-68.8330657242578));
#55455=CARTESIAN_POINT('Ctrl Pts',(69.1288984009232,-3.2,-68.7173813501792));
#55456=CARTESIAN_POINT('Ctrl Pts',(69.2398819908939,-3.17338961943437,-68.6312955463344));
#55457=CARTESIAN_POINT('Ctrl Pts',(69.3834362607195,-3.10942911377837,-68.5460136539369));
#55458=CARTESIAN_POINT('Ctrl Pts',(69.4275625459595,-3.08412818192396,-68.5249247721427));
#55459=CARTESIAN_POINT('Ctrl Pts',(69.4877072527583,-3.04217851329272,-68.5042990729589));
#55460=CARTESIAN_POINT('Ctrl Pts',(69.5067541265897,-3.02752752094712,-68.4992584438156));
#55461=CARTESIAN_POINT('Ctrl Pts',(69.5338144178888,-3.0047787352159,-68.4944494059774));
#55462=CARTESIAN_POINT('Ctrl Pts',(69.5425831555537,-2.99706694568741,-68.4933050443442));
#55463=CARTESIAN_POINT('Ctrl Pts',(69.5553608395922,-2.98533323281901,-68.4922764783636));
#55464=CARTESIAN_POINT('Ctrl Pts',(69.5595575143713,-2.98139431344429,-68.4920482857816));
#55465=CARTESIAN_POINT('Ctrl Pts',(69.5657590477657,-2.97544772408396,-68.4918779910258));
#55466=CARTESIAN_POINT('Ctrl Pts',(69.5678106467725,-2.97345915857006,-68.4918498917935));
#55467=CARTESIAN_POINT('Ctrl Pts',(69.5718827575381,-2.96946983325026,-68.4918510247012));
#55468=CARTESIAN_POINT('Ctrl Pts',(69.5742030138968,-2.9671690925441,-68.4918889124516));
#55469=CARTESIAN_POINT('Ctrl Pts',(69.6304766779912,-2.9108510642639,-68.4935139055799));
#55470=CARTESIAN_POINT('Ctrl Pts',(69.6874723237403,-2.83816261493271,-68.5227290785019));
#55471=CARTESIAN_POINT('Ctrl Pts',(69.7773929376926,-2.64912508050823,-68.6364382683653));
#55472=CARTESIAN_POINT('Ctrl Pts',(69.81,-2.53242495717256,-68.7206842099989));
#55473=CARTESIAN_POINT('Ctrl Pts',(69.81,-2.4,-68.8330657242578));
#55474=CARTESIAN_POINT('',(69.8505628535685,-2.4,-68.8330657242578));
#55475=CARTESIAN_POINT('',(69.81,-2.4,-68.8330657242578));
#55476=CARTESIAN_POINT('',(69.81,-2.4,-68.8330657242578));
#55477=CARTESIAN_POINT('Ctrl Pts',(69.01,-4.,-68.8330657242578));
#55478=CARTESIAN_POINT('Ctrl Pts',(69.0981350353444,-4.,-68.7901894268517));
#55479=CARTESIAN_POINT('Ctrl Pts',(69.1841672155914,-3.99269386732579,-68.7513422007598));
#55480=CARTESIAN_POINT('Ctrl Pts',(69.2672949450843,-3.97912863029249,-68.7165431137667));
#55481=CARTESIAN_POINT('Ctrl Pts',(69.3552801201021,-3.96477072876174,-68.6797105937613));
#55482=CARTESIAN_POINT('Ctrl Pts',(69.4400105423113,-3.9434016071158,-68.6474133539709));
#55483=CARTESIAN_POINT('Ctrl Pts',(69.520549866384,-3.91631302893826,-68.619646507302));
#55484=CARTESIAN_POINT('Ctrl Pts',(69.5690063626367,-3.90001518186709,-68.6029405798925));
#55485=CARTESIAN_POINT('Ctrl Pts',(69.6159460898517,-3.88164790170279,-68.5878740346459));
#55486=CARTESIAN_POINT('Ctrl Pts',(69.6611696748886,-3.86149856466073,-68.5744409514027));
#55487=CARTESIAN_POINT('Ctrl Pts',(69.756872521439,-3.81885822755673,-68.5460136539369));
#55488=CARTESIAN_POINT('Ctrl Pts',(69.845125091919,-3.76825636384791,-68.5249247721427));
#55489=CARTESIAN_POINT('Ctrl Pts',(69.9253180343173,-3.7123234723396,-68.5111743060202));
#55490=CARTESIAN_POINT('Ctrl Pts',(69.9654145055165,-3.68435702658545,-68.5042990729589));
#55491=CARTESIAN_POINT('Ctrl Pts',(70.0035082531795,-3.65505504189424,-68.4992584438156));
#55492=CARTESIAN_POINT('Ctrl Pts',(70.0395886415782,-3.62472332758594,-68.4960524185901));
#55493=CARTESIAN_POINT('Ctrl Pts',(70.0576288312445,-3.6095574742426,-68.4944494063802));
#55494=CARTESIAN_POINT('Ctrl Pts',(70.0751663023228,-3.59413389909915,-68.4933050446909));
#55495=CARTESIAN_POINT('Ctrl Pts',(70.0922032231018,-3.57848894082167,-68.4926193336904));
#55496=CARTESIAN_POINT('Ctrl Pts',(70.1007216899127,-3.57066645578614,-68.4922764779317));
#55497=CARTESIAN_POINT('Ctrl Pts',(70.1091150245872,-3.56278863087319,-68.4920482858386));
#55498=CARTESIAN_POINT('Ctrl Pts',(70.1173837399351,-3.55485984107481,-68.4919347559444));
#55499=CARTESIAN_POINT('Ctrl Pts',(70.1215180955314,-3.55089544816793,-68.4918779910258));
#55500=CARTESIAN_POINT('Ctrl Pts',(70.125621293545,-3.54691831714011,-68.4918498917935));
#55501=CARTESIAN_POINT('Ctrl Pts',(70.1296934043106,-3.54292899182031,-68.4918504582473));
#55502=CARTESIAN_POINT('Ctrl Pts',(70.1337655150761,-3.53893966650051,-68.4918510247012));
#55503=CARTESIAN_POINT('Ctrl Pts',(70.1384060277936,-3.53433818508819,-68.4918889124516));
#55504=CARTESIAN_POINT('Ctrl Pts',(70.1418165528902,-3.53092497125303,-68.4919381546676));
#55505=CARTESIAN_POINT('Ctrl Pts',(70.2509533559824,-3.42170212852774,-68.4935139055799));
#55506=CARTESIAN_POINT('Ctrl Pts',(70.3649446474806,-3.27632522986542,-68.5227290785019));
#55507=CARTESIAN_POINT('Ctrl Pts',(70.4548652614329,-3.08728769544094,-68.5795836734336));
#55508=CARTESIAN_POINT('Ctrl Pts',(70.4843083303921,-3.02539037382255,-68.5981998025462));
#55509=CARTESIAN_POINT('Ctrl Pts',(70.5111322238759,-2.95869691727524,-68.619762063831));
#55510=CARTESIAN_POINT('Ctrl Pts',(70.5338741189805,-2.88768751148745,-68.6442957957687));
#55511=CARTESIAN_POINT('Ctrl Pts',(70.5555816359246,-2.81990785318532,-68.667713650758));
#55512=CARTESIAN_POINT('Ctrl Pts',(70.573568588876,-2.74819666553881,-68.6938386981152));
#55513=CARTESIAN_POINT('Ctrl Pts',(70.5865908506068,-2.67300199646701,-68.7226721477428));
#55514=CARTESIAN_POINT('Ctrl Pts',(70.5986851920796,-2.60316543324227,-68.7494510278517));
#55515=CARTESIAN_POINT('Ctrl Pts',(70.6064964754021,-2.53032473177313,-68.7785659004545));
#55516=CARTESIAN_POINT('Ctrl Pts',(70.6090669981782,-2.45485641135309,-68.8100015749897));
#55517=CARTESIAN_POINT('Ctrl Pts',(70.6096847131045,-2.4367208365903,-68.8175557914156));
#55518=CARTESIAN_POINT('Ctrl Pts',(70.61,-2.41843358703513,-68.8252439568642));
#55519=CARTESIAN_POINT('Ctrl Pts',(70.61,-2.4,-68.8330657242578));
#55520=CARTESIAN_POINT('Origin',(69.01,-2.4,-137.681359688174));
#55521=CARTESIAN_POINT('Origin',(69.01,-2.4,-137.681359688174));
#55522=CARTESIAN_POINT('Origin',(79.81,-1.84247779607689,70.));
#55523=CARTESIAN_POINT('',(-82.79,-1.84247779607832,80.));
#55524=CARTESIAN_POINT('',(79.81,-1.84247779607689,70.));
#55525=CARTESIAN_POINT('Origin',(-82.79,-2.4,80.));
#55526=CARTESIAN_POINT('',(69.81,86.,80.));
#55527=CARTESIAN_POINT('Origin',(69.81,91.,80.));
#55528=CARTESIAN_POINT('',(69.81,91.,-75.));
#55529=CARTESIAN_POINT('',(70.61,91.,75.));
#55530=CARTESIAN_POINT('Origin',(69.01,-3.19999999999999,-80.));
#55531=CARTESIAN_POINT('',(69.01,86.,-80.));
#55532=CARTESIAN_POINT('',(69.01,-1.84247779607698,-80.));
#55533=CARTESIAN_POINT('Origin',(79.81,-1.84247779607689,-70.));
#55534=CARTESIAN_POINT('',(79.81,-1.84247779607689,-70.));
#55535=CARTESIAN_POINT('Origin',(79.81,-3.3424777960769,-70.));
#55536=CARTESIAN_POINT('Origin',(79.81,-3.3424777960769,70.));
#55537=CARTESIAN_POINT('Origin',(61.61,-4.,-68.39));
#55538=CARTESIAN_POINT('Origin',(56.338675369116,-2.,-68.39));
#55539=CARTESIAN_POINT('Origin',(66.8813246308841,-2.,-68.39));
#55540=CARTESIAN_POINT('Origin',(61.61,-4.,-64.39));
#55541=CARTESIAN_POINT('Origin',(66.8813246308841,-2.,-64.39));
#55542=CARTESIAN_POINT('Origin',(56.338675369116,-2.,-64.39));
#55543=CARTESIAN_POINT('Origin',(56.338675369116,-2.,-68.39));
#55544=CARTESIAN_POINT('',(58.1495932410337,-2.84886775246144,-68.39));
#55545=CARTESIAN_POINT('Origin',(56.338675369116,-2.,-68.39));
#55546=CARTESIAN_POINT('',(58.1495932410337,-2.84886775246144,-64.39));
#55547=CARTESIAN_POINT('',(58.1495932410337,-2.84886775246144,-68.39));
#55548=CARTESIAN_POINT('Origin',(56.338675369116,-2.,-64.39));
#55549=CARTESIAN_POINT('Origin',(66.8813246308841,-2.,-66.39));
#55550=CARTESIAN_POINT('',(65.0704067589663,-2.84886775246144,-64.39));
#55551=CARTESIAN_POINT('Origin',(66.8813246308841,-2.,-64.39));
#55552=CARTESIAN_POINT('',(65.0704067589663,-2.84886775246144,-68.39));
#55553=CARTESIAN_POINT('',(65.0704067589663,-2.84886775246144,-68.39));
#55554=CARTESIAN_POINT('Origin',(66.8813246308841,-2.,-68.39));
#55555=CARTESIAN_POINT('Origin',(66.8813246308841,-2.,-64.39));
#55556=CARTESIAN_POINT('',(57.4252260922666,-2.50932065147687,-64.39));
#55557=CARTESIAN_POINT('Origin',(56.338675369116,-2.,-64.39));
#55558=CARTESIAN_POINT('',(58.7053050692247,-1.66334918565392,-64.39));
#55559=CARTESIAN_POINT('',(59.11,-0.8,-64.39));
#55560=CARTESIAN_POINT('',(60.0634934731631,-0.8,-64.39));
#55561=CARTESIAN_POINT('Origin',(60.0634934731631,-2.3,-64.39));
#55562=CARTESIAN_POINT('',(63.156506526837,-0.8,-64.39));
#55563=CARTESIAN_POINT('',(59.11,-0.8,-64.39));
#55564=CARTESIAN_POINT('',(64.5146949307753,-1.66334918565392,-64.39));
#55565=CARTESIAN_POINT('Origin',(63.156506526837,-2.3,-64.39));
#55566=CARTESIAN_POINT('',(64.11,-0.8,-64.39));
#55567=CARTESIAN_POINT('',(65.7947739077334,-2.50932065147687,-64.39));
#55568=CARTESIAN_POINT('Origin',(66.8813246308841,-2.,-64.39));
#55569=CARTESIAN_POINT('',(65.2390620795424,-1.32380208466934,-64.39));
#55570=CARTESIAN_POINT('',(64.8343671487671,-0.460452899015424,-64.39));
#55571=CARTESIAN_POINT('',(63.156506526837,1.0842021724855E-16,-64.39));
#55572=CARTESIAN_POINT('Origin',(63.156506526837,-2.3,-64.39));
#55573=CARTESIAN_POINT('',(60.0634934731631,-4.33680868994202E-16,-64.39));
#55574=CARTESIAN_POINT('',(59.11,1.0842021724855E-16,-64.39));
#55575=CARTESIAN_POINT('',(57.9809379204577,-1.32380208466934,-64.39));
#55576=CARTESIAN_POINT('Origin',(60.0634934731631,-2.3,-64.39));
#55577=CARTESIAN_POINT('',(58.3856328512329,-0.460452899015424,-64.39));
#55578=CARTESIAN_POINT('Origin',(59.11,-0.8,-68.39));
#55579=CARTESIAN_POINT('',(65.7947739077334,-2.50932065147687,-68.39));
#55580=CARTESIAN_POINT('Origin',(66.8813246308841,-2.,-68.39));
#55581=CARTESIAN_POINT('',(64.5146949307753,-1.66334918565392,-68.39));
#55582=CARTESIAN_POINT('',(64.11,-0.8,-68.39));
#55583=CARTESIAN_POINT('',(63.156506526837,-0.8,-68.39));
#55584=CARTESIAN_POINT('Origin',(63.156506526837,-2.3,-68.39));
#55585=CARTESIAN_POINT('',(60.0634934731631,-0.8,-68.39));
#55586=CARTESIAN_POINT('',(59.11,-0.8,-68.39));
#55587=CARTESIAN_POINT('',(58.7053050692247,-1.66334918565392,-68.39));
#55588=CARTESIAN_POINT('Origin',(60.0634934731631,-2.3,-68.39));
#55589=CARTESIAN_POINT('',(59.11,-0.8,-68.39));
#55590=CARTESIAN_POINT('',(57.4252260922666,-2.50932065147687,-68.39));
#55591=CARTESIAN_POINT('Origin',(56.338675369116,-2.,-68.39));
#55592=CARTESIAN_POINT('',(57.9809379204577,-1.32380208466934,-68.39));
#55593=CARTESIAN_POINT('',(58.3856328512329,-0.460452899015424,-68.39));
#55594=CARTESIAN_POINT('',(60.0634934731631,1.0842021724855E-16,-68.39));
#55595=CARTESIAN_POINT('Origin',(60.0634934731631,-2.3,-68.39));
#55596=CARTESIAN_POINT('',(63.156506526837,1.0842021724855E-16,-68.39));
#55597=CARTESIAN_POINT('',(59.11,1.0842021724855E-16,-68.39));
#55598=CARTESIAN_POINT('',(65.2390620795424,-1.32380208466934,-68.39));
#55599=CARTESIAN_POINT('Origin',(63.156506526837,-2.3,-68.39));
#55600=CARTESIAN_POINT('',(64.8343671487671,-0.460452899015424,-68.39));
#55601=CARTESIAN_POINT('Origin',(60.0634934731631,-2.3,-68.39));
#55602=CARTESIAN_POINT('',(60.0634934731631,-0.8,-68.39));
#55603=CARTESIAN_POINT('',(58.7053050692247,-1.66334918565392,-68.39));
#55604=CARTESIAN_POINT('Origin',(63.156506526837,-2.3,-68.39));
#55605=CARTESIAN_POINT('',(64.5146949307753,-1.66334918565392,-68.39));
#55606=CARTESIAN_POINT('',(63.156506526837,-0.8,-68.39));
#55607=CARTESIAN_POINT('Origin',(59.11,-0.8,-68.39));
#55608=CARTESIAN_POINT('Origin',(64.11,-0.8,-68.39));
#55609=CARTESIAN_POINT('Origin',(59.11,-0.8,-68.39));
#55610=CARTESIAN_POINT('Origin',(60.0634934731631,-2.3,-68.39));
#55611=CARTESIAN_POINT('',(57.9809379204577,-1.32380208466934,-68.39));
#55612=CARTESIAN_POINT('',(60.0634934731631,1.0842021724855E-16,-68.39));
#55613=CARTESIAN_POINT('Origin',(63.156506526837,-2.3,-68.39));
#55614=CARTESIAN_POINT('',(63.156506526837,1.0842021724855E-16,-68.39));
#55615=CARTESIAN_POINT('',(65.2390620795424,-1.32380208466934,-68.39));
#55616=CARTESIAN_POINT('Origin',(66.8813246308841,-2.,-66.39));
#55617=CARTESIAN_POINT('',(65.7947739077334,-2.50932065147687,-68.39));
#55618=CARTESIAN_POINT('Origin',(56.338675369116,-2.,-68.39));
#55619=CARTESIAN_POINT('',(57.4252260922666,-2.50932065147687,-68.39));
#55620=CARTESIAN_POINT('Origin',(58.3856328512329,-0.460452899015424,-68.39));
#55621=CARTESIAN_POINT('Origin',(64.8343671487671,-0.460452899015424,-68.39));
#55622=CARTESIAN_POINT('Origin',(59.11,1.0842021724855E-16,-68.39));
#55623=CARTESIAN_POINT('Origin',(61.61,-4.,65.61));
#55624=CARTESIAN_POINT('Origin',(56.338675369116,-2.,65.61));
#55625=CARTESIAN_POINT('Origin',(66.8813246308841,-2.,65.61));
#55626=CARTESIAN_POINT('Origin',(61.61,-4.,69.61));
#55627=CARTESIAN_POINT('Origin',(66.8813246308841,-2.,69.61));
#55628=CARTESIAN_POINT('Origin',(56.338675369116,-2.,69.61));
#55629=CARTESIAN_POINT('Origin',(56.338675369116,-2.,65.61));
#55630=CARTESIAN_POINT('',(58.1495932410337,-2.84886775246144,65.61));
#55631=CARTESIAN_POINT('Origin',(56.338675369116,-2.,65.61));
#55632=CARTESIAN_POINT('',(58.1495932410337,-2.84886775246144,69.61));
#55633=CARTESIAN_POINT('',(58.1495932410337,-2.84886775246144,65.61));
#55634=CARTESIAN_POINT('Origin',(56.338675369116,-2.,69.61));
#55635=CARTESIAN_POINT('Origin',(66.8813246308841,-2.,67.61));
#55636=CARTESIAN_POINT('',(65.0704067589663,-2.84886775246144,69.61));
#55637=CARTESIAN_POINT('Origin',(66.8813246308841,-2.,69.61));
#55638=CARTESIAN_POINT('',(65.0704067589663,-2.84886775246144,65.61));
#55639=CARTESIAN_POINT('',(65.0704067589663,-2.84886775246144,65.61));
#55640=CARTESIAN_POINT('Origin',(66.8813246308841,-2.,65.61));
#55641=CARTESIAN_POINT('Origin',(66.8813246308841,-2.,69.61));
#55642=CARTESIAN_POINT('',(57.4252260922666,-2.50932065147687,69.61));
#55643=CARTESIAN_POINT('Origin',(56.338675369116,-2.,69.61));
#55644=CARTESIAN_POINT('',(58.7053050692247,-1.66334918565392,69.61));
#55645=CARTESIAN_POINT('',(59.11,-0.8,69.61));
#55646=CARTESIAN_POINT('',(60.0634934731631,-0.8,69.61));
#55647=CARTESIAN_POINT('Origin',(60.0634934731631,-2.3,69.61));
#55648=CARTESIAN_POINT('',(63.156506526837,-0.8,69.61));
#55649=CARTESIAN_POINT('',(59.11,-0.8,69.61));
#55650=CARTESIAN_POINT('',(64.5146949307753,-1.66334918565392,69.61));
#55651=CARTESIAN_POINT('Origin',(63.156506526837,-2.3,69.61));
#55652=CARTESIAN_POINT('',(64.11,-0.8,69.61));
#55653=CARTESIAN_POINT('',(65.7947739077334,-2.50932065147687,69.61));
#55654=CARTESIAN_POINT('Origin',(66.8813246308841,-2.,69.61));
#55655=CARTESIAN_POINT('',(65.2390620795424,-1.32380208466934,69.61));
#55656=CARTESIAN_POINT('',(64.8343671487671,-0.460452899015424,69.61));
#55657=CARTESIAN_POINT('',(63.156506526837,1.0842021724855E-16,69.61));
#55658=CARTESIAN_POINT('Origin',(63.156506526837,-2.3,69.61));
#55659=CARTESIAN_POINT('',(60.0634934731631,-4.33680868994202E-16,69.61));
#55660=CARTESIAN_POINT('',(59.11,1.0842021724855E-16,69.61));
#55661=CARTESIAN_POINT('',(57.9809379204577,-1.32380208466934,69.61));
#55662=CARTESIAN_POINT('Origin',(60.0634934731631,-2.3,69.61));
#55663=CARTESIAN_POINT('',(58.3856328512329,-0.460452899015424,69.61));
#55664=CARTESIAN_POINT('Origin',(59.11,-0.8,65.61));
#55665=CARTESIAN_POINT('',(65.7947739077334,-2.50932065147687,65.61));
#55666=CARTESIAN_POINT('Origin',(66.8813246308841,-2.,65.61));
#55667=CARTESIAN_POINT('',(64.5146949307753,-1.66334918565392,65.61));
#55668=CARTESIAN_POINT('',(64.11,-0.8,65.61));
#55669=CARTESIAN_POINT('',(63.156506526837,-0.8,65.61));
#55670=CARTESIAN_POINT('Origin',(63.156506526837,-2.3,65.61));
#55671=CARTESIAN_POINT('',(60.0634934731631,-0.8,65.61));
#55672=CARTESIAN_POINT('',(59.11,-0.8,65.61));
#55673=CARTESIAN_POINT('',(58.7053050692247,-1.66334918565392,65.61));
#55674=CARTESIAN_POINT('Origin',(60.0634934731631,-2.3,65.61));
#55675=CARTESIAN_POINT('',(59.11,-0.8,65.61));
#55676=CARTESIAN_POINT('',(57.4252260922666,-2.50932065147687,65.61));
#55677=CARTESIAN_POINT('Origin',(56.338675369116,-2.,65.61));
#55678=CARTESIAN_POINT('',(57.9809379204577,-1.32380208466934,65.61));
#55679=CARTESIAN_POINT('',(58.3856328512329,-0.460452899015424,65.61));
#55680=CARTESIAN_POINT('',(60.0634934731631,1.0842021724855E-16,65.61));
#55681=CARTESIAN_POINT('Origin',(60.0634934731631,-2.3,65.61));
#55682=CARTESIAN_POINT('',(63.156506526837,1.0842021724855E-16,65.61));
#55683=CARTESIAN_POINT('',(59.11,1.0842021724855E-16,65.61));
#55684=CARTESIAN_POINT('',(65.2390620795424,-1.32380208466934,65.61));
#55685=CARTESIAN_POINT('Origin',(63.156506526837,-2.3,65.61));
#55686=CARTESIAN_POINT('',(64.8343671487671,-0.460452899015424,65.61));
#55687=CARTESIAN_POINT('Origin',(60.0634934731631,-2.3,65.61));
#55688=CARTESIAN_POINT('',(60.0634934731631,-0.8,65.61));
#55689=CARTESIAN_POINT('',(58.7053050692247,-1.66334918565392,65.61));
#55690=CARTESIAN_POINT('Origin',(63.156506526837,-2.3,65.61));
#55691=CARTESIAN_POINT('',(64.5146949307753,-1.66334918565392,65.61));
#55692=CARTESIAN_POINT('',(63.156506526837,-0.8,65.61));
#55693=CARTESIAN_POINT('Origin',(59.11,-0.8,65.61));
#55694=CARTESIAN_POINT('Origin',(64.11,-0.8,65.61));
#55695=CARTESIAN_POINT('Origin',(59.11,-0.8,65.61));
#55696=CARTESIAN_POINT('Origin',(60.0634934731631,-2.3,65.61));
#55697=CARTESIAN_POINT('',(57.9809379204577,-1.32380208466934,65.61));
#55698=CARTESIAN_POINT('',(60.0634934731631,1.0842021724855E-16,65.61));
#55699=CARTESIAN_POINT('Origin',(63.156506526837,-2.3,65.61));
#55700=CARTESIAN_POINT('',(63.156506526837,1.0842021724855E-16,65.61));
#55701=CARTESIAN_POINT('',(65.2390620795424,-1.32380208466934,65.61));
#55702=CARTESIAN_POINT('Origin',(66.8813246308841,-2.,67.61));
#55703=CARTESIAN_POINT('',(65.7947739077334,-2.50932065147687,65.61));
#55704=CARTESIAN_POINT('Origin',(56.338675369116,-2.,65.61));
#55705=CARTESIAN_POINT('',(57.4252260922666,-2.50932065147687,65.61));
#55706=CARTESIAN_POINT('Origin',(58.3856328512329,-0.460452899015424,65.61));
#55707=CARTESIAN_POINT('Origin',(64.8343671487671,-0.460452899015424,65.61));
#55708=CARTESIAN_POINT('Origin',(59.11,1.0842021724855E-16,65.61));
#55709=CARTESIAN_POINT('Origin',(-48.39,-4.,65.61));
#55710=CARTESIAN_POINT('Origin',(-53.661324630884,-2.,65.61));
#55711=CARTESIAN_POINT('Origin',(-43.1186753691159,-2.,65.61));
#55712=CARTESIAN_POINT('Origin',(-48.39,-4.,69.61));
#55713=CARTESIAN_POINT('Origin',(-43.1186753691159,-2.,69.61));
#55714=CARTESIAN_POINT('Origin',(-53.661324630884,-2.,69.61));
#55715=CARTESIAN_POINT('Origin',(-53.661324630884,-2.,65.61));
#55716=CARTESIAN_POINT('',(-51.8504067589663,-2.84886775246144,65.61));
#55717=CARTESIAN_POINT('Origin',(-53.661324630884,-2.,65.61));
#55718=CARTESIAN_POINT('',(-51.8504067589663,-2.84886775246144,69.61));
#55719=CARTESIAN_POINT('',(-51.8504067589663,-2.84886775246144,65.61));
#55720=CARTESIAN_POINT('Origin',(-53.661324630884,-2.,69.61));
#55721=CARTESIAN_POINT('Origin',(-43.1186753691159,-2.,67.61));
#55722=CARTESIAN_POINT('',(-44.9295932410337,-2.84886775246144,69.61));
#55723=CARTESIAN_POINT('Origin',(-43.1186753691159,-2.,69.61));
#55724=CARTESIAN_POINT('',(-44.9295932410337,-2.84886775246144,65.61));
#55725=CARTESIAN_POINT('',(-44.9295932410337,-2.84886775246144,65.61));
#55726=CARTESIAN_POINT('Origin',(-43.1186753691159,-2.,65.61));
#55727=CARTESIAN_POINT('Origin',(-43.1186753691159,-2.,69.61));
#55728=CARTESIAN_POINT('',(-52.5747739077334,-2.50932065147687,69.61));
#55729=CARTESIAN_POINT('Origin',(-53.661324630884,-2.,69.61));
#55730=CARTESIAN_POINT('',(-51.2946949307753,-1.66334918565392,69.61));
#55731=CARTESIAN_POINT('',(-50.89,-0.8,69.61));
#55732=CARTESIAN_POINT('',(-49.9365065268369,-0.8,69.61));
#55733=CARTESIAN_POINT('Origin',(-49.9365065268369,-2.3,69.61));
#55734=CARTESIAN_POINT('',(-46.843493473163,-0.8,69.61));
#55735=CARTESIAN_POINT('',(-50.89,-0.8,69.61));
#55736=CARTESIAN_POINT('',(-45.4853050692247,-1.66334918565392,69.61));
#55737=CARTESIAN_POINT('Origin',(-46.843493473163,-2.3,69.61));
#55738=CARTESIAN_POINT('',(-45.89,-0.8,69.61));
#55739=CARTESIAN_POINT('',(-44.2052260922666,-2.50932065147687,69.61));
#55740=CARTESIAN_POINT('Origin',(-43.1186753691159,-2.,69.61));
#55741=CARTESIAN_POINT('',(-44.7609379204576,-1.32380208466934,69.61));
#55742=CARTESIAN_POINT('',(-45.1656328512329,-0.460452899015424,69.61));
#55743=CARTESIAN_POINT('',(-46.843493473163,1.0842021724855E-16,69.61));
#55744=CARTESIAN_POINT('Origin',(-46.843493473163,-2.3,69.61));
#55745=CARTESIAN_POINT('',(-49.9365065268369,-4.33680868994202E-16,69.61));
#55746=CARTESIAN_POINT('',(-50.89,1.0842021724855E-16,69.61));
#55747=CARTESIAN_POINT('',(-52.0190620795423,-1.32380208466934,69.61));
#55748=CARTESIAN_POINT('Origin',(-49.9365065268369,-2.3,69.61));
#55749=CARTESIAN_POINT('',(-51.6143671487671,-0.460452899015424,69.61));
#55750=CARTESIAN_POINT('Origin',(-50.89,-0.8,65.61));
#55751=CARTESIAN_POINT('',(-44.2052260922666,-2.50932065147686,65.61));
#55752=CARTESIAN_POINT('Origin',(-43.1186753691159,-2.,65.61));
#55753=CARTESIAN_POINT('',(-45.4853050692247,-1.66334918565392,65.61));
#55754=CARTESIAN_POINT('',(-45.89,-0.8,65.61));
#55755=CARTESIAN_POINT('',(-46.843493473163,-0.8,65.61));
#55756=CARTESIAN_POINT('Origin',(-46.843493473163,-2.3,65.61));
#55757=CARTESIAN_POINT('',(-49.9365065268369,-0.8,65.61));
#55758=CARTESIAN_POINT('',(-50.89,-0.8,65.61));
#55759=CARTESIAN_POINT('',(-51.2946949307753,-1.66334918565392,65.61));
#55760=CARTESIAN_POINT('Origin',(-49.9365065268369,-2.3,65.61));
#55761=CARTESIAN_POINT('',(-50.89,-0.8,65.61));
#55762=CARTESIAN_POINT('',(-52.5747739077334,-2.50932065147687,65.61));
#55763=CARTESIAN_POINT('Origin',(-53.661324630884,-2.,65.61));
#55764=CARTESIAN_POINT('',(-52.0190620795423,-1.32380208466934,65.61));
#55765=CARTESIAN_POINT('',(-51.6143671487671,-0.460452899015424,65.61));
#55766=CARTESIAN_POINT('',(-49.9365065268369,1.0842021724855E-16,65.61));
#55767=CARTESIAN_POINT('Origin',(-49.9365065268369,-2.3,65.61));
#55768=CARTESIAN_POINT('',(-46.843493473163,1.0842021724855E-16,65.61));
#55769=CARTESIAN_POINT('',(-50.89,1.0842021724855E-16,65.61));
#55770=CARTESIAN_POINT('',(-44.7609379204576,-1.32380208466934,65.61));
#55771=CARTESIAN_POINT('Origin',(-46.843493473163,-2.3,65.61));
#55772=CARTESIAN_POINT('',(-45.1656328512329,-0.460452899015424,65.61));
#55773=CARTESIAN_POINT('Origin',(-49.9365065268369,-2.3,65.61));
#55774=CARTESIAN_POINT('',(-49.9365065268369,-0.8,65.61));
#55775=CARTESIAN_POINT('',(-51.2946949307753,-1.66334918565392,65.61));
#55776=CARTESIAN_POINT('Origin',(-46.843493473163,-2.3,65.61));
#55777=CARTESIAN_POINT('',(-45.4853050692247,-1.66334918565392,65.61));
#55778=CARTESIAN_POINT('',(-46.843493473163,-0.8,65.61));
#55779=CARTESIAN_POINT('Origin',(-50.89,-0.8,65.61));
#55780=CARTESIAN_POINT('Origin',(-45.89,-0.8,65.61));
#55781=CARTESIAN_POINT('Origin',(-50.89,-0.8,65.61));
#55782=CARTESIAN_POINT('Origin',(-49.9365065268369,-2.3,65.61));
#55783=CARTESIAN_POINT('',(-52.0190620795423,-1.32380208466934,65.61));
#55784=CARTESIAN_POINT('',(-49.9365065268369,1.0842021724855E-16,65.61));
#55785=CARTESIAN_POINT('Origin',(-46.843493473163,-2.3,65.61));
#55786=CARTESIAN_POINT('',(-46.843493473163,1.0842021724855E-16,65.61));
#55787=CARTESIAN_POINT('',(-44.7609379204576,-1.32380208466934,65.61));
#55788=CARTESIAN_POINT('Origin',(-43.1186753691159,-2.,67.61));
#55789=CARTESIAN_POINT('',(-44.2052260922666,-2.50932065147687,65.61));
#55790=CARTESIAN_POINT('Origin',(-53.661324630884,-2.,65.61));
#55791=CARTESIAN_POINT('',(-52.5747739077334,-2.50932065147687,65.61));
#55792=CARTESIAN_POINT('Origin',(-51.6143671487671,-0.460452899015424,65.61));
#55793=CARTESIAN_POINT('Origin',(-45.1656328512329,-0.460452899015424,65.61));
#55794=CARTESIAN_POINT('Origin',(-50.89,1.0842021724855E-16,65.61));
#55795=CARTESIAN_POINT('Origin',(-48.39,-4.,-68.39));
#55796=CARTESIAN_POINT('Origin',(-53.661324630884,-2.,-68.39));
#55797=CARTESIAN_POINT('Origin',(-43.1186753691159,-2.,-68.39));
#55798=CARTESIAN_POINT('Origin',(-48.39,-4.,-64.39));
#55799=CARTESIAN_POINT('Origin',(-43.1186753691159,-2.,-64.39));
#55800=CARTESIAN_POINT('Origin',(-53.661324630884,-2.,-64.39));
#55801=CARTESIAN_POINT('Origin',(-53.661324630884,-2.,-68.39));
#55802=CARTESIAN_POINT('',(-51.8504067589663,-2.84886775246144,-68.39));
#55803=CARTESIAN_POINT('Origin',(-53.661324630884,-2.,-68.39));
#55804=CARTESIAN_POINT('',(-51.8504067589663,-2.84886775246144,-64.39));
#55805=CARTESIAN_POINT('',(-51.8504067589663,-2.84886775246144,-68.39));
#55806=CARTESIAN_POINT('Origin',(-53.661324630884,-2.,-64.39));
#55807=CARTESIAN_POINT('Origin',(-43.1186753691159,-2.,-66.39));
#55808=CARTESIAN_POINT('',(-44.9295932410337,-2.84886775246144,-64.39));
#55809=CARTESIAN_POINT('Origin',(-43.1186753691159,-2.,-64.39));
#55810=CARTESIAN_POINT('',(-44.9295932410337,-2.84886775246144,-68.39));
#55811=CARTESIAN_POINT('',(-44.9295932410337,-2.84886775246144,-68.39));
#55812=CARTESIAN_POINT('Origin',(-43.1186753691159,-2.,-68.39));
#55813=CARTESIAN_POINT('Origin',(-43.1186753691159,-2.,-64.39));
#55814=CARTESIAN_POINT('',(-52.5747739077334,-2.50932065147687,-64.39));
#55815=CARTESIAN_POINT('Origin',(-53.661324630884,-2.,-64.39));
#55816=CARTESIAN_POINT('',(-51.2946949307753,-1.66334918565392,-64.39));
#55817=CARTESIAN_POINT('',(-50.89,-0.8,-64.39));
#55818=CARTESIAN_POINT('',(-49.936506526837,-0.8,-64.39));
#55819=CARTESIAN_POINT('Origin',(-49.936506526837,-2.3,-64.39));
#55820=CARTESIAN_POINT('',(-46.843493473163,-0.8,-64.39));
#55821=CARTESIAN_POINT('',(-50.89,-0.8,-64.39));
#55822=CARTESIAN_POINT('',(-45.4853050692247,-1.66334918565392,-64.39));
#55823=CARTESIAN_POINT('Origin',(-46.843493473163,-2.3,-64.39));
#55824=CARTESIAN_POINT('',(-45.89,-0.8,-64.39));
#55825=CARTESIAN_POINT('',(-44.2052260922666,-2.50932065147687,-64.39));
#55826=CARTESIAN_POINT('Origin',(-43.1186753691159,-2.,-64.39));
#55827=CARTESIAN_POINT('',(-44.7609379204576,-1.32380208466934,-64.39));
#55828=CARTESIAN_POINT('',(-45.1656328512329,-0.460452899015424,-64.39));
#55829=CARTESIAN_POINT('',(-46.843493473163,1.0842021724855E-16,-64.39));
#55830=CARTESIAN_POINT('Origin',(-46.843493473163,-2.3,-64.39));
#55831=CARTESIAN_POINT('',(-49.936506526837,-4.33680868994202E-16,-64.39));
#55832=CARTESIAN_POINT('',(-50.89,1.0842021724855E-16,-64.39));
#55833=CARTESIAN_POINT('',(-52.0190620795423,-1.32380208466934,-64.39));
#55834=CARTESIAN_POINT('Origin',(-49.936506526837,-2.3,-64.39));
#55835=CARTESIAN_POINT('',(-51.6143671487671,-0.460452899015424,-64.39));
#55836=CARTESIAN_POINT('Origin',(-50.89,-0.8,-68.39));
#55837=CARTESIAN_POINT('',(-44.2052260922666,-2.50932065147686,-68.39));
#55838=CARTESIAN_POINT('Origin',(-43.1186753691159,-2.,-68.39));
#55839=CARTESIAN_POINT('',(-45.4853050692247,-1.66334918565392,-68.39));
#55840=CARTESIAN_POINT('',(-45.89,-0.8,-68.39));
#55841=CARTESIAN_POINT('',(-46.843493473163,-0.8,-68.39));
#55842=CARTESIAN_POINT('Origin',(-46.843493473163,-2.3,-68.39));
#55843=CARTESIAN_POINT('',(-49.936506526837,-0.8,-68.39));
#55844=CARTESIAN_POINT('',(-50.89,-0.8,-68.39));
#55845=CARTESIAN_POINT('',(-51.2946949307753,-1.66334918565392,-68.39));
#55846=CARTESIAN_POINT('Origin',(-49.936506526837,-2.3,-68.39));
#55847=CARTESIAN_POINT('',(-50.89,-0.8,-68.39));
#55848=CARTESIAN_POINT('',(-52.5747739077334,-2.50932065147687,-68.39));
#55849=CARTESIAN_POINT('Origin',(-53.661324630884,-2.,-68.39));
#55850=CARTESIAN_POINT('',(-52.0190620795423,-1.32380208466934,-68.39));
#55851=CARTESIAN_POINT('',(-51.6143671487671,-0.460452899015424,-68.39));
#55852=CARTESIAN_POINT('',(-49.936506526837,1.0842021724855E-16,-68.39));
#55853=CARTESIAN_POINT('Origin',(-49.936506526837,-2.3,-68.39));
#55854=CARTESIAN_POINT('',(-46.843493473163,1.0842021724855E-16,-68.39));
#55855=CARTESIAN_POINT('',(-50.89,1.0842021724855E-16,-68.39));
#55856=CARTESIAN_POINT('',(-44.7609379204576,-1.32380208466934,-68.39));
#55857=CARTESIAN_POINT('Origin',(-46.843493473163,-2.3,-68.39));
#55858=CARTESIAN_POINT('',(-45.1656328512329,-0.460452899015424,-68.39));
#55859=CARTESIAN_POINT('Origin',(-49.936506526837,-2.3,-68.39));
#55860=CARTESIAN_POINT('',(-49.936506526837,-0.8,-68.39));
#55861=CARTESIAN_POINT('',(-51.2946949307753,-1.66334918565392,-68.39));
#55862=CARTESIAN_POINT('Origin',(-46.843493473163,-2.3,-68.39));
#55863=CARTESIAN_POINT('',(-45.4853050692247,-1.66334918565392,-68.39));
#55864=CARTESIAN_POINT('',(-46.843493473163,-0.8,-68.39));
#55865=CARTESIAN_POINT('Origin',(-50.89,-0.8,-68.39));
#55866=CARTESIAN_POINT('Origin',(-45.89,-0.8,-68.39));
#55867=CARTESIAN_POINT('Origin',(-50.89,-0.8,-68.39));
#55868=CARTESIAN_POINT('Origin',(-49.936506526837,-2.3,-68.39));
#55869=CARTESIAN_POINT('',(-52.0190620795423,-1.32380208466934,-68.39));
#55870=CARTESIAN_POINT('',(-49.936506526837,1.0842021724855E-16,-68.39));
#55871=CARTESIAN_POINT('Origin',(-46.843493473163,-2.3,-68.39));
#55872=CARTESIAN_POINT('',(-46.843493473163,1.0842021724855E-16,-68.39));
#55873=CARTESIAN_POINT('',(-44.7609379204576,-1.32380208466934,-68.39));
#55874=CARTESIAN_POINT('Origin',(-43.1186753691159,-2.,-66.39));
#55875=CARTESIAN_POINT('',(-44.2052260922666,-2.50932065147687,-68.39));
#55876=CARTESIAN_POINT('Origin',(-53.661324630884,-2.,-68.39));
#55877=CARTESIAN_POINT('',(-52.5747739077334,-2.50932065147687,-68.39));
#55878=CARTESIAN_POINT('Origin',(-51.6143671487671,-0.460452899015424,-68.39));
#55879=CARTESIAN_POINT('Origin',(-45.1656328512329,-0.460452899015424,-68.39));
#55880=CARTESIAN_POINT('Origin',(-50.89,1.0842021724855E-16,-68.39));
#55881=CARTESIAN_POINT('Origin',(-86.39,44.5787611019615,-30.));
#55882=CARTESIAN_POINT('Ctrl Pts',(-86.39,44.5787611019615,-12.5));
#55883=CARTESIAN_POINT('Ctrl Pts',(-86.39,43.433398281725,-12.5));
#55884=CARTESIAN_POINT('Ctrl Pts',(-86.3900000000003,41.4793849623337,-12.6924535140054));
#55885=CARTESIAN_POINT('Ctrl Pts',(-86.3900000000001,39.5894256066326,-13.2069280492973));
#55886=CARTESIAN_POINT('Ctrl Pts',(-86.3900000000001,38.8257009252949,-13.4727301229578));
#55887=CARTESIAN_POINT('Origin',(-86.39,42.6698984466481,-20.6937528963263));
#55888=CARTESIAN_POINT('',(-86.39,46.1862026520568,-22.1631559439119));
#55889=CARTESIAN_POINT('Ctrl Pts',(-86.39,44.5787611019615,-22.));
#55890=CARTESIAN_POINT('Ctrl Pts',(-86.39,45.1023555340697,-22.));
#55891=CARTESIAN_POINT('Ctrl Pts',(-86.39,45.6259499661778,-22.0515695504083));
#55892=CARTESIAN_POINT('Ctrl Pts',(-86.3899999999998,46.1394836780905,-22.1537177567742));
#55893=CARTESIAN_POINT('Ctrl Pts',(-86.3899999999998,46.1550660227812,-22.1568172778459));
#55894=CARTESIAN_POINT('Ctrl Pts',(-86.3899999999998,46.1706391043629,-22.1599633677105));
#55895=CARTESIAN_POINT('Ctrl Pts',(-86.3899999999998,46.1862026525634,-22.1631559443817));
#55896=CARTESIAN_POINT('',(-86.39,47.7866618629516,-21.4437528963263));
#55897=CARTESIAN_POINT('Origin',(-86.39,46.487623757275,-20.6937528963263));
#55898=CARTESIAN_POINT('',(-86.39,51.1378158375422,-15.6393839483491));
#55899=CARTESIAN_POINT('',(-86.39,43.2797229962849,-29.25));
#55900=CARTESIAN_POINT('Origin',(-86.39,49.8387777318655,-14.8893839483491));
#55901=CARTESIAN_POINT('',(-86.39,61.7683968696973,-26.7187856671455));
#55902=CARTESIAN_POINT('',(-86.39,56.0151454716109,-16.7539809986688));
#55903=CARTESIAN_POINT('Ctrl Pts',(-86.39,61.7683968689589,-26.7187856673309));
#55904=CARTESIAN_POINT('Ctrl Pts',(-86.39,61.7599375519114,-26.674463640704));
#55905=CARTESIAN_POINT('Ctrl Pts',(-86.3900000000001,61.5322159292861,-25.5059524219446));
#55906=CARTESIAN_POINT('Ctrl Pts',(-86.3900000000002,60.8508742849282,-23.2598700311452));
#55907=CARTESIAN_POINT('Ctrl Pts',(-86.39,59.2232760668162,-20.2148479377946));
#55908=CARTESIAN_POINT('Ctrl Pts',(-86.39,57.4908812316947,-18.1039187234887));
#55909=CARTESIAN_POINT('Ctrl Pts',(-86.3900000000001,56.3382988733641,-17.0329646666082));
#55910=CARTESIAN_POINT('Ctrl Pts',(-86.3900000000001,56.015145471611,-16.7539809986688));
#55911=CARTESIAN_POINT('',(-86.39,53.7358855886589,-17.139395137807));
#55912=CARTESIAN_POINT('Origin',(-86.39,55.0349236943356,-17.889395137807));
#55913=CARTESIAN_POINT('',(-86.39,45.8777992076382,-30.75));
#55914=CARTESIAN_POINT('',(-86.3899999999998,52.1693515295639,-27.4736373074919));
#55915=CARTESIAN_POINT('Ctrl Pts',(-86.3899999999997,50.5618748736091,-24.6894451446548));
#55916=CARTESIAN_POINT('Ctrl Pts',(-86.3899999999997,50.8041422375712,-24.9624237973974));
#55917=CARTESIAN_POINT('Ctrl Pts',(-86.3899999999996,51.3485297861136,-25.6673520933051));
#55918=CARTESIAN_POINT('Ctrl Pts',(-86.3899999999995,51.8596181789187,-26.6235312230362));
#55919=CARTESIAN_POINT('Ctrl Pts',(-86.3899999999996,52.1092282227056,-27.2929693864679));
#55920=CARTESIAN_POINT('Ctrl Pts',(-86.3899999999996,52.1693515272627,-27.4736373005769));
#55921=CARTESIAN_POINT('',(-86.39,53.5926110635042,-28.5));
#55922=CARTESIAN_POINT('Origin',(-86.39,53.5926110635042,-27.));
#55923=CARTESIAN_POINT('',(-86.39,60.2949931567668,-28.5));
#55924=CARTESIAN_POINT('',(-86.39,-3.78600659594871E-14,-28.5));
#55925=CARTESIAN_POINT('Origin',(-86.39,60.2949931567668,-27.));
#55926=CARTESIAN_POINT('',(-86.39,56.0151454719897,-43.2460190010043));
#55927=CARTESIAN_POINT('',(-86.39,61.7683968694786,-33.2812143329271));
#55928=CARTESIAN_POINT('Ctrl Pts',(-86.3900000000001,56.0151454719897,-43.2460190010042));
#55929=CARTESIAN_POINT('Ctrl Pts',(-86.3900000000001,56.3382988733641,-42.9670353333918));
#55930=CARTESIAN_POINT('Ctrl Pts',(-86.39,57.4908812316947,-41.8960812765113));
#55931=CARTESIAN_POINT('Ctrl Pts',(-86.3899999999999,59.2232760668162,-39.7851520622054));
#55932=CARTESIAN_POINT('Ctrl Pts',(-86.3899999999999,60.8508742849283,-36.7401299688548));
#55933=CARTESIAN_POINT('Ctrl Pts',(-86.3900000000002,61.5322159292861,-34.4940475780554));
#55934=CARTESIAN_POINT('Ctrl Pts',(-86.3900000000002,61.7599375519114,-33.325536359296));
#55935=CARTESIAN_POINT('Ctrl Pts',(-86.3900000000002,61.7683968689589,-33.2812143326691));
#55936=CARTESIAN_POINT('',(-86.39,60.2949931567668,-31.5));
#55937=CARTESIAN_POINT('Origin',(-86.39,60.2949931567668,-33.));
#55938=CARTESIAN_POINT('',(-86.39,53.5926110635042,-31.5));
#55939=CARTESIAN_POINT('',(-86.39,-3.78600659594871E-14,-31.5));
#55940=CARTESIAN_POINT('',(-86.3899999999999,52.1693515289861,-32.5263626942444));
#55941=CARTESIAN_POINT('Origin',(-86.39,53.5926110635042,-32.9999999999999));
#55942=CARTESIAN_POINT('Ctrl Pts',(-86.3899999999998,52.1693515261484,-32.5263627027716));
#55943=CARTESIAN_POINT('Ctrl Pts',(-86.3899999999998,52.1092282218831,-32.7070306157379));
#55944=CARTESIAN_POINT('Ctrl Pts',(-86.3899999999998,51.8596181783615,-33.3764687780062));
#55945=CARTESIAN_POINT('Ctrl Pts',(-86.39,51.3485297861136,-34.3326479066949));
#55946=CARTESIAN_POINT('Ctrl Pts',(-86.3899999999998,50.8041422375712,-35.0375762026026));
#55947=CARTESIAN_POINT('Ctrl Pts',(-86.3899999999998,50.5618748736091,-35.3105548553452));
#55948=CARTESIAN_POINT('',(-86.39,53.7358855886589,-42.860604862193));
#55949=CARTESIAN_POINT('',(-86.39,45.8777992076382,-29.25));
#55950=CARTESIAN_POINT('Origin',(-86.39,55.0349236943356,-42.110604862193));
#55951=CARTESIAN_POINT('',(-86.39,50.3318212777197,-46.5272698779464));
#55952=CARTESIAN_POINT('Ctrl Pts',(-86.39,38.825700926836,-46.5272698775785));
#55953=CARTESIAN_POINT('Ctrl Pts',(-86.3900000000001,39.5894256076847,-46.7930719509892));
#55954=CARTESIAN_POINT('Ctrl Pts',(-86.3900000000002,41.4793849628776,-47.3075464860481));
#55955=CARTESIAN_POINT('Ctrl Pts',(-86.39,44.5787611019615,-47.6128083915182));
#55956=CARTESIAN_POINT('Ctrl Pts',(-86.3900000000003,47.6781372410454,-47.3075464860481));
#55957=CARTESIAN_POINT('Ctrl Pts',(-86.3900000000001,49.5680965962383,-46.7930719509892));
#55958=CARTESIAN_POINT('Ctrl Pts',(-86.39,50.331821277087,-46.5272698775786));
#55959=CARTESIAN_POINT('',(-86.39,51.1378158375422,-44.3606160516509));
#55960=CARTESIAN_POINT('Origin',(-86.39,49.8387777318655,-45.1106160516509));
#55961=CARTESIAN_POINT('',(-86.39,47.7866618629516,-38.5562471036737));
#55962=CARTESIAN_POINT('',(-86.39,43.2797229962849,-30.75));
#55963=CARTESIAN_POINT('',(-86.39,46.1862026523886,-37.8368440547629));
#55964=CARTESIAN_POINT('Origin',(-86.39,46.4876237572749,-39.3062471036737));
#55965=CARTESIAN_POINT('',(-86.39,42.9713195518663,-37.8368440560881));
#55966=CARTESIAN_POINT('Ctrl Pts',(-86.3899999999997,46.1862026525626,-37.8368440556185));
#55967=CARTESIAN_POINT('Ctrl Pts',(-86.3899999999997,46.1706391043624,-37.8400366322896));
#55968=CARTESIAN_POINT('Ctrl Pts',(-86.3899999999996,45.6418375870482,-37.9468656555161));
#55969=CARTESIAN_POINT('Ctrl Pts',(-86.3899999999997,44.5787611019615,-38.0515695504083));
#55970=CARTESIAN_POINT('Ctrl Pts',(-86.3899999999996,43.5156846168748,-37.9468656555161));
#55971=CARTESIAN_POINT('Ctrl Pts',(-86.3899999999997,42.9868830995607,-37.8400366322896));
#55972=CARTESIAN_POINT('Ctrl Pts',(-86.3899999999997,42.971319551943,-37.836844055738));
#55973=CARTESIAN_POINT('',(-86.39,41.3708603409714,-38.5562471036737));
#55974=CARTESIAN_POINT('Origin',(-86.39,42.6698984466481,-39.3062471036737));
#55975=CARTESIAN_POINT('',(-86.39,45.8777992076382,-30.75));
#55976=CARTESIAN_POINT('',(-86.39,33.1423767323121,-43.2460190013313));
#55977=CARTESIAN_POINT('Ctrl Pts',(-86.3900000000001,27.3891253349641,-33.281214332669));
#55978=CARTESIAN_POINT('Ctrl Pts',(-86.3900000000001,27.3975846520116,-33.3255363592959));
#55979=CARTESIAN_POINT('Ctrl Pts',(-86.3900000000001,27.6253062746369,-34.4940475780554));
#55980=CARTESIAN_POINT('Ctrl Pts',(-86.39,28.3066479189948,-36.7401299688549));
#55981=CARTESIAN_POINT('Ctrl Pts',(-86.39,29.9342461371069,-39.7851520622054));
#55982=CARTESIAN_POINT('Ctrl Pts',(-86.3900000000001,31.6666409722284,-41.8960812765113));
#55983=CARTESIAN_POINT('Ctrl Pts',(-86.3900000000001,32.8192233305589,-42.9670353333918));
#55984=CARTESIAN_POINT('Ctrl Pts',(-86.3900000000001,33.1423767323121,-43.2460190013313));
#55985=CARTESIAN_POINT('',(-86.39,35.4216366152641,-42.860604862193));
#55986=CARTESIAN_POINT('Origin',(-86.39,34.1225985095874,-42.110604862193));
#55987=CARTESIAN_POINT('',(-86.39,38.7727956517265,-37.0562271467965));
#55988=CARTESIAN_POINT('',(-86.39,43.2797229962849,-29.25));
#55989=CARTESIAN_POINT('',(-86.39,38.5956473299119,-35.3105548561393));
#55990=CARTESIAN_POINT('Origin',(-86.39,37.4737575460498,-36.3062271467965));
#55991=CARTESIAN_POINT('',(-86.3899999999999,36.9881706743592,-32.5263626925082));
#55992=CARTESIAN_POINT('Ctrl Pts',(-86.3899999999998,38.5956473303139,-35.3105548553452));
#55993=CARTESIAN_POINT('Ctrl Pts',(-86.3899999999998,38.3533799663518,-35.0375762026026));
#55994=CARTESIAN_POINT('Ctrl Pts',(-86.3899999999997,37.8089924178094,-34.3326479066949));
#55995=CARTESIAN_POINT('Ctrl Pts',(-86.3899999999999,37.2979040250044,-33.3764687769638));
#55996=CARTESIAN_POINT('Ctrl Pts',(-86.3899999999999,37.0482939812175,-32.7070306135321));
#55997=CARTESIAN_POINT('Ctrl Pts',(-86.3899999999998,36.9881706766604,-32.5263626994232));
#55998=CARTESIAN_POINT('',(-86.39,35.5649111404189,-31.5));
#55999=CARTESIAN_POINT('Origin',(-86.39,35.5649111404189,-33.));
#56000=CARTESIAN_POINT('',(-86.39,-3.78600659594871E-14,-31.5));
#56001=CARTESIAN_POINT('',(-86.39,33.1423767319333,-16.7539809989958));
#56002=CARTESIAN_POINT('Ctrl Pts',(-86.3900000000001,33.1423767319333,-16.7539809989958));
#56003=CARTESIAN_POINT('Ctrl Pts',(-86.3900000000001,32.819223330559,-17.0329646666082));
#56004=CARTESIAN_POINT('Ctrl Pts',(-86.3900000000001,31.6666409722284,-18.1039187234887));
#56005=CARTESIAN_POINT('Ctrl Pts',(-86.3899999999999,29.9342461371069,-20.2148479377946));
#56006=CARTESIAN_POINT('Ctrl Pts',(-86.3900000000004,28.3066479189948,-23.2598700311452));
#56007=CARTESIAN_POINT('Ctrl Pts',(-86.3900000000002,27.6253062746369,-25.5059524219446));
#56008=CARTESIAN_POINT('Ctrl Pts',(-86.3900000000002,27.3975846520116,-26.674463640704));
#56009=CARTESIAN_POINT('Ctrl Pts',(-86.3900000000002,27.3891253349641,-26.7187856673309));
#56010=CARTESIAN_POINT('',(-86.39,35.5649111404189,-28.5));
#56011=CARTESIAN_POINT('',(-86.39,-3.78600659594871E-14,-28.5));
#56012=CARTESIAN_POINT('',(-86.3899999999999,36.988170674937,-27.4736373057556));
#56013=CARTESIAN_POINT('Origin',(-86.39,35.5649111404189,-27.));
#56014=CARTESIAN_POINT('',(-86.39,38.5956473300202,-24.6894451439698));
#56015=CARTESIAN_POINT('Ctrl Pts',(-86.3899999999998,36.9881706777747,-27.4736372972284));
#56016=CARTESIAN_POINT('Ctrl Pts',(-86.3899999999998,37.0482939820399,-27.2929693842621));
#56017=CARTESIAN_POINT('Ctrl Pts',(-86.3899999999999,37.2979040255616,-26.6235312219938));
#56018=CARTESIAN_POINT('Ctrl Pts',(-86.3899999999997,37.8089924178094,-25.6673520933051));
#56019=CARTESIAN_POINT('Ctrl Pts',(-86.3899999999998,38.3533799663518,-24.9624237973974));
#56020=CARTESIAN_POINT('Ctrl Pts',(-86.3899999999998,38.5956473303139,-24.6894451446548));
#56021=CARTESIAN_POINT('',(-86.39,38.7727956517265,-22.9437728532035));
#56022=CARTESIAN_POINT('Origin',(-86.39,37.4737575460499,-23.6937728532035));
#56023=CARTESIAN_POINT('',(-86.39,35.4216366152641,-17.139395137807));
#56024=CARTESIAN_POINT('',(-86.39,43.2797229962849,-30.75));
#56025=CARTESIAN_POINT('Origin',(-86.39,34.1225985095875,-17.889395137807));
#56026=CARTESIAN_POINT('Ctrl Pts',(-86.39,44.5787611019615,-0.5));
#56027=CARTESIAN_POINT('Ctrl Pts',(-86.39,42.6480066335628,-0.5));
#56028=CARTESIAN_POINT('Ctrl Pts',(-86.3899999999995,38.7864976967653,-0.880325434261422));
#56029=CARTESIAN_POINT('Ctrl Pts',(-86.3899999999997,34.8506764348762,-2.07424376132674));
#56030=CARTESIAN_POINT('Ctrl Pts',(-86.3899999999997,32.8626902557638,-2.92534739713908));
#56031=CARTESIAN_POINT('Ctrl Pts',(-86.3899999999997,32.6508629759047,-3.01900602948033));
#56032=CARTESIAN_POINT('Origin',(-86.39,36.2795905006212,-9.62541485779656));
#56033=CARTESIAN_POINT('',(-86.39,52.3121016231526,-11.0146003449218));
#56034=CARTESIAN_POINT('Ctrl Pts',(-86.39,44.5787611019615,-9.5));
#56035=CARTESIAN_POINT('Ctrl Pts',(-86.39,45.9204718342386,-9.5));
#56036=CARTESIAN_POINT('Ctrl Pts',(-86.3899999999998,48.5636521071579,-9.76033053440579));
#56037=CARTESIAN_POINT('Ctrl Pts',(-86.39,51.1067797000701,-10.5236598583039));
#56038=CARTESIAN_POINT('Ctrl Pts',(-86.3900000000001,52.3121016228057,-11.0146003457735));
#56039=CARTESIAN_POINT('Origin',(-86.39,52.8779317033019,-9.62541485779658));
#56040=CARTESIAN_POINT('Origin',(-86.39,55.9000854795073,-4.39089096912261));
#56041=CARTESIAN_POINT('',(-86.39,73.9088368631419,-26.8393082747607));
#56042=CARTESIAN_POINT('',(-86.39,61.981165935949,-6.17977240953646));
#56043=CARTESIAN_POINT('Ctrl Pts',(-86.3899999999997,73.9088368640174,-26.839308274661));
#56044=CARTESIAN_POINT('Ctrl Pts',(-86.3899999999997,73.8150807723753,-25.9691649995626));
#56045=CARTESIAN_POINT('Ctrl Pts',(-86.3899999999998,73.3905329456444,-23.1927173488564));
#56046=CARTESIAN_POINT('Ctrl Pts',(-86.3899999999996,72.0088947532483,-18.6380666239304));
#56047=CARTESIAN_POINT('Ctrl Pts',(-86.3899999999996,69.2652291855737,-13.5050293808538));
#56048=CARTESIAN_POINT('Ctrl Pts',(-86.3899999999999,65.8355371052309,-9.3259374892749));
#56049=CARTESIAN_POINT('Ctrl Pts',(-86.3899999999998,63.2074283898883,-7.07576138751773));
#56050=CARTESIAN_POINT('Ctrl Pts',(-86.3899999999997,61.981165935513,-6.17977241013897));
#56051=CARTESIAN_POINT('Origin',(-86.39,61.0962221090323,-7.39091832371568));
#56052=CARTESIAN_POINT('',(-86.39,64.8871997647975,-27.2044726114797));
#56053=CARTESIAN_POINT('Ctrl Pts',(-86.39,57.1538693431349,-13.8100697594034));
#56054=CARTESIAN_POINT('Ctrl Pts',(-86.39,57.8284952042209,-14.3341115102115));
#56055=CARTESIAN_POINT('Ctrl Pts',(-86.3899999999999,59.4786368856762,-15.7895125368886));
#56056=CARTESIAN_POINT('Ctrl Pts',(-86.3899999999999,61.7337643465056,-18.5373932985594));
#56057=CARTESIAN_POINT('Ctrl Pts',(-86.3899999999998,63.6403794020083,-22.1044191793415));
#56058=CARTESIAN_POINT('Ctrl Pts',(-86.3899999999998,64.5418111191123,-25.076041306158));
#56059=CARTESIAN_POINT('Ctrl Pts',(-86.3899999999999,64.8317241957022,-26.801305653953));
#56060=CARTESIAN_POINT('Ctrl Pts',(-86.3899999999999,64.8871997647975,-27.2044726114797));
#56061=CARTESIAN_POINT('Origin',(-86.39,66.3731980659926,-27.));
#56062=CARTESIAN_POINT('Origin',(-86.39,72.4174689786827,-27.));
#56063=CARTESIAN_POINT('',(-86.39,61.9811659358818,-53.8202275903908));
#56064=CARTESIAN_POINT('',(-86.39,73.9088368645467,-33.1606917253857));
#56065=CARTESIAN_POINT('Ctrl Pts',(-86.3899999999998,61.981165935513,-53.820227589861));
#56066=CARTESIAN_POINT('Ctrl Pts',(-86.3899999999997,63.2074283898883,-52.9242386124823));
#56067=CARTESIAN_POINT('Ctrl Pts',(-86.3899999999997,65.8355371052309,-50.6740625107251));
#56068=CARTESIAN_POINT('Ctrl Pts',(-86.3899999999997,69.2652291855737,-46.4949706191462));
#56069=CARTESIAN_POINT('Ctrl Pts',(-86.39,72.0088947532483,-41.3619333760696));
#56070=CARTESIAN_POINT('Ctrl Pts',(-86.3899999999997,73.3905329456444,-36.8072826511436));
#56071=CARTESIAN_POINT('Ctrl Pts',(-86.3899999999996,73.8150807723754,-34.0308350004374));
#56072=CARTESIAN_POINT('Ctrl Pts',(-86.3899999999996,73.9088368640174,-33.1606917253389));
#56073=CARTESIAN_POINT('Origin',(-86.39,72.4174689786827,-33.));
#56074=CARTESIAN_POINT('',(-86.39,64.8871997648004,-32.7955273884995));
#56075=CARTESIAN_POINT('Origin',(-86.39,66.3731980659926,-33.));
#56076=CARTESIAN_POINT('Ctrl Pts',(-86.39,64.8871997648004,-32.7955273884995));
#56077=CARTESIAN_POINT('Ctrl Pts',(-86.39,64.8317241957022,-33.198694346047));
#56078=CARTESIAN_POINT('Ctrl Pts',(-86.3899999999999,64.5418111191122,-34.923958693842));
#56079=CARTESIAN_POINT('Ctrl Pts',(-86.3899999999999,63.6403794020083,-37.8955808206585));
#56080=CARTESIAN_POINT('Ctrl Pts',(-86.39,61.7337643465056,-41.4626067014406));
#56081=CARTESIAN_POINT('Ctrl Pts',(-86.39,59.4786368856762,-44.2104874631114));
#56082=CARTESIAN_POINT('Ctrl Pts',(-86.3899999999999,57.8284952042209,-45.6658884897885));
#56083=CARTESIAN_POINT('Ctrl Pts',(-86.3899999999999,57.1538693431349,-46.1899302405967));
#56084=CARTESIAN_POINT('Origin',(-86.39,61.0962221090322,-52.6090816762843));
#56085=CARTESIAN_POINT('',(-86.39,56.5066592283165,-56.9809939712271));
#56086=CARTESIAN_POINT('Ctrl Pts',(-86.3899999999997,32.6508629759048,-56.9809939705197));
#56087=CARTESIAN_POINT('Ctrl Pts',(-86.3899999999997,32.8626902557639,-57.074652602861));
#56088=CARTESIAN_POINT('Ctrl Pts',(-86.3899999999997,34.8506764348762,-57.9257562386733));
#56089=CARTESIAN_POINT('Ctrl Pts',(-86.39,38.7864976967653,-59.1196745657386));
#56090=CARTESIAN_POINT('Ctrl Pts',(-86.3899999999997,44.5787611019615,-59.6901627171307));
#56091=CARTESIAN_POINT('Ctrl Pts',(-86.3899999999998,50.3710245071578,-59.1196745657386));
#56092=CARTESIAN_POINT('Ctrl Pts',(-86.3899999999999,54.3068457690469,-57.9257562386733));
#56093=CARTESIAN_POINT('Ctrl Pts',(-86.3899999999999,56.2948319481591,-57.0746526028609));
#56094=CARTESIAN_POINT('Ctrl Pts',(-86.3899999999999,56.5066592280182,-56.9809939705197));
#56095=CARTESIAN_POINT('Origin',(-86.39,55.9000854795073,-55.6091090308774));
#56096=CARTESIAN_POINT('',(-86.39,52.3121016229798,-48.9853996547525));
#56097=CARTESIAN_POINT('Origin',(-86.39,52.8779317033019,-50.3745851422034));
#56098=CARTESIAN_POINT('',(-86.39,36.8454205808236,-48.9853996550999));
#56099=CARTESIAN_POINT('Ctrl Pts',(-86.3899999999999,52.3121016227473,-48.9853996542503));
#56100=CARTESIAN_POINT('Ctrl Pts',(-86.39,51.1067797000296,-49.4763401417082));
#56101=CARTESIAN_POINT('Ctrl Pts',(-86.39,48.5636521071369,-50.2396694655963));
#56102=CARTESIAN_POINT('Ctrl Pts',(-86.3899999999999,44.5787611019615,-50.6321469729213));
#56103=CARTESIAN_POINT('Ctrl Pts',(-86.3900000000001,40.5938700967862,-50.2396694655963));
#56104=CARTESIAN_POINT('Ctrl Pts',(-86.3899999999999,38.0507425038934,-49.4763401417082));
#56105=CARTESIAN_POINT('Ctrl Pts',(-86.3899999999999,36.8454205811756,-48.9853996542502));
#56106=CARTESIAN_POINT('Origin',(-86.39,36.2795905006212,-50.3745851422034));
#56107=CARTESIAN_POINT('',(-86.39,27.1763562679741,-53.8202275904635));
#56108=CARTESIAN_POINT('Ctrl Pts',(-86.3899999999997,15.2486853399057,-33.1606917253389));
#56109=CARTESIAN_POINT('Ctrl Pts',(-86.3899999999997,15.3424414315477,-34.0308350004374));
#56110=CARTESIAN_POINT('Ctrl Pts',(-86.3899999999997,15.7669892582787,-36.8072826511436));
#56111=CARTESIAN_POINT('Ctrl Pts',(-86.3899999999997,17.1486274506748,-41.3619333760696));
#56112=CARTESIAN_POINT('Ctrl Pts',(-86.3899999999996,19.8922930183494,-46.4949706191462));
#56113=CARTESIAN_POINT('Ctrl Pts',(-86.3899999999997,23.3219850986922,-50.6740625107251));
#56114=CARTESIAN_POINT('Ctrl Pts',(-86.3899999999998,25.9500938140347,-52.9242386124823));
#56115=CARTESIAN_POINT('Ctrl Pts',(-86.3899999999998,27.17635626841,-53.820227589861));
#56116=CARTESIAN_POINT('Origin',(-86.39,28.0613000948908,-52.6090816762843));
#56117=CARTESIAN_POINT('',(-86.39,32.0036528606872,-46.1899302415183));
#56118=CARTESIAN_POINT('Origin',(-86.39,31.0834721426076,-47.3745261404244));
#56119=CARTESIAN_POINT('',(-86.39,24.2703224391255,-32.7955273885202));
#56120=CARTESIAN_POINT('Ctrl Pts',(-86.39,32.0036528607881,-46.1899302405967));
#56121=CARTESIAN_POINT('Ctrl Pts',(-86.3899999999999,31.3290269997021,-45.6658884897885));
#56122=CARTESIAN_POINT('Ctrl Pts',(-86.3899999999997,29.6788853182468,-44.2104874631114));
#56123=CARTESIAN_POINT('Ctrl Pts',(-86.3899999999999,27.4237578574175,-41.4626067014406));
#56124=CARTESIAN_POINT('Ctrl Pts',(-86.3899999999996,25.5171428019148,-37.8955808206585));
#56125=CARTESIAN_POINT('Ctrl Pts',(-86.39,24.6157110848108,-34.923958693842));
#56126=CARTESIAN_POINT('Ctrl Pts',(-86.39,24.3257980082209,-33.198694346047));
#56127=CARTESIAN_POINT('Ctrl Pts',(-86.39,24.2703224391255,-32.7955273885202));
#56128=CARTESIAN_POINT('Origin',(-86.39,22.7843241379305,-33.));
#56129=CARTESIAN_POINT('',(-86.39,27.1763562680412,-6.17977240960921));
#56130=CARTESIAN_POINT('Ctrl Pts',(-86.3899999999997,27.1763562684101,-6.17977241013893));
#56131=CARTESIAN_POINT('Ctrl Pts',(-86.3899999999997,25.9500938140348,-7.0757613875177));
#56132=CARTESIAN_POINT('Ctrl Pts',(-86.3899999999997,23.3219850986922,-9.32593748927488));
#56133=CARTESIAN_POINT('Ctrl Pts',(-86.3899999999997,19.8922930183494,-13.5050293808538));
#56134=CARTESIAN_POINT('Ctrl Pts',(-86.3899999999996,17.1486274506748,-18.6380666239304));
#56135=CARTESIAN_POINT('Ctrl Pts',(-86.3899999999997,15.7669892582787,-23.1927173488564));
#56136=CARTESIAN_POINT('Ctrl Pts',(-86.3899999999997,15.3424414315477,-25.9691649995626));
#56137=CARTESIAN_POINT('Ctrl Pts',(-86.3899999999997,15.2486853399057,-26.8393082746611));
#56138=CARTESIAN_POINT('',(-86.3899999999999,24.2703224391227,-27.2044726115005));
#56139=CARTESIAN_POINT('Origin',(-86.39,22.7843241379304,-27.));
#56140=CARTESIAN_POINT('',(-86.39,32.0036528607432,-13.8100697584875));
#56141=CARTESIAN_POINT('Ctrl Pts',(-86.3899999999999,24.2703224391227,-27.2044726115005));
#56142=CARTESIAN_POINT('Ctrl Pts',(-86.3899999999999,24.3257980082209,-26.801305653953));
#56143=CARTESIAN_POINT('Ctrl Pts',(-86.3899999999999,24.6157110848108,-25.076041306158));
#56144=CARTESIAN_POINT('Ctrl Pts',(-86.39,25.5171428019148,-22.1044191793415));
#56145=CARTESIAN_POINT('Ctrl Pts',(-86.3899999999999,27.4237578574175,-18.5373932985594));
#56146=CARTESIAN_POINT('Ctrl Pts',(-86.39,29.6788853182468,-15.7895125368886));
#56147=CARTESIAN_POINT('Ctrl Pts',(-86.3899999999999,31.3290269997022,-14.3341115102115));
#56148=CARTESIAN_POINT('Ctrl Pts',(-86.3899999999999,32.0036528607881,-13.8100697594033));
#56149=CARTESIAN_POINT('Origin',(-86.39,31.0834721426076,-12.6254738595756));
#56150=CARTESIAN_POINT('Origin',(-86.39,28.0613000948908,-7.39091832371568));
#56151=CARTESIAN_POINT('Origin',(-86.39,30.2431724514241,0.829967899138609));
#56152=CARTESIAN_POINT('',(-86.39,58.2818165767216,-0.530143045432115));
#56153=CARTESIAN_POINT('Ctrl Pts',(-86.39,44.5787611019615,2.5));
#56154=CARTESIAN_POINT('Ctrl Pts',(-86.3899999999999,46.7058634824009,2.5));
#56155=CARTESIAN_POINT('Ctrl Pts',(-86.3899999999999,50.9600682432795,2.08099740293233));
#56156=CARTESIAN_POINT('Ctrl Pts',(-86.39,55.4939941495213,0.705646015552456));
#56157=CARTESIAN_POINT('Ctrl Pts',(-86.39,57.863878739489,-0.335776881547477));
#56158=CARTESIAN_POINT('Ctrl Pts',(-86.39,58.2818165767217,-0.530143045432121));
#56159=CARTESIAN_POINT('Origin',(-86.39,58.914349752499,0.829967899138591));
#56160=CARTESIAN_POINT('Origin',(-86.39,61.1722800421212,4.74081788071294));
#56161=CARTESIAN_POINT('Origin',(-86.39,66.3683162853859,1.74061665201678));
#56162=CARTESIAN_POINT('',(-86.39,76.9518771320469,-27.1323759919381));
#56163=CARTESIAN_POINT('Ctrl Pts',(-86.3899999999998,63.2487659306122,-3.39775347084041));
#56164=CARTESIAN_POINT('Ctrl Pts',(-86.3899999999998,64.7867667693756,-4.47726951085139));
#56165=CARTESIAN_POINT('Ctrl Pts',(-86.39,67.8660024791148,-7.0635732469528));
#56166=CARTESIAN_POINT('Ctrl Pts',(-86.3900000000002,71.775717465263,-11.8275747416186));
#56167=CARTESIAN_POINT('Ctrl Pts',(-86.3899999999997,74.7983998703283,-17.4826157721267));
#56168=CARTESIAN_POINT('Ctrl Pts',(-86.39,76.3805781139171,-22.698358449033));
#56169=CARTESIAN_POINT('Ctrl Pts',(-86.3899999999999,76.8486238665249,-25.9669410775951));
#56170=CARTESIAN_POINT('Ctrl Pts',(-86.3899999999999,76.9518771315612,-27.1323759917098));
#56171=CARTESIAN_POINT('Origin',(-86.39,78.4460245797131,-27.));
#56172=CARTESIAN_POINT('Origin',(-86.39,82.9621121574678,-27.));
#56173=CARTESIAN_POINT('',(-86.3899999999999,67.2171661194344,-62.9773275507524));
#56174=CARTESIAN_POINT('',(-86.3899999999999,84.4575665229983,-33.1166895167565));
#56175=CARTESIAN_POINT('Ctrl Pts',(-86.3899999999999,67.2171661194344,-62.9773275507524));
#56176=CARTESIAN_POINT('Ctrl Pts',(-86.39,68.1585542512634,-62.3311804544817));
#56177=CARTESIAN_POINT('Ctrl Pts',(-86.39,70.120027043277,-60.8582491474625));
#56178=CARTESIAN_POINT('Ctrl Pts',(-86.3899999999999,72.9083073089528,-58.329286199092));
#56179=CARTESIAN_POINT('Ctrl Pts',(-86.3899999999999,75.5496661779346,-55.41704471446));
#56180=CARTESIAN_POINT('Ctrl Pts',(-86.3900000000001,77.8907325893732,-52.2581266162731));
#56181=CARTESIAN_POINT('Ctrl Pts',(-86.3899999999996,79.9131883593013,-48.8865394828812));
#56182=CARTESIAN_POINT('Ctrl Pts',(-86.3899999999997,81.5929974870803,-45.3315997101041));
#56183=CARTESIAN_POINT('Ctrl Pts',(-86.39,82.9188283169055,-41.6302351306666));
#56184=CARTESIAN_POINT('Ctrl Pts',(-86.3899999999999,83.8728260383109,-37.8158880252114));
#56185=CARTESIAN_POINT('Ctrl Pts',(-86.3899999999998,84.2979456369875,-34.9568586727847));
#56186=CARTESIAN_POINT('Ctrl Pts',(-86.3899999999998,84.4366426410887,-33.3848430749953));
#56187=CARTESIAN_POINT('Ctrl Pts',(-86.3899999999999,84.4575665229983,-33.1166895167565));
#56188=CARTESIAN_POINT('Origin',(-86.39,82.9621122252415,-33.));
#56189=CARTESIAN_POINT('',(-86.39,76.9518771320466,-32.8676240081228));
#56190=CARTESIAN_POINT('Origin',(-86.39,78.4460245797131,-33.));
#56191=CARTESIAN_POINT('Ctrl Pts',(-86.39,76.9518771315612,-32.8676240082902));
#56192=CARTESIAN_POINT('Ctrl Pts',(-86.39,76.8486238665249,-34.0330589224049));
#56193=CARTESIAN_POINT('Ctrl Pts',(-86.3900000000001,76.3805781139171,-37.301641550967));
#56194=CARTESIAN_POINT('Ctrl Pts',(-86.3899999999998,74.7983998703283,-42.5173842278733));
#56195=CARTESIAN_POINT('Ctrl Pts',(-86.3899999999998,71.7757174652631,-48.1724252583814));
#56196=CARTESIAN_POINT('Ctrl Pts',(-86.3900000000001,67.8660024791148,-52.9364267530473));
#56197=CARTESIAN_POINT('Ctrl Pts',(-86.39,64.7867667693755,-55.5227304891487));
#56198=CARTESIAN_POINT('Ctrl Pts',(-86.39,63.248765930612,-56.6022465291597));
#56199=CARTESIAN_POINT('Origin',(-86.39,66.3683162666315,-61.7406166195334));
#56200=CARTESIAN_POINT('Origin',(-86.39,61.1722799429393,-64.740817708925));
#56201=CARTESIAN_POINT('',(-86.39,58.2818165768387,-59.4698569545135));
#56202=CARTESIAN_POINT('Origin',(-86.39,58.9143497524989,-60.8299678991386));
#56203=CARTESIAN_POINT('',(-86.3899999999999,30.8757056272014,-59.4698569545679));
#56204=CARTESIAN_POINT('Ctrl Pts',(-86.39,58.2818165768387,-59.4698569545134));
#56205=CARTESIAN_POINT('Ctrl Pts',(-86.39,57.863878739489,-59.6642231184525));
#56206=CARTESIAN_POINT('Ctrl Pts',(-86.39,55.4939941495213,-60.7056460155525));
#56207=CARTESIAN_POINT('Ctrl Pts',(-86.3899999999999,50.9600682432795,-62.0809974029323));
#56208=CARTESIAN_POINT('Ctrl Pts',(-86.39,44.5787611019615,-62.7095012985338));
#56209=CARTESIAN_POINT('Ctrl Pts',(-86.3900000000001,38.1974539606436,-62.0809974029323));
#56210=CARTESIAN_POINT('Ctrl Pts',(-86.3899999999999,33.6635280544017,-60.7056460155525));
#56211=CARTESIAN_POINT('Ctrl Pts',(-86.3899999999999,31.293643464434,-59.6642231184525));
#56212=CARTESIAN_POINT('Ctrl Pts',(-86.3899999999999,30.8757056272014,-59.4698569545679));
#56213=CARTESIAN_POINT('Origin',(-86.39,30.2431724514241,-60.8299678991386));
#56214=CARTESIAN_POINT('Origin',(-86.39,22.7892059208967,-61.7406166479301));
#56215=CARTESIAN_POINT('',(-86.39,25.9087562731289,-56.6022465300058));
#56216=CARTESIAN_POINT('Origin',(-86.39,25.0470014756374,-57.8300000340158));
#56217=CARTESIAN_POINT('',(-86.39,12.2056450718761,-32.8676240080646));
#56218=CARTESIAN_POINT('Ctrl Pts',(-86.3899999999997,25.9087562733108,-56.6022465291596));
#56219=CARTESIAN_POINT('Ctrl Pts',(-86.3899999999997,24.3707554345474,-55.5227304891486));
#56220=CARTESIAN_POINT('Ctrl Pts',(-86.3899999999997,21.2915197248082,-52.9364267530472));
#56221=CARTESIAN_POINT('Ctrl Pts',(-86.3900000000001,17.38180473866,-48.1724252583814));
#56222=CARTESIAN_POINT('Ctrl Pts',(-86.39,14.3591223335948,-42.5173842278733));
#56223=CARTESIAN_POINT('Ctrl Pts',(-86.3899999999999,12.776944090006,-37.301641550967));
#56224=CARTESIAN_POINT('Ctrl Pts',(-86.3899999999998,12.3088983373981,-34.0330589224049));
#56225=CARTESIAN_POINT('Ctrl Pts',(-86.3899999999998,12.2056450723618,-32.8676240082902));
#56226=CARTESIAN_POINT('Origin',(-86.39,10.7114976242099,-33.));
#56227=CARTESIAN_POINT('',(-86.39,12.2056450718764,-27.13237599188));
#56228=CARTESIAN_POINT('Origin',(-86.39,10.7114976242099,-27.));
#56229=CARTESIAN_POINT('',(-86.39,25.9087562731469,-3.39775347015071));
#56230=CARTESIAN_POINT('Ctrl Pts',(-86.3899999999999,12.2056450723618,-27.1323759917097));
#56231=CARTESIAN_POINT('Ctrl Pts',(-86.3899999999999,12.3088983373981,-25.966941077595));
#56232=CARTESIAN_POINT('Ctrl Pts',(-86.3899999999999,12.776944090006,-22.698358449033));
#56233=CARTESIAN_POINT('Ctrl Pts',(-86.39,14.3591223335948,-17.4826157721267));
#56234=CARTESIAN_POINT('Ctrl Pts',(-86.3899999999999,17.38180473866,-11.8275747416186));
#56235=CARTESIAN_POINT('Ctrl Pts',(-86.39,21.2915197248083,-7.06357324695279));
#56236=CARTESIAN_POINT('Ctrl Pts',(-86.39,24.3707554345475,-4.47726951085134));
#56237=CARTESIAN_POINT('Ctrl Pts',(-86.39,25.9087562733109,-3.39775347084034));
#56238=CARTESIAN_POINT('Origin',(-86.39,25.0470014756374,-2.16999996598413));
#56239=CARTESIAN_POINT('Origin',(-86.39,22.789205939653,1.74061661544304));
#56240=CARTESIAN_POINT('Ctrl Pts',(-85.5899999999998,84.4575665229977,-33.1166895167634));
#56241=CARTESIAN_POINT('Ctrl Pts',(-86.55,84.4575665229977,-33.1166895167634));
#56242=CARTESIAN_POINT('Ctrl Pts',(-85.5899999999998,84.4366426410883,-33.3848430749998));
#56243=CARTESIAN_POINT('Ctrl Pts',(-86.55,84.4366426410883,-33.3848430749998));
#56244=CARTESIAN_POINT('Ctrl Pts',(-85.5899999999997,84.2979456369872,-34.9568586727869));
#56245=CARTESIAN_POINT('Ctrl Pts',(-86.55,84.2979456369872,-34.9568586727869));
#56246=CARTESIAN_POINT('Ctrl Pts',(-85.5899999999998,83.8728260383109,-37.8158880252114));
#56247=CARTESIAN_POINT('Ctrl Pts',(-86.55,83.8728260383109,-37.8158880252114));
#56248=CARTESIAN_POINT('Ctrl Pts',(-85.59,82.9188283169055,-41.6302351306666));
#56249=CARTESIAN_POINT('Ctrl Pts',(-86.5500000000002,82.9188283169055,-41.6302351306666));
#56250=CARTESIAN_POINT('Ctrl Pts',(-85.5899999999997,81.5929974870803,-45.3315997101041));
#56251=CARTESIAN_POINT('Ctrl Pts',(-86.5499999999999,81.5929974870803,-45.3315997101041));
#56252=CARTESIAN_POINT('Ctrl Pts',(-85.5899999999996,79.9131883593013,-48.8865394828812));
#56253=CARTESIAN_POINT('Ctrl Pts',(-86.5499999999998,79.9131883593013,-48.8865394828812));
#56254=CARTESIAN_POINT('Ctrl Pts',(-85.5900000000001,77.8907325893732,-52.2581266162731));
#56255=CARTESIAN_POINT('Ctrl Pts',(-86.5500000000003,77.8907325893732,-52.2581266162731));
#56256=CARTESIAN_POINT('Ctrl Pts',(-85.5899999999998,75.5496661779346,-55.41704471446));
#56257=CARTESIAN_POINT('Ctrl Pts',(-86.55,75.5496661779346,-55.41704471446));
#56258=CARTESIAN_POINT('Ctrl Pts',(-85.5899999999998,72.9083073089528,-58.329286199092));
#56259=CARTESIAN_POINT('Ctrl Pts',(-86.55,72.9083073089528,-58.329286199092));
#56260=CARTESIAN_POINT('Ctrl Pts',(-85.5899999999999,70.1200270432783,-60.8582491474613));
#56261=CARTESIAN_POINT('Ctrl Pts',(-86.5500000000002,70.1200270432783,-60.8582491474613));
#56262=CARTESIAN_POINT('Ctrl Pts',(-85.59,68.1585542512663,-62.3311804544795));
#56263=CARTESIAN_POINT('Ctrl Pts',(-86.5500000000002,68.1585542512663,-62.3311804544795));
#56264=CARTESIAN_POINT('Ctrl Pts',(-85.5899999999999,67.2171661194389,-62.9773275507493));
#56265=CARTESIAN_POINT('Ctrl Pts',(-86.5500000000001,67.2171661194389,-62.9773275507493));
#56266=CARTESIAN_POINT('',(-86.39,67.2171661194344,-62.9773275507524));
#56267=CARTESIAN_POINT('',(-85.5899999999996,84.4575665229983,-33.1166895167565));
#56268=CARTESIAN_POINT('Origin',(913.61,45.8777992076386,-29.25));
#56269=CARTESIAN_POINT('',(-86.3900000000002,53.7358855886589,-42.860604862193));
#56270=CARTESIAN_POINT('Origin',(913.61,43.2797229962853,-30.75));
#56271=CARTESIAN_POINT('',(-85.5899999999994,51.1378158375422,-44.3606160516509));
#56272=CARTESIAN_POINT('',(-86.39,47.7866618629516,-38.5562471036737));
#56273=CARTESIAN_POINT('Origin',(913.61,45.8777992076386,-30.75));
#56274=CARTESIAN_POINT('',(-85.5899999999993,41.3708603409714,-38.5562471036737));
#56275=CARTESIAN_POINT('Origin',(913.61,43.2797229962853,-29.25));
#56276=CARTESIAN_POINT('',(-85.5899999999993,35.4216366152641,-42.860604862193));
#56277=CARTESIAN_POINT('',(-86.3899999999997,38.7727956517265,-37.0562271467965));
#56278=CARTESIAN_POINT('Origin',(913.61,4.00385864813601E-13,-31.5));
#56279=CARTESIAN_POINT('',(-85.5899999999992,35.5649111404189,-31.5));
#56280=CARTESIAN_POINT('Origin',(913.61,4.00385864813601E-13,-28.5));
#56281=CARTESIAN_POINT('',(-86.3899999999997,35.5649111404189,-28.5));
#56282=CARTESIAN_POINT('Origin',(913.61,43.2797229962853,-30.75));
#56283=CARTESIAN_POINT('',(-86.3900000000002,35.4216366152641,-17.139395137807));
#56284=CARTESIAN_POINT('',(-85.5899999999991,38.7727956517265,-22.9437728532035));
#56285=CARTESIAN_POINT('Origin',(913.61,43.2797229962853,-29.25));
#56286=CARTESIAN_POINT('',(-86.3900000000004,51.1378158375422,-15.6393839483491));
#56287=CARTESIAN_POINT('',(-85.5899999999988,47.7866618629516,-21.4437528963263));
#56288=CARTESIAN_POINT('Origin',(913.61,45.8777992076386,-30.75));
#56289=CARTESIAN_POINT('',(-85.5899999999994,53.7358855886589,-17.139395137807));
#56290=CARTESIAN_POINT('Origin',(913.61,4.00385864813601E-13,-28.5));
#56291=CARTESIAN_POINT('',(-86.3900000000002,60.2949931567668,-28.5));
#56292=CARTESIAN_POINT('',(-85.5899999999991,53.5926110635042,-28.5));
#56293=CARTESIAN_POINT('Origin',(913.61,4.00385864813601E-13,-31.5));
#56294=CARTESIAN_POINT('',(-86.39,53.5926110635042,-31.5));
#56295=CARTESIAN_POINT('',(-85.5899999999993,60.2949931567668,-31.5));
#56296=CARTESIAN_POINT('Ctrl Pts',(-85.5899999999998,61.981165935513,-53.820227589861));
#56297=CARTESIAN_POINT('Ctrl Pts',(-86.55,61.981165935513,-53.820227589861));
#56298=CARTESIAN_POINT('Ctrl Pts',(-85.5899999999998,63.2074283898883,-52.9242386124823));
#56299=CARTESIAN_POINT('Ctrl Pts',(-86.55,63.2074283898883,-52.9242386124823));
#56300=CARTESIAN_POINT('Ctrl Pts',(-85.5899999999998,65.8355371052309,-50.6740625107251));
#56301=CARTESIAN_POINT('Ctrl Pts',(-86.55,65.8355371052309,-50.6740625107251));
#56302=CARTESIAN_POINT('Ctrl Pts',(-85.5899999999998,69.2652291855737,-46.4949706191462));
#56303=CARTESIAN_POINT('Ctrl Pts',(-86.55,69.2652291855737,-46.4949706191462));
#56304=CARTESIAN_POINT('Ctrl Pts',(-85.5900000000001,72.0088947532483,-41.3619333760696));
#56305=CARTESIAN_POINT('Ctrl Pts',(-86.5500000000002,72.0088947532483,-41.3619333760696));
#56306=CARTESIAN_POINT('Ctrl Pts',(-85.5899999999998,73.3905329456444,-36.8072826511436));
#56307=CARTESIAN_POINT('Ctrl Pts',(-86.5499999999999,73.3905329456444,-36.8072826511436));
#56308=CARTESIAN_POINT('Ctrl Pts',(-85.5899999999997,73.8150807723754,-34.0308350004374));
#56309=CARTESIAN_POINT('Ctrl Pts',(-86.5499999999998,73.8150807723754,-34.0308350004374));
#56310=CARTESIAN_POINT('Ctrl Pts',(-85.5899999999997,73.9088368640174,-33.1606917253389));
#56311=CARTESIAN_POINT('Ctrl Pts',(-86.5499999999998,73.9088368640174,-33.1606917253389));
#56312=CARTESIAN_POINT('',(-85.59,73.9088368640223,-33.1606917252932));
#56313=CARTESIAN_POINT('',(-86.3899999999997,61.9811659354668,-53.8202275898948));
#56314=CARTESIAN_POINT('Ctrl Pts',(-85.5899999999998,76.9518771315612,-32.8676240082902));
#56315=CARTESIAN_POINT('Ctrl Pts',(-86.5500000000002,76.9518771315612,-32.8676240082902));
#56316=CARTESIAN_POINT('Ctrl Pts',(-85.5899999999999,76.8486238665249,-34.0330589224049));
#56317=CARTESIAN_POINT('Ctrl Pts',(-86.5500000000002,76.8486238665249,-34.0330589224049));
#56318=CARTESIAN_POINT('Ctrl Pts',(-85.59,76.3805781139171,-37.301641550967));
#56319=CARTESIAN_POINT('Ctrl Pts',(-86.5500000000004,76.3805781139171,-37.301641550967));
#56320=CARTESIAN_POINT('Ctrl Pts',(-85.5899999999997,74.7983998703283,-42.5173842278733));
#56321=CARTESIAN_POINT('Ctrl Pts',(-86.5500000000001,74.7983998703283,-42.5173842278733));
#56322=CARTESIAN_POINT('Ctrl Pts',(-85.5899999999997,71.7757174652631,-48.1724252583814));
#56323=CARTESIAN_POINT('Ctrl Pts',(-86.5500000000001,71.7757174652631,-48.1724252583814));
#56324=CARTESIAN_POINT('Ctrl Pts',(-85.5899999999999,67.8660024791148,-52.9364267530473));
#56325=CARTESIAN_POINT('Ctrl Pts',(-86.5500000000003,67.8660024791148,-52.9364267530473));
#56326=CARTESIAN_POINT('Ctrl Pts',(-85.5899999999999,64.7867667693755,-55.5227304891487));
#56327=CARTESIAN_POINT('Ctrl Pts',(-86.5500000000002,64.7867667693755,-55.5227304891487));
#56328=CARTESIAN_POINT('Ctrl Pts',(-85.5899999999999,63.248765930612,-56.6022465291597));
#56329=CARTESIAN_POINT('Ctrl Pts',(-86.5500000000002,63.248765930612,-56.6022465291597));
#56330=CARTESIAN_POINT('',(-86.39,76.9518771315567,-32.8676240083405));
#56331=CARTESIAN_POINT('Ctrl Pts',(-85.59,73.9088368640174,-26.839308274661));
#56332=CARTESIAN_POINT('Ctrl Pts',(-86.5499999999999,73.9088368640174,-26.839308274661));
#56333=CARTESIAN_POINT('Ctrl Pts',(-85.59,73.8150807723753,-25.9691649995626));
#56334=CARTESIAN_POINT('Ctrl Pts',(-86.5499999999999,73.8150807723753,-25.9691649995626));
#56335=CARTESIAN_POINT('Ctrl Pts',(-85.5900000000001,73.3905329456444,-23.1927173488564));
#56336=CARTESIAN_POINT('Ctrl Pts',(-86.55,73.3905329456444,-23.1927173488564));
#56337=CARTESIAN_POINT('Ctrl Pts',(-85.59,72.0088947532483,-18.6380666239304));
#56338=CARTESIAN_POINT('Ctrl Pts',(-86.5499999999999,72.0088947532483,-18.6380666239304));
#56339=CARTESIAN_POINT('Ctrl Pts',(-85.59,69.2652291855737,-13.5050293808538));
#56340=CARTESIAN_POINT('Ctrl Pts',(-86.5499999999999,69.2652291855737,-13.5050293808538));
#56341=CARTESIAN_POINT('Ctrl Pts',(-85.5900000000002,65.8355371052309,-9.3259374892749));
#56342=CARTESIAN_POINT('Ctrl Pts',(-86.5500000000002,65.8355371052309,-9.3259374892749));
#56343=CARTESIAN_POINT('Ctrl Pts',(-85.5900000000001,63.2074283898883,-7.07576138751773));
#56344=CARTESIAN_POINT('Ctrl Pts',(-86.55,63.2074283898883,-7.07576138751773));
#56345=CARTESIAN_POINT('Ctrl Pts',(-85.5900000000001,61.981165935513,-6.17977241013897));
#56346=CARTESIAN_POINT('Ctrl Pts',(-86.55,61.981165935513,-6.17977241013897));
#56347=CARTESIAN_POINT('',(-85.5900000000001,61.9811659354668,-6.1797724101052));
#56348=CARTESIAN_POINT('',(-86.3899999999997,73.9088368640223,-26.8393082747068));
#56349=CARTESIAN_POINT('Ctrl Pts',(-85.5899999999999,63.2487659306122,-3.39775347084041));
#56350=CARTESIAN_POINT('Ctrl Pts',(-86.5500000000002,63.2487659306122,-3.39775347084041));
#56351=CARTESIAN_POINT('Ctrl Pts',(-85.5899999999999,64.7867667693756,-4.47726951085139));
#56352=CARTESIAN_POINT('Ctrl Pts',(-86.5500000000002,64.7867667693756,-4.47726951085139));
#56353=CARTESIAN_POINT('Ctrl Pts',(-85.5900000000001,67.8660024791148,-7.0635732469528));
#56354=CARTESIAN_POINT('Ctrl Pts',(-86.5500000000004,67.8660024791148,-7.0635732469528));
#56355=CARTESIAN_POINT('Ctrl Pts',(-85.5900000000003,71.775717465263,-11.8275747416186));
#56356=CARTESIAN_POINT('Ctrl Pts',(-86.5500000000006,71.775717465263,-11.8275747416186));
#56357=CARTESIAN_POINT('Ctrl Pts',(-85.5899999999998,74.7983998703283,-17.4826157721267));
#56358=CARTESIAN_POINT('Ctrl Pts',(-86.5500000000002,74.7983998703283,-17.4826157721267));
#56359=CARTESIAN_POINT('Ctrl Pts',(-85.5900000000001,76.3805781139171,-22.698358449033));
#56360=CARTESIAN_POINT('Ctrl Pts',(-86.5500000000004,76.3805781139171,-22.698358449033));
#56361=CARTESIAN_POINT('Ctrl Pts',(-85.59,76.8486238665249,-25.9669410775951));
#56362=CARTESIAN_POINT('Ctrl Pts',(-86.5500000000004,76.8486238665249,-25.9669410775951));
#56363=CARTESIAN_POINT('Ctrl Pts',(-85.59,76.9518771315612,-27.1323759917098));
#56364=CARTESIAN_POINT('Ctrl Pts',(-86.5500000000003,76.9518771315612,-27.1323759917098));
#56365=CARTESIAN_POINT('',(-85.5900000000001,76.9518771315568,-27.1323759916595));
#56366=CARTESIAN_POINT('Ctrl Pts',(-85.5899999999998,44.5787611019615,-0.5));
#56367=CARTESIAN_POINT('Ctrl Pts',(-86.55,44.5787611019615,-0.5));
#56368=CARTESIAN_POINT('Ctrl Pts',(-85.5899999999998,42.6480066335628,-0.5));
#56369=CARTESIAN_POINT('Ctrl Pts',(-86.55,42.6480066335628,-0.5));
#56370=CARTESIAN_POINT('Ctrl Pts',(-85.5899999999994,38.7864976967653,-0.880325434261422));
#56371=CARTESIAN_POINT('Ctrl Pts',(-86.5499999999996,38.7864976967653,-0.880325434261422));
#56372=CARTESIAN_POINT('Ctrl Pts',(-85.5899999999995,34.8506764348762,-2.07424376132674));
#56373=CARTESIAN_POINT('Ctrl Pts',(-86.5499999999997,34.8506764348762,-2.07424376132674));
#56374=CARTESIAN_POINT('Ctrl Pts',(-85.5899999999996,32.8626902557638,-2.92534739713908));
#56375=CARTESIAN_POINT('Ctrl Pts',(-86.5499999999998,32.8626902557638,-2.92534739713908));
#56376=CARTESIAN_POINT('Ctrl Pts',(-85.5899999999996,32.6508629759047,-3.01900602948033));
#56377=CARTESIAN_POINT('Ctrl Pts',(-86.5499999999998,32.6508629759047,-3.01900602948033));
#56378=CARTESIAN_POINT('Ctrl Pts',(-85.5899999999998,44.5787611019615,2.5));
#56379=CARTESIAN_POINT('Ctrl Pts',(-86.5500000000001,44.5787611019615,2.5));
#56380=CARTESIAN_POINT('Ctrl Pts',(-85.5899999999998,46.7058634824009,2.5));
#56381=CARTESIAN_POINT('Ctrl Pts',(-86.5500000000001,46.7058634824009,2.5));
#56382=CARTESIAN_POINT('Ctrl Pts',(-85.5899999999997,50.9600682432795,2.08099740293233));
#56383=CARTESIAN_POINT('Ctrl Pts',(-86.55,50.9600682432795,2.08099740293233));
#56384=CARTESIAN_POINT('Ctrl Pts',(-85.5899999999999,55.4939941495213,0.705646015552456));
#56385=CARTESIAN_POINT('Ctrl Pts',(-86.5500000000002,55.4939941495213,0.705646015552456));
#56386=CARTESIAN_POINT('Ctrl Pts',(-85.5899999999998,57.863878739489,-0.335776881547477));
#56387=CARTESIAN_POINT('Ctrl Pts',(-86.5500000000001,57.863878739489,-0.335776881547477));
#56388=CARTESIAN_POINT('Ctrl Pts',(-85.5899999999998,58.2818165781778,-0.530143046109336));
#56389=CARTESIAN_POINT('Ctrl Pts',(-86.5500000000001,58.2818165781778,-0.530143046109336));
#56390=CARTESIAN_POINT('',(-85.5900000000001,58.2818165781183,-0.530143046081633));
#56391=CARTESIAN_POINT('Ctrl Pts',(-85.5900000000001,27.1763562684101,-6.17977241013893));
#56392=CARTESIAN_POINT('Ctrl Pts',(-86.5499999999997,27.1763562684101,-6.17977241013893));
#56393=CARTESIAN_POINT('Ctrl Pts',(-85.5900000000001,25.9500938140348,-7.0757613875177));
#56394=CARTESIAN_POINT('Ctrl Pts',(-86.5499999999997,25.9500938140348,-7.0757613875177));
#56395=CARTESIAN_POINT('Ctrl Pts',(-85.5900000000001,23.3219850986922,-9.32593748927488));
#56396=CARTESIAN_POINT('Ctrl Pts',(-86.5499999999997,23.3219850986922,-9.32593748927488));
#56397=CARTESIAN_POINT('Ctrl Pts',(-85.5900000000001,19.8922930183494,-13.5050293808538));
#56398=CARTESIAN_POINT('Ctrl Pts',(-86.5499999999997,19.8922930183494,-13.5050293808538));
#56399=CARTESIAN_POINT('Ctrl Pts',(-85.59,17.1486274506748,-18.6380666239304));
#56400=CARTESIAN_POINT('Ctrl Pts',(-86.5499999999996,17.1486274506748,-18.6380666239304));
#56401=CARTESIAN_POINT('Ctrl Pts',(-85.59,15.7669892582787,-23.1927173488564));
#56402=CARTESIAN_POINT('Ctrl Pts',(-86.5499999999996,15.7669892582787,-23.1927173488564));
#56403=CARTESIAN_POINT('Ctrl Pts',(-85.59,15.3424414315477,-25.9691649995626));
#56404=CARTESIAN_POINT('Ctrl Pts',(-86.5499999999997,15.3424414315477,-25.9691649995626));
#56405=CARTESIAN_POINT('Ctrl Pts',(-85.5900000000001,15.2486853399057,-26.8393082746611));
#56406=CARTESIAN_POINT('Ctrl Pts',(-86.5499999999997,15.2486853399057,-26.8393082746611));
#56407=CARTESIAN_POINT('',(-86.3899999999997,27.1763562684563,-6.17977241010519));
#56408=CARTESIAN_POINT('Ctrl Pts',(-85.59,12.2056450723618,-27.1323759917097));
#56409=CARTESIAN_POINT('Ctrl Pts',(-86.55,12.2056450723618,-27.1323759917097));
#56410=CARTESIAN_POINT('Ctrl Pts',(-85.59,12.3088983373981,-25.966941077595));
#56411=CARTESIAN_POINT('Ctrl Pts',(-86.55,12.3088983373981,-25.966941077595));
#56412=CARTESIAN_POINT('Ctrl Pts',(-85.59,12.776944090006,-22.698358449033));
#56413=CARTESIAN_POINT('Ctrl Pts',(-86.55,12.776944090006,-22.698358449033));
#56414=CARTESIAN_POINT('Ctrl Pts',(-85.5900000000001,14.3591223335948,-17.4826157721267));
#56415=CARTESIAN_POINT('Ctrl Pts',(-86.5500000000001,14.3591223335948,-17.4826157721267));
#56416=CARTESIAN_POINT('Ctrl Pts',(-85.59,17.38180473866,-11.8275747416186));
#56417=CARTESIAN_POINT('Ctrl Pts',(-86.55,17.38180473866,-11.8275747416186));
#56418=CARTESIAN_POINT('Ctrl Pts',(-85.5900000000001,21.2915197248083,-7.06357324695279));
#56419=CARTESIAN_POINT('Ctrl Pts',(-86.5500000000001,21.2915197248083,-7.06357324695279));
#56420=CARTESIAN_POINT('Ctrl Pts',(-85.5900000000001,24.3707554345475,-4.47726951085134));
#56421=CARTESIAN_POINT('Ctrl Pts',(-86.5500000000001,24.3707554345475,-4.47726951085134));
#56422=CARTESIAN_POINT('Ctrl Pts',(-85.5900000000001,25.9087562733109,-3.39775347084034));
#56423=CARTESIAN_POINT('Ctrl Pts',(-86.5500000000001,25.9087562733109,-3.39775347084034));
#56424=CARTESIAN_POINT('',(-86.39,12.2056450723663,-27.1323759916595));
#56425=CARTESIAN_POINT('',(-85.5900000000001,25.9087562733283,-3.39775347082815));
#56426=CARTESIAN_POINT('Ctrl Pts',(-85.59,15.2486853399057,-33.1606917253389));
#56427=CARTESIAN_POINT('Ctrl Pts',(-86.5499999999998,15.2486853399057,-33.1606917253389));
#56428=CARTESIAN_POINT('Ctrl Pts',(-85.59,15.3424414315477,-34.0308350004374));
#56429=CARTESIAN_POINT('Ctrl Pts',(-86.5499999999998,15.3424414315477,-34.0308350004374));
#56430=CARTESIAN_POINT('Ctrl Pts',(-85.59,15.7669892582787,-36.8072826511436));
#56431=CARTESIAN_POINT('Ctrl Pts',(-86.5499999999997,15.7669892582787,-36.8072826511436));
#56432=CARTESIAN_POINT('Ctrl Pts',(-85.5900000000001,17.1486274506748,-41.3619333760696));
#56433=CARTESIAN_POINT('Ctrl Pts',(-86.5499999999998,17.1486274506748,-41.3619333760696));
#56434=CARTESIAN_POINT('Ctrl Pts',(-85.59,19.8922930183494,-46.4949706191462));
#56435=CARTESIAN_POINT('Ctrl Pts',(-86.5499999999997,19.8922930183494,-46.4949706191462));
#56436=CARTESIAN_POINT('Ctrl Pts',(-85.59,23.3219850986922,-50.6740625107251));
#56437=CARTESIAN_POINT('Ctrl Pts',(-86.5499999999998,23.3219850986922,-50.6740625107251));
#56438=CARTESIAN_POINT('Ctrl Pts',(-85.5900000000001,25.9500938140347,-52.9242386124823));
#56439=CARTESIAN_POINT('Ctrl Pts',(-86.5499999999999,25.9500938140347,-52.9242386124823));
#56440=CARTESIAN_POINT('Ctrl Pts',(-85.5900000000001,27.17635626841,-53.820227589861));
#56441=CARTESIAN_POINT('Ctrl Pts',(-86.5499999999999,27.17635626841,-53.820227589861));
#56442=CARTESIAN_POINT('',(-85.5900000000001,27.1763562684562,-53.8202275898948));
#56443=CARTESIAN_POINT('Ctrl Pts',(-85.59,25.9087562733108,-56.6022465291596));
#56444=CARTESIAN_POINT('Ctrl Pts',(-86.5500000000001,25.9087562733108,-56.6022465291596));
#56445=CARTESIAN_POINT('Ctrl Pts',(-85.59,24.3707554345474,-55.5227304891486));
#56446=CARTESIAN_POINT('Ctrl Pts',(-86.5500000000001,24.3707554345474,-55.5227304891486));
#56447=CARTESIAN_POINT('Ctrl Pts',(-85.59,21.2915197248082,-52.9364267530472));
#56448=CARTESIAN_POINT('Ctrl Pts',(-86.5500000000001,21.2915197248082,-52.9364267530472));
#56449=CARTESIAN_POINT('Ctrl Pts',(-85.5900000000003,17.38180473866,-48.1724252583814));
#56450=CARTESIAN_POINT('Ctrl Pts',(-86.5500000000004,17.38180473866,-48.1724252583814));
#56451=CARTESIAN_POINT('Ctrl Pts',(-85.5900000000002,14.3591223335948,-42.5173842278733));
#56452=CARTESIAN_POINT('Ctrl Pts',(-86.5500000000003,14.3591223335948,-42.5173842278733));
#56453=CARTESIAN_POINT('Ctrl Pts',(-85.5900000000001,12.776944090006,-37.301641550967));
#56454=CARTESIAN_POINT('Ctrl Pts',(-86.5500000000002,12.776944090006,-37.301641550967));
#56455=CARTESIAN_POINT('Ctrl Pts',(-85.5900000000001,12.3088983373981,-34.0330589224049));
#56456=CARTESIAN_POINT('Ctrl Pts',(-86.5500000000002,12.3088983373981,-34.0330589224049));
#56457=CARTESIAN_POINT('Ctrl Pts',(-85.5900000000001,12.2056450723618,-32.8676240082902));
#56458=CARTESIAN_POINT('Ctrl Pts',(-86.5500000000002,12.2056450723618,-32.8676240082902));
#56459=CARTESIAN_POINT('',(-86.3899999999997,25.9087562733283,-56.6022465291718));
#56460=CARTESIAN_POINT('',(-85.5899999999997,12.2056450723663,-32.8676240083405));
#56461=CARTESIAN_POINT('Ctrl Pts',(-85.5900000000001,58.2818165781778,-59.4698569538907));
#56462=CARTESIAN_POINT('Ctrl Pts',(-86.5500000000001,58.2818165781778,-59.4698569538907));
#56463=CARTESIAN_POINT('Ctrl Pts',(-85.5900000000001,57.863878739489,-59.6642231184525));
#56464=CARTESIAN_POINT('Ctrl Pts',(-86.5500000000001,57.863878739489,-59.6642231184525));
#56465=CARTESIAN_POINT('Ctrl Pts',(-85.5900000000001,55.4939941495213,-60.7056460155525));
#56466=CARTESIAN_POINT('Ctrl Pts',(-86.5500000000001,55.4939941495213,-60.7056460155525));
#56467=CARTESIAN_POINT('Ctrl Pts',(-85.59,50.9600682432795,-62.0809974029323));
#56468=CARTESIAN_POINT('Ctrl Pts',(-86.5499999999999,50.9600682432795,-62.0809974029323));
#56469=CARTESIAN_POINT('Ctrl Pts',(-85.5900000000001,44.5787611019615,-62.7095012985338));
#56470=CARTESIAN_POINT('Ctrl Pts',(-86.55,44.5787611019615,-62.7095012985338));
#56471=CARTESIAN_POINT('Ctrl Pts',(-85.5900000000002,38.1974539606436,-62.0809974029323));
#56472=CARTESIAN_POINT('Ctrl Pts',(-86.5500000000001,38.1974539606436,-62.0809974029323));
#56473=CARTESIAN_POINT('Ctrl Pts',(-85.59,33.6635280544017,-60.7056460155525));
#56474=CARTESIAN_POINT('Ctrl Pts',(-86.55,33.6635280544017,-60.7056460155525));
#56475=CARTESIAN_POINT('Ctrl Pts',(-85.59,31.293643464434,-59.6642231184525));
#56476=CARTESIAN_POINT('Ctrl Pts',(-86.5499999999999,31.293643464434,-59.6642231184525));
#56477=CARTESIAN_POINT('Ctrl Pts',(-85.5899999999999,30.8757056257452,-59.4698569538907));
#56478=CARTESIAN_POINT('Ctrl Pts',(-86.5499999999999,30.8757056257452,-59.4698569538907));
#56479=CARTESIAN_POINT('',(-86.39,58.2818165781182,-59.4698569539184));
#56480=CARTESIAN_POINT('',(-85.5899999999998,30.8757056258048,-59.4698569539184));
#56481=CARTESIAN_POINT('Ctrl Pts',(-85.5900000000001,32.6508629759048,-56.9809939705197));
#56482=CARTESIAN_POINT('Ctrl Pts',(-86.55,32.6508629759048,-56.9809939705197));
#56483=CARTESIAN_POINT('Ctrl Pts',(-85.5900000000001,32.8626902557639,-57.074652602861));
#56484=CARTESIAN_POINT('Ctrl Pts',(-86.55,32.8626902557639,-57.074652602861));
#56485=CARTESIAN_POINT('Ctrl Pts',(-85.5900000000001,34.8506764348762,-57.9257562386733));
#56486=CARTESIAN_POINT('Ctrl Pts',(-86.55,34.8506764348762,-57.9257562386733));
#56487=CARTESIAN_POINT('Ctrl Pts',(-85.5900000000004,38.7864976967653,-59.1196745657386));
#56488=CARTESIAN_POINT('Ctrl Pts',(-86.5500000000003,38.7864976967653,-59.1196745657386));
#56489=CARTESIAN_POINT('Ctrl Pts',(-85.5900000000001,44.5787611019615,-59.6901627171307));
#56490=CARTESIAN_POINT('Ctrl Pts',(-86.5499999999999,44.5787611019615,-59.6901627171307));
#56491=CARTESIAN_POINT('Ctrl Pts',(-85.5900000000002,50.3710245071578,-59.1196745657386));
#56492=CARTESIAN_POINT('Ctrl Pts',(-86.55,50.3710245071578,-59.1196745657386));
#56493=CARTESIAN_POINT('Ctrl Pts',(-85.5900000000002,54.3068457690469,-57.9257562386733));
#56494=CARTESIAN_POINT('Ctrl Pts',(-86.5500000000001,54.3068457690469,-57.9257562386733));
#56495=CARTESIAN_POINT('Ctrl Pts',(-85.5900000000002,56.2948319481591,-57.0746526028609));
#56496=CARTESIAN_POINT('Ctrl Pts',(-86.5500000000001,56.2948319481591,-57.0746526028609));
#56497=CARTESIAN_POINT('Ctrl Pts',(-85.5900000000002,56.5066592280182,-56.9809939705197));
#56498=CARTESIAN_POINT('Ctrl Pts',(-86.5500000000001,56.5066592280182,-56.9809939705197));
#56499=CARTESIAN_POINT('',(-85.5900000000003,56.5066592279993,-56.9809939705281));
#56500=CARTESIAN_POINT('Ctrl Pts',(-85.5900000000001,56.0151454704998,-43.2460190022905));
#56501=CARTESIAN_POINT('Ctrl Pts',(-86.5500000000003,56.0151454704998,-43.2460190022905));
#56502=CARTESIAN_POINT('Ctrl Pts',(-85.5900000000001,56.3382988733641,-42.9670353333918));
#56503=CARTESIAN_POINT('Ctrl Pts',(-86.5500000000003,56.3382988733641,-42.9670353333918));
#56504=CARTESIAN_POINT('Ctrl Pts',(-85.59,57.4908812316947,-41.8960812765113));
#56505=CARTESIAN_POINT('Ctrl Pts',(-86.5500000000003,57.4908812316947,-41.8960812765113));
#56506=CARTESIAN_POINT('Ctrl Pts',(-85.59,59.2232760668162,-39.7851520622054));
#56507=CARTESIAN_POINT('Ctrl Pts',(-86.5500000000002,59.2232760668162,-39.7851520622054));
#56508=CARTESIAN_POINT('Ctrl Pts',(-85.59,60.8508742849283,-36.7401299688548));
#56509=CARTESIAN_POINT('Ctrl Pts',(-86.5500000000002,60.8508742849283,-36.7401299688548));
#56510=CARTESIAN_POINT('Ctrl Pts',(-85.5900000000002,61.5322159292861,-34.4940475780554));
#56511=CARTESIAN_POINT('Ctrl Pts',(-86.5500000000004,61.5322159292861,-34.4940475780554));
#56512=CARTESIAN_POINT('Ctrl Pts',(-85.5900000000002,61.7599375519114,-33.325536359296));
#56513=CARTESIAN_POINT('Ctrl Pts',(-86.5500000000004,61.7599375519114,-33.325536359296));
#56514=CARTESIAN_POINT('Ctrl Pts',(-85.5900000000002,61.7683968689589,-33.2812143326691));
#56515=CARTESIAN_POINT('Ctrl Pts',(-86.5500000000004,61.7683968689589,-33.2812143326691));
#56516=CARTESIAN_POINT('',(-85.5900000000001,61.7683968689589,-33.2812143326695));
#56517=CARTESIAN_POINT('',(-86.3900000000002,56.0151454704896,-43.2460190022993));
#56518=CARTESIAN_POINT('Ctrl Pts',(-85.5900000000001,64.887199765057,-32.7955273866341));
#56519=CARTESIAN_POINT('Ctrl Pts',(-86.55,64.887199765057,-32.7955273866341));
#56520=CARTESIAN_POINT('Ctrl Pts',(-85.5900000000001,64.8317241957022,-33.198694346047));
#56521=CARTESIAN_POINT('Ctrl Pts',(-86.55,64.8317241957022,-33.198694346047));
#56522=CARTESIAN_POINT('Ctrl Pts',(-85.59,64.5418111191122,-34.923958693842));
#56523=CARTESIAN_POINT('Ctrl Pts',(-86.5499999999999,64.5418111191122,-34.923958693842));
#56524=CARTESIAN_POINT('Ctrl Pts',(-85.59,63.6403794020083,-37.8955808206585));
#56525=CARTESIAN_POINT('Ctrl Pts',(-86.5499999999999,63.6403794020083,-37.8955808206585));
#56526=CARTESIAN_POINT('Ctrl Pts',(-85.5900000000001,61.7337643465056,-41.4626067014406));
#56527=CARTESIAN_POINT('Ctrl Pts',(-86.55,61.7337643465056,-41.4626067014406));
#56528=CARTESIAN_POINT('Ctrl Pts',(-85.5900000000001,59.4786368856762,-44.2104874631114));
#56529=CARTESIAN_POINT('Ctrl Pts',(-86.55,59.4786368856762,-44.2104874631114));
#56530=CARTESIAN_POINT('Ctrl Pts',(-85.59,57.8284952042209,-45.6658884897885));
#56531=CARTESIAN_POINT('Ctrl Pts',(-86.5499999999999,57.8284952042209,-45.6658884897885));
#56532=CARTESIAN_POINT('Ctrl Pts',(-85.59,57.1538693431349,-46.1899302405967));
#56533=CARTESIAN_POINT('Ctrl Pts',(-86.5499999999999,57.1538693431349,-46.1899302405967));
#56534=CARTESIAN_POINT('',(-86.3900000000002,64.8871997650542,-32.795527386655));
#56535=CARTESIAN_POINT('Ctrl Pts',(-85.5900000000003,61.7683968689589,-26.7187856673309));
#56536=CARTESIAN_POINT('Ctrl Pts',(-86.5500000000003,61.7683968689589,-26.7187856673309));
#56537=CARTESIAN_POINT('Ctrl Pts',(-85.5900000000003,61.7599375519114,-26.674463640704));
#56538=CARTESIAN_POINT('Ctrl Pts',(-86.5500000000003,61.7599375519114,-26.674463640704));
#56539=CARTESIAN_POINT('Ctrl Pts',(-85.5900000000003,61.5322159292861,-25.5059524219446));
#56540=CARTESIAN_POINT('Ctrl Pts',(-86.5500000000004,61.5322159292861,-25.5059524219446));
#56541=CARTESIAN_POINT('Ctrl Pts',(-85.5900000000004,60.8508742849282,-23.2598700311452));
#56542=CARTESIAN_POINT('Ctrl Pts',(-86.5500000000004,60.8508742849282,-23.2598700311452));
#56543=CARTESIAN_POINT('Ctrl Pts',(-85.5900000000003,59.2232760668162,-20.2148479377946));
#56544=CARTESIAN_POINT('Ctrl Pts',(-86.5500000000003,59.2232760668162,-20.2148479377946));
#56545=CARTESIAN_POINT('Ctrl Pts',(-85.5900000000002,57.4908812316947,-18.1039187234887));
#56546=CARTESIAN_POINT('Ctrl Pts',(-86.5500000000002,57.4908812316947,-18.1039187234887));
#56547=CARTESIAN_POINT('Ctrl Pts',(-85.5900000000003,56.3382988733641,-17.0329646666082));
#56548=CARTESIAN_POINT('Ctrl Pts',(-86.5500000000004,56.3382988733641,-17.0329646666082));
#56549=CARTESIAN_POINT('Ctrl Pts',(-85.5900000000004,56.0151454704999,-16.7539809977095));
#56550=CARTESIAN_POINT('Ctrl Pts',(-86.5500000000004,56.0151454704999,-16.7539809977095));
#56551=CARTESIAN_POINT('',(-85.59,56.0151454704897,-16.7539809977007));
#56552=CARTESIAN_POINT('',(-86.3900000000002,61.7683968689589,-26.7187856673305));
#56553=CARTESIAN_POINT('Ctrl Pts',(-85.5900000000001,57.1538693431349,-13.8100697594034));
#56554=CARTESIAN_POINT('Ctrl Pts',(-86.55,57.1538693431349,-13.8100697594034));
#56555=CARTESIAN_POINT('Ctrl Pts',(-85.5900000000001,57.8284952042209,-14.3341115102115));
#56556=CARTESIAN_POINT('Ctrl Pts',(-86.55,57.8284952042209,-14.3341115102115));
#56557=CARTESIAN_POINT('Ctrl Pts',(-85.5900000000001,59.4786368856762,-15.7895125368886));
#56558=CARTESIAN_POINT('Ctrl Pts',(-86.55,59.4786368856762,-15.7895125368886));
#56559=CARTESIAN_POINT('Ctrl Pts',(-85.5900000000001,61.7337643465056,-18.5373932985594));
#56560=CARTESIAN_POINT('Ctrl Pts',(-86.55,61.7337643465056,-18.5373932985594));
#56561=CARTESIAN_POINT('Ctrl Pts',(-85.59,63.6403794020083,-22.1044191793415));
#56562=CARTESIAN_POINT('Ctrl Pts',(-86.5499999999999,63.6403794020083,-22.1044191793415));
#56563=CARTESIAN_POINT('Ctrl Pts',(-85.59,64.5418111191123,-25.076041306158));
#56564=CARTESIAN_POINT('Ctrl Pts',(-86.5499999999999,64.5418111191123,-25.076041306158));
#56565=CARTESIAN_POINT('Ctrl Pts',(-85.59,64.8317241957022,-26.801305653953));
#56566=CARTESIAN_POINT('Ctrl Pts',(-86.5499999999999,64.8317241957022,-26.801305653953));
#56567=CARTESIAN_POINT('Ctrl Pts',(-85.59,64.8871997650571,-27.2044726133659));
#56568=CARTESIAN_POINT('Ctrl Pts',(-86.5499999999999,64.8871997650571,-27.2044726133659));
#56569=CARTESIAN_POINT('',(-85.5900000000001,64.8871997650542,-27.204472613345));
#56570=CARTESIAN_POINT('Ctrl Pts',(-85.5899999999996,44.5787611019615,-12.5));
#56571=CARTESIAN_POINT('Ctrl Pts',(-86.5500000000004,44.5787611019615,-12.5));
#56572=CARTESIAN_POINT('Ctrl Pts',(-85.5899999999996,43.433398281725,-12.5));
#56573=CARTESIAN_POINT('Ctrl Pts',(-86.5500000000004,43.433398281725,-12.5));
#56574=CARTESIAN_POINT('Ctrl Pts',(-85.5899999999999,41.4793849491346,-12.6924535153054));
#56575=CARTESIAN_POINT('Ctrl Pts',(-86.5500000000007,41.4793849491346,-12.6924535153054));
#56576=CARTESIAN_POINT('Ctrl Pts',(-85.5899999999998,39.5894255810997,-13.2069280562477));
#56577=CARTESIAN_POINT('Ctrl Pts',(-86.5500000000005,39.5894255810997,-13.2069280562477));
#56578=CARTESIAN_POINT('Ctrl Pts',(-85.5899999999997,38.8257008878975,-13.4727301359734));
#56579=CARTESIAN_POINT('Ctrl Pts',(-86.5500000000005,38.8257008878975,-13.4727301359734));
#56580=CARTESIAN_POINT('Ctrl Pts',(-85.5900000000001,44.5787611019615,-9.5));
#56581=CARTESIAN_POINT('Ctrl Pts',(-86.5500000000001,44.5787611019615,-9.5));
#56582=CARTESIAN_POINT('Ctrl Pts',(-85.5900000000001,45.9204718342386,-9.5));
#56583=CARTESIAN_POINT('Ctrl Pts',(-86.5500000000001,45.9204718342386,-9.5));
#56584=CARTESIAN_POINT('Ctrl Pts',(-85.59,48.5636521071579,-9.76033053440579));
#56585=CARTESIAN_POINT('Ctrl Pts',(-86.55,48.5636521071579,-9.76033053440579));
#56586=CARTESIAN_POINT('Ctrl Pts',(-85.5900000000001,51.1067797000701,-10.5236598583039));
#56587=CARTESIAN_POINT('Ctrl Pts',(-86.5500000000002,51.1067797000701,-10.5236598583039));
#56588=CARTESIAN_POINT('Ctrl Pts',(-85.5900000000002,52.3121016228057,-11.0146003457735));
#56589=CARTESIAN_POINT('Ctrl Pts',(-86.5500000000002,52.3121016228057,-11.0146003457735));
#56590=CARTESIAN_POINT('',(-85.5900000000002,52.3121016227476,-11.0146003457498));
#56591=CARTESIAN_POINT('Ctrl Pts',(-85.5900000000001,33.1423767334232,-16.7539809977095));
#56592=CARTESIAN_POINT('Ctrl Pts',(-86.5500000000006,33.1423767334232,-16.7539809977095));
#56593=CARTESIAN_POINT('Ctrl Pts',(-85.5900000000001,32.819223330559,-17.0329646666082));
#56594=CARTESIAN_POINT('Ctrl Pts',(-86.5500000000006,32.819223330559,-17.0329646666082));
#56595=CARTESIAN_POINT('Ctrl Pts',(-85.5900000000001,31.6666409722284,-18.1039187234887));
#56596=CARTESIAN_POINT('Ctrl Pts',(-86.5500000000006,31.6666409722284,-18.1039187234887));
#56597=CARTESIAN_POINT('Ctrl Pts',(-85.59,29.9342461371069,-20.2148479377946));
#56598=CARTESIAN_POINT('Ctrl Pts',(-86.5500000000005,29.9342461371069,-20.2148479377946));
#56599=CARTESIAN_POINT('Ctrl Pts',(-85.5900000000004,28.3066479189948,-23.2598700311452));
#56600=CARTESIAN_POINT('Ctrl Pts',(-86.5500000000009,28.3066479189948,-23.2598700311452));
#56601=CARTESIAN_POINT('Ctrl Pts',(-85.5900000000002,27.6253062746369,-25.5059524219446));
#56602=CARTESIAN_POINT('Ctrl Pts',(-86.5500000000007,27.6253062746369,-25.5059524219446));
#56603=CARTESIAN_POINT('Ctrl Pts',(-85.5900000000002,27.3975846520116,-26.674463640704));
#56604=CARTESIAN_POINT('Ctrl Pts',(-86.5500000000007,27.3975846520116,-26.674463640704));
#56605=CARTESIAN_POINT('Ctrl Pts',(-85.5900000000002,27.3891253349641,-26.7187856673309));
#56606=CARTESIAN_POINT('Ctrl Pts',(-86.5500000000007,27.3891253349641,-26.7187856673309));
#56607=CARTESIAN_POINT('',(-86.3900000000002,33.1423767334334,-16.7539809977007));
#56608=CARTESIAN_POINT('Ctrl Pts',(-85.59,24.270322438866,-27.2044726133659));
#56609=CARTESIAN_POINT('Ctrl Pts',(-86.55,24.270322438866,-27.2044726133659));
#56610=CARTESIAN_POINT('Ctrl Pts',(-85.59,24.3257980082209,-26.801305653953));
#56611=CARTESIAN_POINT('Ctrl Pts',(-86.55,24.3257980082209,-26.801305653953));
#56612=CARTESIAN_POINT('Ctrl Pts',(-85.59,24.6157110848108,-25.076041306158));
#56613=CARTESIAN_POINT('Ctrl Pts',(-86.55,24.6157110848108,-25.076041306158));
#56614=CARTESIAN_POINT('Ctrl Pts',(-85.5900000000001,25.5171428019148,-22.1044191793415));
#56615=CARTESIAN_POINT('Ctrl Pts',(-86.5500000000001,25.5171428019148,-22.1044191793415));
#56616=CARTESIAN_POINT('Ctrl Pts',(-85.59,27.4237578574175,-18.5373932985594));
#56617=CARTESIAN_POINT('Ctrl Pts',(-86.55,27.4237578574175,-18.5373932985594));
#56618=CARTESIAN_POINT('Ctrl Pts',(-85.59,29.6788853182468,-15.7895125368886));
#56619=CARTESIAN_POINT('Ctrl Pts',(-86.55,29.6788853182468,-15.7895125368886));
#56620=CARTESIAN_POINT('Ctrl Pts',(-85.59,31.3290269997022,-14.3341115102115));
#56621=CARTESIAN_POINT('Ctrl Pts',(-86.55,31.3290269997022,-14.3341115102115));
#56622=CARTESIAN_POINT('Ctrl Pts',(-85.59,32.0036528607881,-13.8100697594033));
#56623=CARTESIAN_POINT('Ctrl Pts',(-86.55,32.0036528607881,-13.8100697594033));
#56624=CARTESIAN_POINT('',(-86.3899999999999,24.2703224388689,-27.2044726133451));
#56625=CARTESIAN_POINT('',(-85.59,32.0036528607784,-13.8100697594109));
#56626=CARTESIAN_POINT('Ctrl Pts',(-85.5900000000002,27.3891253349641,-33.281214332669));
#56627=CARTESIAN_POINT('Ctrl Pts',(-86.5500000000002,27.3891253349641,-33.281214332669));
#56628=CARTESIAN_POINT('Ctrl Pts',(-85.5900000000002,27.3975846520116,-33.3255363592959));
#56629=CARTESIAN_POINT('Ctrl Pts',(-86.5500000000002,27.3975846520116,-33.3255363592959));
#56630=CARTESIAN_POINT('Ctrl Pts',(-85.5900000000001,27.6253062746369,-34.4940475780554));
#56631=CARTESIAN_POINT('Ctrl Pts',(-86.5500000000002,27.6253062746369,-34.4940475780554));
#56632=CARTESIAN_POINT('Ctrl Pts',(-85.5900000000001,28.3066479189948,-36.7401299688549));
#56633=CARTESIAN_POINT('Ctrl Pts',(-86.5500000000001,28.3066479189948,-36.7401299688549));
#56634=CARTESIAN_POINT('Ctrl Pts',(-85.5900000000001,29.9342461371069,-39.7851520622054));
#56635=CARTESIAN_POINT('Ctrl Pts',(-86.5500000000001,29.9342461371069,-39.7851520622054));
#56636=CARTESIAN_POINT('Ctrl Pts',(-85.5900000000001,31.6666409722284,-41.8960812765113));
#56637=CARTESIAN_POINT('Ctrl Pts',(-86.5500000000002,31.6666409722284,-41.8960812765113));
#56638=CARTESIAN_POINT('Ctrl Pts',(-85.5900000000001,32.8192233305589,-42.9670353333918));
#56639=CARTESIAN_POINT('Ctrl Pts',(-86.5500000000002,32.8192233305589,-42.9670353333918));
#56640=CARTESIAN_POINT('Ctrl Pts',(-85.5900000000001,33.1423767334232,-43.2460190022905));
#56641=CARTESIAN_POINT('Ctrl Pts',(-86.5500000000002,33.1423767334232,-43.2460190022905));
#56642=CARTESIAN_POINT('',(-85.5900000000001,33.1423767334334,-43.2460190022993));
#56643=CARTESIAN_POINT('Ctrl Pts',(-85.5900000000001,32.0036528607881,-46.1899302405967));
#56644=CARTESIAN_POINT('Ctrl Pts',(-86.55,32.0036528607881,-46.1899302405967));
#56645=CARTESIAN_POINT('Ctrl Pts',(-85.59,31.3290269997021,-45.6658884897885));
#56646=CARTESIAN_POINT('Ctrl Pts',(-86.5499999999999,31.3290269997021,-45.6658884897885));
#56647=CARTESIAN_POINT('Ctrl Pts',(-85.5899999999999,29.6788853182468,-44.2104874631114));
#56648=CARTESIAN_POINT('Ctrl Pts',(-86.5499999999997,29.6788853182468,-44.2104874631114));
#56649=CARTESIAN_POINT('Ctrl Pts',(-85.5900000000001,27.4237578574175,-41.4626067014406));
#56650=CARTESIAN_POINT('Ctrl Pts',(-86.5499999999999,27.4237578574175,-41.4626067014406));
#56651=CARTESIAN_POINT('Ctrl Pts',(-85.5899999999997,25.5171428019148,-37.8955808206585));
#56652=CARTESIAN_POINT('Ctrl Pts',(-86.5499999999996,25.5171428019148,-37.8955808206585));
#56653=CARTESIAN_POINT('Ctrl Pts',(-85.5900000000001,24.6157110848108,-34.923958693842));
#56654=CARTESIAN_POINT('Ctrl Pts',(-86.55,24.6157110848108,-34.923958693842));
#56655=CARTESIAN_POINT('Ctrl Pts',(-85.5900000000001,24.3257980082209,-33.198694346047));
#56656=CARTESIAN_POINT('Ctrl Pts',(-86.55,24.3257980082209,-33.198694346047));
#56657=CARTESIAN_POINT('Ctrl Pts',(-85.5900000000001,24.270322438866,-32.7955273866341));
#56658=CARTESIAN_POINT('Ctrl Pts',(-86.5499999999999,24.270322438866,-32.7955273866341));
#56659=CARTESIAN_POINT('',(-86.39,32.0036528607783,-46.189930240589));
#56660=CARTESIAN_POINT('',(-85.5900000000001,24.2703224388689,-32.7955273866549));
#56661=CARTESIAN_POINT('Ctrl Pts',(-85.59,52.3121016227473,-48.9853996542503));
#56662=CARTESIAN_POINT('Ctrl Pts',(-86.5500000000001,52.3121016227473,-48.9853996542503));
#56663=CARTESIAN_POINT('Ctrl Pts',(-85.5900000000001,51.1067797000296,-49.4763401417082));
#56664=CARTESIAN_POINT('Ctrl Pts',(-86.5500000000001,51.1067797000296,-49.4763401417082));
#56665=CARTESIAN_POINT('Ctrl Pts',(-85.5900000000001,48.5636521071369,-50.2396694655963));
#56666=CARTESIAN_POINT('Ctrl Pts',(-86.5500000000002,48.5636521071369,-50.2396694655963));
#56667=CARTESIAN_POINT('Ctrl Pts',(-85.59,44.5787611019615,-50.6321469729213));
#56668=CARTESIAN_POINT('Ctrl Pts',(-86.55,44.5787611019615,-50.6321469729213));
#56669=CARTESIAN_POINT('Ctrl Pts',(-85.5900000000002,40.5938700967862,-50.2396694655963));
#56670=CARTESIAN_POINT('Ctrl Pts',(-86.5500000000002,40.5938700967862,-50.2396694655963));
#56671=CARTESIAN_POINT('Ctrl Pts',(-85.59,38.0507425038934,-49.4763401417082));
#56672=CARTESIAN_POINT('Ctrl Pts',(-86.5500000000001,38.0507425038934,-49.4763401417082));
#56673=CARTESIAN_POINT('Ctrl Pts',(-85.59,36.8454205811756,-48.9853996542502));
#56674=CARTESIAN_POINT('Ctrl Pts',(-86.5500000000001,36.8454205811756,-48.9853996542502));
#56675=CARTESIAN_POINT('',(-86.39,52.3121016227475,-48.9853996542502));
#56676=CARTESIAN_POINT('',(-85.5900000000001,36.8454205811755,-48.9853996542502));
#56677=CARTESIAN_POINT('Ctrl Pts',(-85.5900000000001,38.825700926836,-46.5272698775785));
#56678=CARTESIAN_POINT('Ctrl Pts',(-86.5500000000004,38.825700926836,-46.5272698775785));
#56679=CARTESIAN_POINT('Ctrl Pts',(-85.5900000000001,39.5894256076847,-46.7930719509892));
#56680=CARTESIAN_POINT('Ctrl Pts',(-86.5500000000005,39.5894256076847,-46.7930719509892));
#56681=CARTESIAN_POINT('Ctrl Pts',(-85.5900000000002,41.4793849628776,-47.3075464860481));
#56682=CARTESIAN_POINT('Ctrl Pts',(-86.5500000000006,41.4793849628776,-47.3075464860481));
#56683=CARTESIAN_POINT('Ctrl Pts',(-85.5900000000001,44.5787611019615,-47.6128083915182));
#56684=CARTESIAN_POINT('Ctrl Pts',(-86.5500000000004,44.5787611019615,-47.6128083915182));
#56685=CARTESIAN_POINT('Ctrl Pts',(-85.5900000000004,47.6781372410454,-47.3075464860481));
#56686=CARTESIAN_POINT('Ctrl Pts',(-86.5500000000007,47.6781372410454,-47.3075464860481));
#56687=CARTESIAN_POINT('Ctrl Pts',(-85.5900000000002,49.5680965962383,-46.7930719509892));
#56688=CARTESIAN_POINT('Ctrl Pts',(-86.5500000000005,49.5680965962383,-46.7930719509892));
#56689=CARTESIAN_POINT('Ctrl Pts',(-85.5900000000001,50.331821277087,-46.5272698775786));
#56690=CARTESIAN_POINT('Ctrl Pts',(-86.5500000000004,50.331821277087,-46.5272698775786));
#56691=CARTESIAN_POINT('',(-85.59,50.3318212771098,-46.5272698775706));
#56692=CARTESIAN_POINT('Ctrl Pts',(-85.5900000000003,52.1693515320407,-32.5263626850653));
#56693=CARTESIAN_POINT('Ctrl Pts',(-86.5499999999999,52.1693515320407,-32.5263626850653));
#56694=CARTESIAN_POINT('Ctrl Pts',(-85.5900000000003,52.1092282262322,-32.7070306040739));
#56695=CARTESIAN_POINT('Ctrl Pts',(-86.5499999999999,52.1092282262322,-32.7070306040739));
#56696=CARTESIAN_POINT('Ctrl Pts',(-85.5900000000003,51.8596181813079,-33.3764687724939));
#56697=CARTESIAN_POINT('Ctrl Pts',(-86.5499999999999,51.8596181813079,-33.3764687724939));
#56698=CARTESIAN_POINT('Ctrl Pts',(-85.5900000000005,51.3485297861136,-34.3326479066949));
#56699=CARTESIAN_POINT('Ctrl Pts',(-86.55,51.3485297861136,-34.3326479066949));
#56700=CARTESIAN_POINT('Ctrl Pts',(-85.5900000000003,50.8041422375712,-35.0375762026026));
#56701=CARTESIAN_POINT('Ctrl Pts',(-86.5499999999999,50.8041422375712,-35.0375762026026));
#56702=CARTESIAN_POINT('Ctrl Pts',(-85.5900000000003,50.5618748736091,-35.3105548553452));
#56703=CARTESIAN_POINT('Ctrl Pts',(-86.5499999999999,50.5618748736091,-35.3105548553452));
#56704=CARTESIAN_POINT('',(-86.3899999999999,52.1693515320421,-32.5263626850612));
#56705=CARTESIAN_POINT('Ctrl Pts',(-85.5900000000001,50.5618748736091,-24.6894451446548));
#56706=CARTESIAN_POINT('Ctrl Pts',(-86.5499999999996,50.5618748736091,-24.6894451446548));
#56707=CARTESIAN_POINT('Ctrl Pts',(-85.5900000000001,50.8041422375712,-24.9624237973974));
#56708=CARTESIAN_POINT('Ctrl Pts',(-86.5499999999996,50.8041422375712,-24.9624237973974));
#56709=CARTESIAN_POINT('Ctrl Pts',(-85.59,51.3485297861136,-25.6673520933051));
#56710=CARTESIAN_POINT('Ctrl Pts',(-86.5499999999995,51.3485297861136,-25.6673520933051));
#56711=CARTESIAN_POINT('Ctrl Pts',(-85.59,51.8596181813079,-26.6235312275061));
#56712=CARTESIAN_POINT('Ctrl Pts',(-86.5499999999994,51.8596181813079,-26.6235312275061));
#56713=CARTESIAN_POINT('Ctrl Pts',(-85.59,52.1092282262323,-27.2929693959262));
#56714=CARTESIAN_POINT('Ctrl Pts',(-86.5499999999995,52.1092282262323,-27.2929693959262));
#56715=CARTESIAN_POINT('Ctrl Pts',(-85.59,52.1693515320408,-27.4736373149347));
#56716=CARTESIAN_POINT('Ctrl Pts',(-86.5499999999995,52.1693515320408,-27.4736373149347));
#56717=CARTESIAN_POINT('',(-85.5900000000002,52.1693515320421,-27.4736373149388));
#56718=CARTESIAN_POINT('Ctrl Pts',(-85.5900000000004,44.5787611019615,-22.));
#56719=CARTESIAN_POINT('Ctrl Pts',(-86.55,44.5787611019615,-22.));
#56720=CARTESIAN_POINT('Ctrl Pts',(-85.5900000000005,45.1023555340697,-22.));
#56721=CARTESIAN_POINT('Ctrl Pts',(-86.55,45.1023555340697,-22.));
#56722=CARTESIAN_POINT('Ctrl Pts',(-85.5900000000004,45.6418375870485,-22.0531343444839));
#56723=CARTESIAN_POINT('Ctrl Pts',(-86.55,45.6418375870485,-22.0531343444839));
#56724=CARTESIAN_POINT('Ctrl Pts',(-85.5900000000003,46.1706391043629,-22.1599633677105));
#56725=CARTESIAN_POINT('Ctrl Pts',(-86.5499999999998,46.1706391043629,-22.1599633677105));
#56726=CARTESIAN_POINT('Ctrl Pts',(-85.5900000000003,46.1862026525634,-22.1631559443817));
#56727=CARTESIAN_POINT('Ctrl Pts',(-86.5499999999998,46.1862026525634,-22.1631559443817));
#56728=CARTESIAN_POINT('',(-85.5900000000003,46.1862026525626,-22.1631559443816));
#56729=CARTESIAN_POINT('Ctrl Pts',(-85.5900000000003,36.9881706718823,-27.4736373149347));
#56730=CARTESIAN_POINT('Ctrl Pts',(-86.5499999999998,36.9881706718823,-27.4736373149347));
#56731=CARTESIAN_POINT('Ctrl Pts',(-85.5900000000003,37.0482939776908,-27.2929693959261));
#56732=CARTESIAN_POINT('Ctrl Pts',(-86.5499999999999,37.0482939776908,-27.2929693959261));
#56733=CARTESIAN_POINT('Ctrl Pts',(-85.5900000000004,37.2979040226152,-26.6235312275061));
#56734=CARTESIAN_POINT('Ctrl Pts',(-86.5499999999999,37.2979040226152,-26.6235312275061));
#56735=CARTESIAN_POINT('Ctrl Pts',(-85.5900000000002,37.8089924178094,-25.6673520933051));
#56736=CARTESIAN_POINT('Ctrl Pts',(-86.5499999999997,37.8089924178094,-25.6673520933051));
#56737=CARTESIAN_POINT('Ctrl Pts',(-85.5900000000003,38.3533799663518,-24.9624237973974));
#56738=CARTESIAN_POINT('Ctrl Pts',(-86.5499999999998,38.3533799663518,-24.9624237973974));
#56739=CARTESIAN_POINT('Ctrl Pts',(-85.5900000000003,38.5956473303139,-24.6894451446548));
#56740=CARTESIAN_POINT('Ctrl Pts',(-86.5499999999998,38.5956473303139,-24.6894451446548));
#56741=CARTESIAN_POINT('',(-86.3899999999997,36.988170671881,-27.4736373149387));
#56742=CARTESIAN_POINT('',(-85.5900000000003,38.5956473303199,-24.6894451446481));
#56743=CARTESIAN_POINT('Ctrl Pts',(-85.5900000000007,38.5956473303139,-35.3105548553452));
#56744=CARTESIAN_POINT('Ctrl Pts',(-86.5499999999998,38.5956473303139,-35.3105548553452));
#56745=CARTESIAN_POINT('Ctrl Pts',(-85.5900000000006,38.3533799663518,-35.0375762026026));
#56746=CARTESIAN_POINT('Ctrl Pts',(-86.5499999999997,38.3533799663518,-35.0375762026026));
#56747=CARTESIAN_POINT('Ctrl Pts',(-85.5900000000005,37.8089924178094,-34.3326479066949));
#56748=CARTESIAN_POINT('Ctrl Pts',(-86.5499999999996,37.8089924178094,-34.3326479066949));
#56749=CARTESIAN_POINT('Ctrl Pts',(-85.5900000000008,37.2979040226152,-33.3764687724939));
#56750=CARTESIAN_POINT('Ctrl Pts',(-86.5499999999999,37.2979040226152,-33.3764687724939));
#56751=CARTESIAN_POINT('Ctrl Pts',(-85.5900000000007,37.0482939776908,-32.7070306040739));
#56752=CARTESIAN_POINT('Ctrl Pts',(-86.5499999999999,37.0482939776908,-32.7070306040739));
#56753=CARTESIAN_POINT('Ctrl Pts',(-85.5900000000007,36.9881706718823,-32.5263626850653));
#56754=CARTESIAN_POINT('Ctrl Pts',(-86.5499999999998,36.9881706718823,-32.5263626850653));
#56755=CARTESIAN_POINT('',(-86.3899999999999,38.5956473303199,-35.3105548553519));
#56756=CARTESIAN_POINT('',(-85.5900000000003,36.988170671881,-32.5263626850613));
#56757=CARTESIAN_POINT('Ctrl Pts',(-85.5900000000002,46.1862026525626,-37.8368440556185));
#56758=CARTESIAN_POINT('Ctrl Pts',(-86.5499999999997,46.1862026525626,-37.8368440556185));
#56759=CARTESIAN_POINT('Ctrl Pts',(-85.5900000000002,46.1706391043624,-37.8400366322896));
#56760=CARTESIAN_POINT('Ctrl Pts',(-86.5499999999997,46.1706391043624,-37.8400366322896));
#56761=CARTESIAN_POINT('Ctrl Pts',(-85.5900000000001,45.6418375870482,-37.9468656555161));
#56762=CARTESIAN_POINT('Ctrl Pts',(-86.5499999999996,45.6418375870482,-37.9468656555161));
#56763=CARTESIAN_POINT('Ctrl Pts',(-85.5900000000003,44.5787611019615,-38.0515695504083));
#56764=CARTESIAN_POINT('Ctrl Pts',(-86.5499999999997,44.5787611019615,-38.0515695504083));
#56765=CARTESIAN_POINT('Ctrl Pts',(-85.5900000000001,43.5156846168748,-37.9468656555161));
#56766=CARTESIAN_POINT('Ctrl Pts',(-86.5499999999996,43.5156846168748,-37.9468656555161));
#56767=CARTESIAN_POINT('Ctrl Pts',(-85.5900000000002,42.9868830995607,-37.8400366322896));
#56768=CARTESIAN_POINT('Ctrl Pts',(-86.5499999999997,42.9868830995607,-37.8400366322896));
#56769=CARTESIAN_POINT('Ctrl Pts',(-85.5900000000002,42.9713195513605,-37.8368440556185));
#56770=CARTESIAN_POINT('Ctrl Pts',(-86.5499999999997,42.9713195513605,-37.8368440556185));
#56771=CARTESIAN_POINT('',(-86.3899999999996,46.1862026525626,-37.8368440556185));
#56772=CARTESIAN_POINT('',(-85.5900000000001,42.9713195513605,-37.8368440556185));
#56773=CARTESIAN_POINT('Origin',(-85.9899999999996,53.5926110635042,-32.9999999999999));
#56774=CARTESIAN_POINT('Origin',(-85.9899999999997,66.3731980659926,-33.));
#56775=CARTESIAN_POINT('Origin',(-85.9899999999997,60.2949931567668,-33.));
#56776=CARTESIAN_POINT('Origin',(-85.99,78.4460245797131,-33.));
#56777=CARTESIAN_POINT('Origin',(-85.99,72.4174689786827,-33.));
#56778=CARTESIAN_POINT('Origin',(-85.9900000000002,66.3683162666315,-61.7406166195334));
#56779=CARTESIAN_POINT('Origin',(-85.9899999998252,61.1722799429393,-64.740817708925));
#56780=CARTESIAN_POINT('Origin',(-85.9899999999997,22.7892059208967,-61.7406166479301));
#56781=CARTESIAN_POINT('Origin',(-85.9900000000002,22.789205939653,1.74061661544304));
#56782=CARTESIAN_POINT('Origin',(-85.99,61.1722800421212,4.74081788071294));
#56783=CARTESIAN_POINT('Origin',(-85.990000000157,66.3683162853859,1.74061665201678));
#56784=CARTESIAN_POINT('Origin',(-85.9900000000001,82.9621121574678,-27.));
#56785=CARTESIAN_POINT('Origin',(-85.9900000000747,82.9621122252415,-33.));
#56786=CARTESIAN_POINT('Origin',(-85.9899999999998,30.2431724514241,0.829967899138609));
#56787=CARTESIAN_POINT('Origin',(-85.9899999999996,58.9143497524989,-60.8299678991386));
#56788=CARTESIAN_POINT('Origin',(-85.9899999999992,30.2431724514241,-60.8299678991386));
#56789=CARTESIAN_POINT('Origin',(-85.9899999999993,25.0470014756374,-57.8300000340158));
#56790=CARTESIAN_POINT('Origin',(-85.9899999999993,10.7114976242099,-33.));
#56791=CARTESIAN_POINT('Origin',(-85.9899999999996,10.7114976242099,-27.));
#56792=CARTESIAN_POINT('Origin',(-85.9899999999995,25.0470014756374,-2.16999996598413));
#56793=CARTESIAN_POINT('Origin',(-85.9899999999996,58.914349752499,0.829967899138591));
#56794=CARTESIAN_POINT('Origin',(-85.9899999999997,78.4460245797131,-27.));
#56795=CARTESIAN_POINT('Origin',(-85.9899999999993,61.0962221090322,-52.6090816762843));
#56796=CARTESIAN_POINT('Origin',(-85.9899999999997,55.9000854795073,-55.6091090308774));
#56797=CARTESIAN_POINT('Origin',(-85.9899999999995,28.0613000948908,-52.6090816762843));
#56798=CARTESIAN_POINT('Origin',(-85.9899999999995,28.0613000948908,-7.39091832371568));
#56799=CARTESIAN_POINT('Origin',(-85.9899999999996,55.9000854795073,-4.39089096912261));
#56800=CARTESIAN_POINT('Origin',(-85.9899999999996,61.0962221090323,-7.39091832371568));
#56801=CARTESIAN_POINT('Origin',(-85.9899999999997,72.4174689786827,-27.));
#56802=CARTESIAN_POINT('Origin',(-85.9899999999997,36.2795905006212,-9.62541485779656));
#56803=CARTESIAN_POINT('Origin',(-85.9899999999996,52.8779317033019,-50.3745851422034));
#56804=CARTESIAN_POINT('Origin',(-85.9899999999998,36.2795905006212,-50.3745851422034));
#56805=CARTESIAN_POINT('Origin',(-85.9899999999997,31.0834721426076,-47.3745261404244));
#56806=CARTESIAN_POINT('Origin',(-85.9899999999996,22.7843241379305,-33.));
#56807=CARTESIAN_POINT('Origin',(-85.9899999999995,22.7843241379304,-27.));
#56808=CARTESIAN_POINT('Origin',(-85.9899999999996,31.0834721426076,-12.6254738595756));
#56809=CARTESIAN_POINT('Origin',(-85.99,52.8779317033019,-9.62541485779658));
#56810=CARTESIAN_POINT('Origin',(-85.9899999999997,66.3731980659926,-27.));
#56811=CARTESIAN_POINT('Origin',(-85.9899999999998,55.0349236943356,-42.110604862193));
#56812=CARTESIAN_POINT('Origin',(-85.9899999999998,49.8387777318655,-45.1106160516509));
#56813=CARTESIAN_POINT('Origin',(-85.9899999999997,34.1225985095874,-42.110604862193));
#56814=CARTESIAN_POINT('Origin',(-85.9899999999997,34.1225985095875,-17.889395137807));
#56815=CARTESIAN_POINT('Origin',(-85.9899999999999,49.8387777318655,-14.8893839483491));
#56816=CARTESIAN_POINT('Origin',(-85.9899999999999,55.0349236943356,-17.889395137807));
#56817=CARTESIAN_POINT('Origin',(-85.9899999999997,60.2949931567668,-27.));
#56818=CARTESIAN_POINT('Origin',(-85.9899999999995,42.6698984466481,-20.6937528963263));
#56819=CARTESIAN_POINT('Origin',(-85.9899999999997,46.4876237572749,-39.3062471036737));
#56820=CARTESIAN_POINT('Origin',(-85.9899999999996,42.6698984466481,-39.3062471036737));
#56821=CARTESIAN_POINT('Origin',(-85.9899999999993,37.4737575460498,-36.3062271467965));
#56822=CARTESIAN_POINT('Origin',(-85.9899999999993,35.5649111404189,-33.));
#56823=CARTESIAN_POINT('Origin',(-85.9899999999993,35.5649111404189,-27.));
#56824=CARTESIAN_POINT('Origin',(-85.9899999999995,37.4737575460499,-23.6937728532035));
#56825=CARTESIAN_POINT('Origin',(-85.989999999999,46.487623757275,-20.6937528963263));
#56826=CARTESIAN_POINT('Origin',(-85.9899999999992,53.5926110635042,-27.));
#56827=CARTESIAN_POINT('Origin',(-74.39,76.,45.));
#56828=CARTESIAN_POINT('',(-74.39,76.,47.667));
#56829=CARTESIAN_POINT('',(-74.39,78.667,45.));
#56830=CARTESIAN_POINT('Origin',(-74.39,70.792807570849,47.667));
#56831=CARTESIAN_POINT('',(-74.39,70.792807570849,47.667));
#56832=CARTESIAN_POINT('Origin',(-74.39,70.792807570849,45.));
#56833=CARTESIAN_POINT('',(-74.39,68.9069537854245,46.8858537854245));
#56834=CARTESIAN_POINT('Origin',(-74.39,66.0242462145755,44.0031462145755));
#56835=CARTESIAN_POINT('',(-74.39,66.0242462145755,44.0031462145755));
#56836=CARTESIAN_POINT('Origin',(-74.39,67.9101,42.117292429151));
#56837=CARTESIAN_POINT('',(-74.39,65.2431,42.117292429151));
#56838=CARTESIAN_POINT('Origin',(-74.39,65.2431,34.547707570849));
#56839=CARTESIAN_POINT('',(-74.39,65.2431,34.547707570849));
#56840=CARTESIAN_POINT('Origin',(-74.39,67.9101,34.547707570849));
#56841=CARTESIAN_POINT('',(-74.39,66.0242462145755,32.6618537854245));
#56842=CARTESIAN_POINT('Origin',(-74.39,68.9069537854245,29.7791462145755));
#56843=CARTESIAN_POINT('',(-74.39,68.9069537854245,29.7791462145755));
#56844=CARTESIAN_POINT('Origin',(-74.39,70.792807570849,31.665));
#56845=CARTESIAN_POINT('',(-74.39,70.792807570849,28.998));
#56846=CARTESIAN_POINT('Origin',(-74.39,76.,28.998));
#56847=CARTESIAN_POINT('',(-74.39,76.,28.998));
#56848=CARTESIAN_POINT('Origin',(-74.39,76.,31.665));
#56849=CARTESIAN_POINT('',(-74.39,78.667,31.665));
#56850=CARTESIAN_POINT('Origin',(-74.39,78.667,45.));
#56851=CARTESIAN_POINT('Origin',(-74.39,64.417,65.));
#56852=CARTESIAN_POINT('',(-74.39,64.417,65.));
#56853=CARTESIAN_POINT('',(-74.39,64.417,75.));
#56854=CARTESIAN_POINT('Origin',(-74.39,64.6169999999999,65.));
#56855=CARTESIAN_POINT('',(-74.39,78.6669999999999,65.));
#56856=CARTESIAN_POINT('Origin',(-74.39,78.667,75.));
#56857=CARTESIAN_POINT('',(-74.39,78.667,75.));
#56858=CARTESIAN_POINT('Origin',(-74.39,78.467,75.));
#56859=CARTESIAN_POINT('Origin',(-84.39,91.,75.));
#56860=CARTESIAN_POINT('Origin',(69.81,91.,75.));
#56861=CARTESIAN_POINT('Origin',(69.01,86.,-80.));
#56862=CARTESIAN_POINT('Origin',(-82.79,86.,-80.));
#56863=CARTESIAN_POINT('Origin',(60.61,1.21259619067905E-14,-69.5));
#56864=CARTESIAN_POINT('',(60.61,46.0787611019615,-69.5));
#56865=CARTESIAN_POINT('Origin',(60.61,46.0787611019615,-68.));
#56866=CARTESIAN_POINT('',(60.61,46.0787611019615,-66.5));
#56867=CARTESIAN_POINT('Origin',(60.61,1.21259619067905E-14,-66.5));
#56868=CARTESIAN_POINT('Origin',(60.61,1.21259619067905E-14,-16.5));
#56869=CARTESIAN_POINT('',(60.61,18.0787611019615,-16.5));
#56870=CARTESIAN_POINT('Origin',(60.61,1.21259619067905E-14,-19.5));
#56871=CARTESIAN_POINT('',(60.61,18.0787611019615,-19.5));
#56872=CARTESIAN_POINT('Origin',(60.61,18.0787611019615,-18.));
#56873=CARTESIAN_POINT('Origin',(60.61,1.21259619067905E-14,-21.5));
#56874=CARTESIAN_POINT('',(60.61,18.0787611019615,-21.5));
#56875=CARTESIAN_POINT('Origin',(60.61,1.21259619067905E-14,-24.5));
#56876=CARTESIAN_POINT('',(60.61,18.0787611019615,-24.5));
#56877=CARTESIAN_POINT('Origin',(60.61,18.0787611019615,-23.));
#56878=CARTESIAN_POINT('Origin',(60.61,1.21259619067905E-14,-24.5));
#56879=CARTESIAN_POINT('',(60.61,46.0787611019615,-24.5));
#56880=CARTESIAN_POINT('Origin',(60.61,46.0787611019615,-23.));
#56881=CARTESIAN_POINT('',(60.61,46.0787611019615,-21.5));
#56882=CARTESIAN_POINT('Origin',(60.61,1.21259619067905E-14,-21.5));
#56883=CARTESIAN_POINT('Origin',(60.61,1.21259619067905E-14,-26.5));
#56884=CARTESIAN_POINT('',(60.61,18.0787611019615,-26.5));
#56885=CARTESIAN_POINT('Origin',(60.61,1.21259619067905E-14,-29.5));
#56886=CARTESIAN_POINT('',(60.61,18.0787611019615,-29.5));
#56887=CARTESIAN_POINT('Origin',(60.61,18.0787611019615,-28.));
#56888=CARTESIAN_POINT('Origin',(60.61,1.21259619067905E-14,-19.5));
#56889=CARTESIAN_POINT('',(60.61,46.0787611019615,-19.5));
#56890=CARTESIAN_POINT('Origin',(60.61,46.0787611019615,-18.));
#56891=CARTESIAN_POINT('',(60.61,46.0787611019615,-16.5));
#56892=CARTESIAN_POINT('Origin',(60.61,1.21259619067905E-14,-16.5));
#56893=CARTESIAN_POINT('Origin',(60.61,1.21259619067905E-14,-14.5));
#56894=CARTESIAN_POINT('',(60.61,46.0787611019615,-14.5));
#56895=CARTESIAN_POINT('Origin',(60.61,46.0787611019615,-13.));
#56896=CARTESIAN_POINT('',(60.61,46.0787611019615,-11.5));
#56897=CARTESIAN_POINT('Origin',(60.61,1.21259619067905E-14,-11.5));
#56898=CARTESIAN_POINT('Origin',(60.61,1.21259619067905E-14,-11.5));
#56899=CARTESIAN_POINT('',(60.61,18.0787611019615,-11.5));
#56900=CARTESIAN_POINT('Origin',(60.61,1.21259619067905E-14,-14.5));
#56901=CARTESIAN_POINT('',(60.61,18.0787611019615,-14.5));
#56902=CARTESIAN_POINT('Origin',(60.61,18.0787611019615,-13.));
#56903=CARTESIAN_POINT('Origin',(60.61,1.21259619067905E-14,-51.5));
#56904=CARTESIAN_POINT('',(60.61,18.0787611019615,-51.5));
#56905=CARTESIAN_POINT('Origin',(60.61,1.21259619067905E-14,-54.5));
#56906=CARTESIAN_POINT('',(60.61,18.0787611019615,-54.5));
#56907=CARTESIAN_POINT('Origin',(60.61,18.0787611019615,-53.));
#56908=CARTESIAN_POINT('Origin',(60.61,1.21259619067905E-14,-46.5));
#56909=CARTESIAN_POINT('',(60.61,18.0787611019615,-46.5));
#56910=CARTESIAN_POINT('Origin',(60.61,1.21259619067905E-14,-49.5));
#56911=CARTESIAN_POINT('',(60.61,18.0787611019615,-49.5));
#56912=CARTESIAN_POINT('Origin',(60.61,18.0787611019615,-48.));
#56913=CARTESIAN_POINT('Origin',(60.61,1.21259619067905E-14,-41.5));
#56914=CARTESIAN_POINT('',(60.61,18.0787611019615,-41.5));
#56915=CARTESIAN_POINT('Origin',(60.61,1.21259619067905E-14,-44.5));
#56916=CARTESIAN_POINT('',(60.61,18.0787611019615,-44.5));
#56917=CARTESIAN_POINT('Origin',(60.61,18.0787611019615,-43.));
#56918=CARTESIAN_POINT('Origin',(60.61,1.21259619067905E-14,-44.5));
#56919=CARTESIAN_POINT('',(60.61,46.0787611019615,-44.5));
#56920=CARTESIAN_POINT('Origin',(60.61,46.0787611019615,-43.));
#56921=CARTESIAN_POINT('',(60.61,46.0787611019615,-41.5));
#56922=CARTESIAN_POINT('Origin',(60.61,1.21259619067905E-14,-41.5));
#56923=CARTESIAN_POINT('Origin',(60.61,1.21259619067905E-14,-49.5));
#56924=CARTESIAN_POINT('',(60.61,46.0787611019615,-49.5));
#56925=CARTESIAN_POINT('Origin',(60.61,46.0787611019615,-48.));
#56926=CARTESIAN_POINT('',(60.61,46.0787611019615,-46.5));
#56927=CARTESIAN_POINT('Origin',(60.61,1.21259619067905E-14,-46.5));
#56928=CARTESIAN_POINT('Origin',(60.61,1.21259619067905E-14,-54.5));
#56929=CARTESIAN_POINT('',(60.61,46.0787611019615,-54.5));
#56930=CARTESIAN_POINT('Origin',(60.61,46.0787611019615,-53.));
#56931=CARTESIAN_POINT('',(60.61,46.0787611019615,-51.5));
#56932=CARTESIAN_POINT('Origin',(60.61,1.21259619067905E-14,-51.5));
#56933=CARTESIAN_POINT('Origin',(60.61,1.21259619067905E-14,-59.5));
#56934=CARTESIAN_POINT('',(60.61,46.0787611019615,-59.5));
#56935=CARTESIAN_POINT('Origin',(60.61,46.0787611019615,-58.));
#56936=CARTESIAN_POINT('',(60.61,46.0787611019615,-56.5));
#56937=CARTESIAN_POINT('Origin',(60.61,1.21259619067905E-14,-56.5));
#56938=CARTESIAN_POINT('Origin',(60.61,1.21259619067905E-14,-64.5));
#56939=CARTESIAN_POINT('',(60.61,46.0787611019615,-64.5));
#56940=CARTESIAN_POINT('Origin',(60.61,46.0787611019615,-63.));
#56941=CARTESIAN_POINT('',(60.61,46.0787611019615,-61.5));
#56942=CARTESIAN_POINT('Origin',(60.61,1.21259619067905E-14,-61.5));
#56943=CARTESIAN_POINT('Origin',(60.61,1.21259619067905E-14,-29.5));
#56944=CARTESIAN_POINT('',(60.61,46.0787611019615,-29.5));
#56945=CARTESIAN_POINT('Origin',(60.61,46.0787611019615,-28.));
#56946=CARTESIAN_POINT('',(60.61,46.0787611019615,-26.5));
#56947=CARTESIAN_POINT('Origin',(60.61,1.21259619067905E-14,-26.5));
#56948=CARTESIAN_POINT('Origin',(60.61,1.21259619067905E-14,-34.5));
#56949=CARTESIAN_POINT('',(60.61,46.0787611019615,-34.5));
#56950=CARTESIAN_POINT('Origin',(60.61,46.0787611019615,-33.));
#56951=CARTESIAN_POINT('',(60.61,46.0787611019615,-31.5));
#56952=CARTESIAN_POINT('Origin',(60.61,1.21259619067905E-14,-31.5));
#56953=CARTESIAN_POINT('Origin',(60.61,1.21259619067905E-14,-31.5));
#56954=CARTESIAN_POINT('',(60.61,18.0787611019615,-31.5));
#56955=CARTESIAN_POINT('Origin',(60.61,1.21259619067905E-14,-34.5));
#56956=CARTESIAN_POINT('',(60.61,18.0787611019615,-34.5));
#56957=CARTESIAN_POINT('Origin',(60.61,18.0787611019615,-33.));
#56958=CARTESIAN_POINT('Origin',(60.61,1.21259619067905E-14,-36.5));
#56959=CARTESIAN_POINT('',(60.61,18.0787611019615,-36.5));
#56960=CARTESIAN_POINT('Origin',(60.61,1.21259619067905E-14,-39.5));
#56961=CARTESIAN_POINT('',(60.61,18.0787611019615,-39.5));
#56962=CARTESIAN_POINT('Origin',(60.61,18.0787611019615,-38.));
#56963=CARTESIAN_POINT('Origin',(60.61,1.21259619067905E-14,-56.5));
#56964=CARTESIAN_POINT('',(60.61,18.0787611019615,-56.5));
#56965=CARTESIAN_POINT('Origin',(60.61,1.21259619067905E-14,-59.5));
#56966=CARTESIAN_POINT('',(60.61,18.0787611019615,-59.5));
#56967=CARTESIAN_POINT('Origin',(60.61,18.0787611019615,-58.));
#56968=CARTESIAN_POINT('Origin',(60.61,1.21259619067905E-14,-61.5));
#56969=CARTESIAN_POINT('',(60.61,18.0787611019615,-61.5));
#56970=CARTESIAN_POINT('Origin',(60.61,1.21259619067905E-14,-64.5));
#56971=CARTESIAN_POINT('',(60.61,18.0787611019615,-64.5));
#56972=CARTESIAN_POINT('Origin',(60.61,18.0787611019615,-63.));
#56973=CARTESIAN_POINT('Origin',(60.61,1.21259619067905E-14,-66.5));
#56974=CARTESIAN_POINT('',(60.61,18.0787611019615,-66.5));
#56975=CARTESIAN_POINT('Origin',(60.61,1.21259619067905E-14,-69.5));
#56976=CARTESIAN_POINT('',(60.61,18.0787611019615,-69.5));
#56977=CARTESIAN_POINT('Origin',(60.61,18.0787611019615,-68.));
#56978=CARTESIAN_POINT('Origin',(60.61,1.21259619067905E-14,-39.5));
#56979=CARTESIAN_POINT('',(60.61,46.0787611019615,-39.5));
#56980=CARTESIAN_POINT('Origin',(60.61,46.0787611019615,-38.));
#56981=CARTESIAN_POINT('',(60.61,46.0787611019615,-36.5));
#56982=CARTESIAN_POINT('Origin',(60.61,1.21259619067905E-14,-36.5));
#56983=CARTESIAN_POINT('Origin',(60.61,1.21259619067905E-14,66.5));
#56984=CARTESIAN_POINT('',(60.61,46.0787611019615,66.5));
#56985=CARTESIAN_POINT('Origin',(60.61,46.0787611019615,68.));
#56986=CARTESIAN_POINT('',(60.61,46.0787611019615,69.5));
#56987=CARTESIAN_POINT('Origin',(60.61,1.21259619067905E-14,69.5));
#56988=CARTESIAN_POINT('Origin',(60.61,1.21259619067905E-14,16.5));
#56989=CARTESIAN_POINT('',(60.61,18.0787611019615,16.5));
#56990=CARTESIAN_POINT('Origin',(60.61,18.0787611019615,18.));
#56991=CARTESIAN_POINT('',(60.61,18.0787611019615,19.5));
#56992=CARTESIAN_POINT('Origin',(60.61,1.21259619067905E-14,19.5));
#56993=CARTESIAN_POINT('Origin',(60.61,1.21259619067905E-14,21.5));
#56994=CARTESIAN_POINT('',(60.61,18.0787611019615,21.5));
#56995=CARTESIAN_POINT('Origin',(60.61,18.0787611019615,23.));
#56996=CARTESIAN_POINT('',(60.61,18.0787611019615,24.5));
#56997=CARTESIAN_POINT('Origin',(60.61,1.21259619067905E-14,24.5));
#56998=CARTESIAN_POINT('Origin',(60.61,1.21259619067905E-14,21.5));
#56999=CARTESIAN_POINT('',(60.61,46.0787611019615,21.5));
#57000=CARTESIAN_POINT('Origin',(60.61,46.0787611019615,23.));
#57001=CARTESIAN_POINT('',(60.61,46.0787611019615,24.5));
#57002=CARTESIAN_POINT('Origin',(60.61,1.21259619067905E-14,24.5));
#57003=CARTESIAN_POINT('Origin',(60.61,1.21259619067905E-14,26.5));
#57004=CARTESIAN_POINT('',(60.61,18.0787611019615,26.5));
#57005=CARTESIAN_POINT('Origin',(60.61,18.0787611019615,28.));
#57006=CARTESIAN_POINT('',(60.61,18.0787611019615,29.5));
#57007=CARTESIAN_POINT('Origin',(60.61,1.21259619067905E-14,29.5));
#57008=CARTESIAN_POINT('Origin',(60.61,1.21259619067905E-14,16.5));
#57009=CARTESIAN_POINT('',(60.61,46.0787611019615,16.5));
#57010=CARTESIAN_POINT('Origin',(60.61,46.0787611019615,18.));
#57011=CARTESIAN_POINT('',(60.61,46.0787611019615,19.5));
#57012=CARTESIAN_POINT('Origin',(60.61,1.21259619067905E-14,19.5));
#57013=CARTESIAN_POINT('Origin',(60.61,1.21259619067905E-14,11.5));
#57014=CARTESIAN_POINT('',(60.61,46.0787611019615,11.5));
#57015=CARTESIAN_POINT('Origin',(60.61,46.0787611019615,13.));
#57016=CARTESIAN_POINT('',(60.61,46.0787611019615,14.5));
#57017=CARTESIAN_POINT('Origin',(60.61,1.21259619067905E-14,14.5));
#57018=CARTESIAN_POINT('Origin',(60.61,1.21259619067905E-14,11.5));
#57019=CARTESIAN_POINT('',(60.61,18.0787611019615,11.5));
#57020=CARTESIAN_POINT('Origin',(60.61,18.0787611019615,13.));
#57021=CARTESIAN_POINT('',(60.61,18.0787611019615,14.5));
#57022=CARTESIAN_POINT('Origin',(60.61,1.21259619067905E-14,14.5));
#57023=CARTESIAN_POINT('Origin',(60.61,1.21259619067905E-14,51.5));
#57024=CARTESIAN_POINT('',(60.61,18.0787611019615,51.5));
#57025=CARTESIAN_POINT('Origin',(60.61,18.0787611019615,53.));
#57026=CARTESIAN_POINT('',(60.61,18.0787611019615,54.5));
#57027=CARTESIAN_POINT('Origin',(60.61,1.21259619067905E-14,54.5));
#57028=CARTESIAN_POINT('Origin',(60.61,1.21259619067905E-14,46.5));
#57029=CARTESIAN_POINT('',(60.61,18.0787611019615,46.5));
#57030=CARTESIAN_POINT('Origin',(60.61,18.0787611019615,48.));
#57031=CARTESIAN_POINT('',(60.61,18.0787611019615,49.5));
#57032=CARTESIAN_POINT('Origin',(60.61,1.21259619067905E-14,49.5));
#57033=CARTESIAN_POINT('Origin',(60.61,1.21259619067905E-14,41.5));
#57034=CARTESIAN_POINT('',(60.61,18.0787611019615,41.5));
#57035=CARTESIAN_POINT('Origin',(60.61,18.0787611019615,43.));
#57036=CARTESIAN_POINT('',(60.61,18.0787611019615,44.5));
#57037=CARTESIAN_POINT('Origin',(60.61,1.21259619067905E-14,44.5));
#57038=CARTESIAN_POINT('Origin',(60.61,1.21259619067905E-14,41.5));
#57039=CARTESIAN_POINT('',(60.61,46.0787611019615,41.5));
#57040=CARTESIAN_POINT('Origin',(60.61,46.0787611019615,43.));
#57041=CARTESIAN_POINT('',(60.61,46.0787611019615,44.5));
#57042=CARTESIAN_POINT('Origin',(60.61,1.21259619067905E-14,44.5));
#57043=CARTESIAN_POINT('Origin',(60.61,1.21259619067905E-14,46.5));
#57044=CARTESIAN_POINT('',(60.61,46.0787611019615,46.5));
#57045=CARTESIAN_POINT('Origin',(60.61,46.0787611019615,48.));
#57046=CARTESIAN_POINT('',(60.61,46.0787611019615,49.5));
#57047=CARTESIAN_POINT('Origin',(60.61,1.21259619067905E-14,49.5));
#57048=CARTESIAN_POINT('Origin',(60.61,1.21259619067905E-14,51.5));
#57049=CARTESIAN_POINT('',(60.61,46.0787611019615,51.5));
#57050=CARTESIAN_POINT('Origin',(60.61,46.0787611019615,53.));
#57051=CARTESIAN_POINT('',(60.61,46.0787611019615,54.5));
#57052=CARTESIAN_POINT('Origin',(60.61,1.21259619067905E-14,54.5));
#57053=CARTESIAN_POINT('Origin',(60.61,1.21259619067905E-14,56.5));
#57054=CARTESIAN_POINT('',(60.61,46.0787611019615,56.5));
#57055=CARTESIAN_POINT('Origin',(60.61,46.0787611019615,58.));
#57056=CARTESIAN_POINT('',(60.61,46.0787611019615,59.5));
#57057=CARTESIAN_POINT('Origin',(60.61,1.21259619067905E-14,59.5));
#57058=CARTESIAN_POINT('Origin',(60.61,1.21259619067905E-14,61.5));
#57059=CARTESIAN_POINT('',(60.61,46.0787611019615,61.5));
#57060=CARTESIAN_POINT('Origin',(60.61,46.0787611019615,63.));
#57061=CARTESIAN_POINT('',(60.61,46.0787611019615,64.5));
#57062=CARTESIAN_POINT('Origin',(60.61,1.21259619067905E-14,64.5));
#57063=CARTESIAN_POINT('Origin',(60.61,1.21259619067905E-14,26.5));
#57064=CARTESIAN_POINT('',(60.61,46.0787611019615,26.5));
#57065=CARTESIAN_POINT('Origin',(60.61,46.0787611019615,28.));
#57066=CARTESIAN_POINT('',(60.61,46.0787611019615,29.5));
#57067=CARTESIAN_POINT('Origin',(60.61,1.21259619067905E-14,29.5));
#57068=CARTESIAN_POINT('Origin',(60.61,1.21259619067905E-14,31.5));
#57069=CARTESIAN_POINT('',(60.61,46.0787611019615,31.5));
#57070=CARTESIAN_POINT('Origin',(60.61,46.0787611019615,33.));
#57071=CARTESIAN_POINT('',(60.61,46.0787611019615,34.5));
#57072=CARTESIAN_POINT('Origin',(60.61,1.21259619067905E-14,34.5));
#57073=CARTESIAN_POINT('Origin',(60.61,1.21259619067905E-14,31.5));
#57074=CARTESIAN_POINT('',(60.61,18.0787611019615,31.5));
#57075=CARTESIAN_POINT('Origin',(60.61,18.0787611019615,33.));
#57076=CARTESIAN_POINT('',(60.61,18.0787611019615,34.5));
#57077=CARTESIAN_POINT('Origin',(60.61,1.21259619067905E-14,34.5));
#57078=CARTESIAN_POINT('Origin',(60.61,1.21259619067905E-14,36.5));
#57079=CARTESIAN_POINT('',(60.61,18.0787611019615,36.5));
#57080=CARTESIAN_POINT('Origin',(60.61,18.0787611019615,38.));
#57081=CARTESIAN_POINT('',(60.61,18.0787611019615,39.5));
#57082=CARTESIAN_POINT('Origin',(60.61,1.21259619067905E-14,39.5));
#57083=CARTESIAN_POINT('Origin',(60.61,1.21259619067905E-14,56.5));
#57084=CARTESIAN_POINT('',(60.61,18.0787611019615,56.5));
#57085=CARTESIAN_POINT('Origin',(60.61,18.0787611019615,58.));
#57086=CARTESIAN_POINT('',(60.61,18.0787611019615,59.5));
#57087=CARTESIAN_POINT('Origin',(60.61,1.21259619067905E-14,59.5));
#57088=CARTESIAN_POINT('Origin',(60.61,1.21259619067905E-14,61.5));
#57089=CARTESIAN_POINT('',(60.61,18.0787611019615,61.5));
#57090=CARTESIAN_POINT('Origin',(60.61,18.0787611019615,63.));
#57091=CARTESIAN_POINT('',(60.61,18.0787611019615,64.5));
#57092=CARTESIAN_POINT('Origin',(60.61,1.21259619067905E-14,64.5));
#57093=CARTESIAN_POINT('Origin',(60.61,1.21259619067905E-14,66.5));
#57094=CARTESIAN_POINT('',(60.61,18.0787611019615,66.5));
#57095=CARTESIAN_POINT('Origin',(60.61,18.0787611019615,68.));
#57096=CARTESIAN_POINT('',(60.61,18.0787611019615,69.5));
#57097=CARTESIAN_POINT('Origin',(60.61,1.21259619067905E-14,69.5));
#57098=CARTESIAN_POINT('Origin',(60.61,1.21259619067905E-14,36.5));
#57099=CARTESIAN_POINT('',(60.61,46.0787611019615,36.5));
#57100=CARTESIAN_POINT('Origin',(60.61,46.0787611019615,38.));
#57101=CARTESIAN_POINT('',(60.61,46.0787611019615,39.5));
#57102=CARTESIAN_POINT('Origin',(60.61,1.21259619067905E-14,39.5));
#57103=CARTESIAN_POINT('Origin',(53.1295753616236,-3.2,80.));
#57104=CARTESIAN_POINT('',(53.1295753616236,-3.19999999999999,78.16));
#57105=CARTESIAN_POINT('Origin',(53.1295753616236,-3.19999999999999,78.16));
#57106=CARTESIAN_POINT('',(52.8895753616236,-3.19999999999999,78.16));
#57107=CARTESIAN_POINT('Origin',(52.8895753616236,-3.19999999999999,78.16));
#57108=CARTESIAN_POINT('',(52.8895753616236,-3.19999999999999,78.4));
#57109=CARTESIAN_POINT('Origin',(-67.1104246383764,-3.19999999999999,78.4));
#57110=CARTESIAN_POINT('',(-67.1104246383764,-3.19999999999999,78.4));
#57111=CARTESIAN_POINT('',(-67.1104246383764,-3.19999999999999,78.16));
#57112=CARTESIAN_POINT('Origin',(-67.1104246383764,-3.19999999999999,78.16));
#57113=CARTESIAN_POINT('',(-67.3504246383764,-3.19999999999999,78.16));
#57114=CARTESIAN_POINT('Origin',(-67.3504246383764,-3.19999999999999,78.16));
#57115=CARTESIAN_POINT('Origin',(-67.1104246383764,-2.4,78.4));
#57116=CARTESIAN_POINT('',(-67.1104246383764,-2.4,80.));
#57117=CARTESIAN_POINT('Origin',(-67.1104246383764,-2.4,78.4));
#57118=CARTESIAN_POINT('Origin',(-67.1104246383764,-2.4,78.4));
#57119=CARTESIAN_POINT('Origin',(52.8895753616236,-2.4,78.4));
#57120=CARTESIAN_POINT('Origin',(52.8895753616236,-2.4,78.4));
#57121=CARTESIAN_POINT('',(52.8895753616236,-2.4,79.2));
#57122=CARTESIAN_POINT('Origin',(52.8895753616236,-2.4,78.4));
#57123=CARTESIAN_POINT('Origin',(52.8895753616236,-2.4,78.4));
#57124=CARTESIAN_POINT('Origin',(52.8895753616236,-2.4,78.4));
#57125=CARTESIAN_POINT('Origin',(52.8895753616236,2.80000000000001,80.));
#57126=CARTESIAN_POINT('',(52.8895753616236,2.80000000000001,80.));
#57127=CARTESIAN_POINT('Origin',(-67.1104246383764,-3.2,80.));
#57128=CARTESIAN_POINT('',(-67.1104246383764,2.79999999999996,80.));
#57129=CARTESIAN_POINT('Origin',(48.8895753616236,2.80000000000003,80.));
#57130=CARTESIAN_POINT('',(48.8895753616235,6.80000000000003,80.));
#57131=CARTESIAN_POINT('Origin',(-63.1104246383764,6.79999999999999,80.));
#57132=CARTESIAN_POINT('',(-63.1104246383764,6.79999999999999,80.));
#57133=CARTESIAN_POINT('Origin',(-63.1104246383764,2.79999999999999,80.));
#57134=CARTESIAN_POINT('Origin',(-52.1104246383764,3.80000000000003,79.9999999999841));
#57135=CARTESIAN_POINT('Origin',(-46.8391000074924,3.80000000000003,77.9999999999841));
#57136=CARTESIAN_POINT('Origin',(-57.3817492692605,3.80000000000003,77.9999999999841));
#57137=CARTESIAN_POINT('Origin',(-52.1104246383764,-0.199999999999972,79.9999999999841));
#57138=CARTESIAN_POINT('Origin',(-57.3817492692605,-0.199999999999971,77.9999999999841));
#57139=CARTESIAN_POINT('Origin',(-46.8391000074924,-0.199999999999971,77.9999999999841));
#57140=CARTESIAN_POINT('Origin',(-46.8391000074924,3.80000000000003,77.9999999999841));
#57141=CARTESIAN_POINT('',(-48.6500178794101,3.80000000000003,78.8488677524455));
#57142=CARTESIAN_POINT('Origin',(-46.8391000074924,3.80000000000003,77.9999999999841));
#57143=CARTESIAN_POINT('',(-48.6500178794101,-0.199999999999972,78.8488677524455));
#57144=CARTESIAN_POINT('',(-48.6500178794101,3.80000000000003,78.8488677524455));
#57145=CARTESIAN_POINT('Origin',(-46.8391000074924,-0.199999999999971,77.9999999999841));
#57146=CARTESIAN_POINT('Origin',(-57.3817492692605,1.80000000000003,77.9999999999841));
#57147=CARTESIAN_POINT('',(-55.5708313973427,-0.199999999999972,78.8488677524455));
#57148=CARTESIAN_POINT('Origin',(-57.3817492692605,-0.199999999999971,77.9999999999841));
#57149=CARTESIAN_POINT('',(-55.5708313973427,3.80000000000003,78.8488677524455));
#57150=CARTESIAN_POINT('',(-55.5708313973427,3.80000000000003,78.8488677524455));
#57151=CARTESIAN_POINT('Origin',(-57.3817492692605,3.80000000000003,77.9999999999841));
#57152=CARTESIAN_POINT('Origin',(-57.3817492692605,-0.199999999999971,77.9999999999841));
#57153=CARTESIAN_POINT('',(-56.2951985461098,-0.199999999999974,78.509320651461));
#57154=CARTESIAN_POINT('Origin',(-57.3817492692605,-0.19999999999997,77.9999999999841));
#57155=CARTESIAN_POINT('',(-55.7394867179188,-0.199999999999974,77.3238020846534));
#57156=CARTESIAN_POINT('',(-55.3347917871435,-0.199999999999974,76.4604528989995));
#57157=CARTESIAN_POINT('',(-53.6569311652134,-0.199999999999972,75.9999999999841));
#57158=CARTESIAN_POINT('Origin',(-53.6569311652134,-0.19999999999997,78.2999999999841));
#57159=CARTESIAN_POINT('',(-50.5639181115395,-0.19999999999997,75.9999999999841));
#57160=CARTESIAN_POINT('',(-49.6104246383764,-0.199999999999972,75.9999999999841));
#57161=CARTESIAN_POINT('',(-48.4813625588341,-0.199999999999974,77.3238020846534));
#57162=CARTESIAN_POINT('Origin',(-50.5639181115395,-0.19999999999997,78.2999999999841));
#57163=CARTESIAN_POINT('',(-47.925650730643,-0.19999999999997,78.509320651461));
#57164=CARTESIAN_POINT('',(-48.8860574896093,-0.199999999999974,76.4604528989995));
#57165=CARTESIAN_POINT('Origin',(-46.8391000074924,-0.19999999999997,77.9999999999841));
#57166=CARTESIAN_POINT('',(-49.2057297076012,-0.199999999999972,77.663349185638));
#57167=CARTESIAN_POINT('',(-49.6104246383764,-0.199999999999972,76.7999999999841));
#57168=CARTESIAN_POINT('',(-50.5639181115395,-0.199999999999972,76.7999999999841));
#57169=CARTESIAN_POINT('Origin',(-50.5639181115395,-0.199999999999971,78.2999999999841));
#57170=CARTESIAN_POINT('',(-53.6569311652134,-0.199999999999972,76.7999999999841));
#57171=CARTESIAN_POINT('',(-49.6104246383764,-0.199999999999972,76.7999999999841));
#57172=CARTESIAN_POINT('',(-55.0151195691517,-0.199999999999972,77.663349185638));
#57173=CARTESIAN_POINT('Origin',(-53.6569311652134,-0.199999999999971,78.2999999999841));
#57174=CARTESIAN_POINT('',(-54.6104246383764,-0.199999999999972,76.7999999999841));
#57175=CARTESIAN_POINT('Origin',(-49.6104246383764,3.80000000000003,76.7999999999841));
#57176=CARTESIAN_POINT('',(-47.925650730643,3.80000000000003,78.509320651461));
#57177=CARTESIAN_POINT('Origin',(-46.8391000074924,3.80000000000003,77.9999999999841));
#57178=CARTESIAN_POINT('',(-48.4813625588341,3.80000000000003,77.3238020846534));
#57179=CARTESIAN_POINT('',(-48.8860574896093,3.80000000000003,76.4604528989995));
#57180=CARTESIAN_POINT('',(-50.5639181115395,3.80000000000003,75.9999999999841));
#57181=CARTESIAN_POINT('Origin',(-50.5639181115395,3.80000000000003,78.2999999999841));
#57182=CARTESIAN_POINT('',(-53.6569311652134,3.80000000000003,75.9999999999841));
#57183=CARTESIAN_POINT('',(-49.6104246383764,3.80000000000003,75.9999999999841));
#57184=CARTESIAN_POINT('',(-55.7394867179188,3.80000000000003,77.3238020846534));
#57185=CARTESIAN_POINT('Origin',(-53.6569311652134,3.80000000000003,78.2999999999841));
#57186=CARTESIAN_POINT('',(-56.2951985461098,3.80000000000003,78.509320651461));
#57187=CARTESIAN_POINT('',(-55.3347917871435,3.80000000000003,76.4604528989995));
#57188=CARTESIAN_POINT('Origin',(-57.3817492692605,3.80000000000003,77.9999999999841));
#57189=CARTESIAN_POINT('',(-55.0151195691517,3.80000000000003,77.663349185638));
#57190=CARTESIAN_POINT('',(-54.6104246383764,3.80000000000003,76.7999999999841));
#57191=CARTESIAN_POINT('',(-53.6569311652134,3.80000000000003,76.7999999999841));
#57192=CARTESIAN_POINT('Origin',(-53.6569311652134,3.80000000000003,78.2999999999841));
#57193=CARTESIAN_POINT('',(-50.5639181115395,3.80000000000003,76.7999999999841));
#57194=CARTESIAN_POINT('',(-49.6104246383764,3.80000000000003,76.7999999999841));
#57195=CARTESIAN_POINT('',(-49.2057297076012,3.80000000000003,77.663349185638));
#57196=CARTESIAN_POINT('Origin',(-50.5639181115395,3.80000000000003,78.2999999999841));
#57197=CARTESIAN_POINT('',(-49.6104246383764,3.80000000000003,76.7999999999841));
#57198=CARTESIAN_POINT('Origin',(-50.5639181115395,3.80000000000003,78.2999999999841));
#57199=CARTESIAN_POINT('',(-50.5639181115395,3.80000000000003,76.7999999999841));
#57200=CARTESIAN_POINT('',(-49.2057297076012,3.80000000000003,77.663349185638));
#57201=CARTESIAN_POINT('Origin',(-53.6569311652134,3.80000000000003,78.2999999999841));
#57202=CARTESIAN_POINT('',(-55.0151195691517,3.80000000000003,77.663349185638));
#57203=CARTESIAN_POINT('',(-53.6569311652134,3.80000000000003,76.7999999999841));
#57204=CARTESIAN_POINT('Origin',(-49.6104246383764,3.80000000000003,76.7999999999841));
#57205=CARTESIAN_POINT('Origin',(-54.6104246383764,3.80000000000003,76.7999999999841));
#57206=CARTESIAN_POINT('Origin',(-49.6104246383764,3.80000000000003,76.7999999999841));
#57207=CARTESIAN_POINT('Origin',(-50.5639181115395,3.80000000000003,78.2999999999841));
#57208=CARTESIAN_POINT('',(-48.4813625588341,3.80000000000003,77.3238020846534));
#57209=CARTESIAN_POINT('',(-50.5639181115395,3.80000000000003,75.9999999999841));
#57210=CARTESIAN_POINT('Origin',(-53.6569311652134,3.80000000000003,78.2999999999841));
#57211=CARTESIAN_POINT('',(-53.6569311652134,3.80000000000003,75.9999999999841));
#57212=CARTESIAN_POINT('',(-55.7394867179188,3.80000000000003,77.3238020846534));
#57213=CARTESIAN_POINT('Origin',(-57.3817492692605,1.80000000000003,77.9999999999841));
#57214=CARTESIAN_POINT('',(-56.2951985461098,3.80000000000003,78.509320651461));
#57215=CARTESIAN_POINT('Origin',(-46.8391000074924,3.80000000000003,77.9999999999841));
#57216=CARTESIAN_POINT('',(-47.925650730643,3.80000000000003,78.509320651461));
#57217=CARTESIAN_POINT('Origin',(-48.8860574896093,3.80000000000003,76.4604528989995));
#57218=CARTESIAN_POINT('Origin',(-55.3347917871435,3.80000000000003,76.4604528989995));
#57219=CARTESIAN_POINT('Origin',(-49.6104246383764,3.80000000000003,75.9999999999841));
#57220=CARTESIAN_POINT('Origin',(38.3304246383764,3.80000000000005,79.9999999999841));
#57221=CARTESIAN_POINT('Origin',(43.6017492692605,3.80000000000006,77.9999999999841));
#57222=CARTESIAN_POINT('Origin',(33.0591000074924,3.80000000000005,77.9999999999841));
#57223=CARTESIAN_POINT('Origin',(38.3304246383764,-0.199999999999946,79.9999999999841));
#57224=CARTESIAN_POINT('Origin',(33.0591000074924,-0.199999999999948,77.9999999999841));
#57225=CARTESIAN_POINT('Origin',(43.6017492692605,-0.199999999999942,77.9999999999841));
#57226=CARTESIAN_POINT('Origin',(33.0591000074924,3.80000000000005,77.9999999999841));
#57227=CARTESIAN_POINT('',(34.8700178794101,-0.199999999999948,78.8488677524455));
#57228=CARTESIAN_POINT('Origin',(33.0591000074924,-0.199999999999948,77.9999999999841));
#57229=CARTESIAN_POINT('',(34.8700178794101,3.80000000000005,78.8488677524455));
#57230=CARTESIAN_POINT('',(34.8700178794101,3.80000000000005,78.8488677524455));
#57231=CARTESIAN_POINT('Origin',(33.0591000074924,3.80000000000005,77.9999999999841));
#57232=CARTESIAN_POINT('Origin',(43.6017492692605,1.80000000000006,77.9999999999841));
#57233=CARTESIAN_POINT('',(41.7908313973427,3.80000000000006,78.8488677524455));
#57234=CARTESIAN_POINT('Origin',(43.6017492692605,3.80000000000006,77.9999999999841));
#57235=CARTESIAN_POINT('',(41.7908313973428,-0.199999999999944,78.8488677524455));
#57236=CARTESIAN_POINT('',(41.7908313973427,3.80000000000006,78.8488677524455));
#57237=CARTESIAN_POINT('Origin',(43.6017492692605,-0.199999999999942,77.9999999999841));
#57238=CARTESIAN_POINT('Origin',(33.0591000074924,-0.199999999999948,77.9999999999841));
#57239=CARTESIAN_POINT('',(34.1456507306431,-0.199999999999949,78.509320651461));
#57240=CARTESIAN_POINT('Origin',(33.0591000074924,-0.199999999999947,77.9999999999841));
#57241=CARTESIAN_POINT('',(34.7013625588341,-0.199999999999946,77.3238020846534));
#57242=CARTESIAN_POINT('',(35.1060574896094,-0.19999999999995,76.4604528989995));
#57243=CARTESIAN_POINT('',(36.7839181115395,-0.199999999999947,75.9999999999841));
#57244=CARTESIAN_POINT('Origin',(36.7839181115395,-0.199999999999945,78.2999999999841));
#57245=CARTESIAN_POINT('',(39.8769311652134,-0.199999999999943,75.9999999999841));
#57246=CARTESIAN_POINT('',(35.8304246383764,-0.199999999999948,75.9999999999841));
#57247=CARTESIAN_POINT('',(41.9594867179188,-0.199999999999945,77.3238020846534));
#57248=CARTESIAN_POINT('Origin',(39.8769311652134,-0.199999999999943,78.2999999999841));
#57249=CARTESIAN_POINT('',(42.5151985461099,-0.199999999999945,78.509320651461));
#57250=CARTESIAN_POINT('',(41.5547917871435,-0.199999999999945,76.4604528989995));
#57251=CARTESIAN_POINT('Origin',(43.6017492692605,-0.199999999999941,77.9999999999841));
#57252=CARTESIAN_POINT('',(41.2351195691517,-0.199999999999944,77.663349185638));
#57253=CARTESIAN_POINT('',(40.8304246383765,-0.199999999999944,76.7999999999841));
#57254=CARTESIAN_POINT('',(39.8769311652134,-0.199999999999945,76.7999999999841));
#57255=CARTESIAN_POINT('Origin',(39.8769311652134,-0.199999999999944,78.2999999999841));
#57256=CARTESIAN_POINT('',(36.7839181115395,-0.199999999999947,76.7999999999841));
#57257=CARTESIAN_POINT('',(35.8304246383764,-0.199999999999947,76.7999999999841));
#57258=CARTESIAN_POINT('',(35.4257297076012,-0.199999999999947,77.663349185638));
#57259=CARTESIAN_POINT('Origin',(36.7839181115395,-0.199999999999946,78.2999999999841));
#57260=CARTESIAN_POINT('',(35.8304246383764,-0.199999999999947,76.7999999999841));
#57261=CARTESIAN_POINT('Origin',(35.8304246383764,3.80000000000005,76.7999999999841));
#57262=CARTESIAN_POINT('',(42.5151985461099,3.80000000000006,78.509320651461));
#57263=CARTESIAN_POINT('Origin',(43.6017492692605,3.80000000000006,77.9999999999841));
#57264=CARTESIAN_POINT('',(41.9594867179188,3.80000000000006,77.3238020846534));
#57265=CARTESIAN_POINT('',(41.5547917871435,3.80000000000006,76.4604528989995));
#57266=CARTESIAN_POINT('',(39.8769311652134,3.80000000000005,75.9999999999841));
#57267=CARTESIAN_POINT('Origin',(39.8769311652134,3.80000000000005,78.2999999999841));
#57268=CARTESIAN_POINT('',(36.7839181115395,3.80000000000005,75.9999999999841));
#57269=CARTESIAN_POINT('',(35.8304246383764,3.80000000000005,75.9999999999841));
#57270=CARTESIAN_POINT('',(34.7013625588341,3.80000000000005,77.3238020846534));
#57271=CARTESIAN_POINT('Origin',(36.7839181115395,3.80000000000005,78.2999999999841));
#57272=CARTESIAN_POINT('',(34.1456507306431,3.80000000000005,78.509320651461));
#57273=CARTESIAN_POINT('',(35.1060574896094,3.80000000000005,76.4604528989995));
#57274=CARTESIAN_POINT('Origin',(33.0591000074924,3.80000000000005,77.9999999999841));
#57275=CARTESIAN_POINT('',(35.4257297076012,3.80000000000005,77.663349185638));
#57276=CARTESIAN_POINT('',(35.8304246383764,3.80000000000005,76.7999999999841));
#57277=CARTESIAN_POINT('',(36.7839181115395,3.80000000000005,76.7999999999841));
#57278=CARTESIAN_POINT('Origin',(36.7839181115395,3.80000000000005,78.2999999999841));
#57279=CARTESIAN_POINT('',(39.8769311652134,3.80000000000005,76.7999999999841));
#57280=CARTESIAN_POINT('',(35.8304246383764,3.80000000000005,76.7999999999841));
#57281=CARTESIAN_POINT('',(41.2351195691517,3.80000000000006,77.663349185638));
#57282=CARTESIAN_POINT('Origin',(39.8769311652134,3.80000000000005,78.2999999999841));
#57283=CARTESIAN_POINT('',(40.8304246383765,3.80000000000006,76.7999999999841));
#57284=CARTESIAN_POINT('Origin',(36.7839181115395,3.80000000000005,78.2999999999841));
#57285=CARTESIAN_POINT('',(35.4257297076012,3.80000000000005,77.663349185638));
#57286=CARTESIAN_POINT('',(36.7839181115395,3.80000000000005,76.7999999999841));
#57287=CARTESIAN_POINT('Origin',(39.8769311652134,3.80000000000005,78.2999999999841));
#57288=CARTESIAN_POINT('',(39.8769311652134,3.80000000000005,76.7999999999841));
#57289=CARTESIAN_POINT('',(41.2351195691517,3.80000000000006,77.663349185638));
#57290=CARTESIAN_POINT('Origin',(35.8304246383764,3.80000000000005,76.7999999999841));
#57291=CARTESIAN_POINT('Origin',(40.8304246383765,3.80000000000006,76.7999999999841));
#57292=CARTESIAN_POINT('Origin',(35.8304246383764,3.80000000000005,76.7999999999841));
#57293=CARTESIAN_POINT('Origin',(36.7839181115395,3.80000000000005,78.2999999999841));
#57294=CARTESIAN_POINT('',(36.7839181115395,3.80000000000005,75.9999999999841));
#57295=CARTESIAN_POINT('',(34.7013625588341,3.80000000000005,77.3238020846534));
#57296=CARTESIAN_POINT('Origin',(39.8769311652134,3.80000000000005,78.2999999999841));
#57297=CARTESIAN_POINT('',(41.9594867179188,3.80000000000006,77.3238020846534));
#57298=CARTESIAN_POINT('',(39.8769311652134,3.80000000000005,75.9999999999841));
#57299=CARTESIAN_POINT('Origin',(43.6017492692605,1.80000000000006,77.9999999999841));
#57300=CARTESIAN_POINT('',(42.5151985461099,1.80000000000006,78.509320651461));
#57301=CARTESIAN_POINT('Origin',(33.0591000074924,3.80000000000005,77.9999999999841));
#57302=CARTESIAN_POINT('',(34.1456507306431,3.80000000000005,78.509320651461));
#57303=CARTESIAN_POINT('Origin',(35.1060574896094,3.80000000000005,76.4604528989995));
#57304=CARTESIAN_POINT('Origin',(41.5547917871435,3.80000000000006,76.4604528989995));
#57305=CARTESIAN_POINT('Origin',(35.8304246383764,3.80000000000005,75.9999999999841));
#57306=CARTESIAN_POINT('Origin',(-67.3504246383764,-3.20000000000001,-80.));
#57307=CARTESIAN_POINT('',(-67.3504246383764,-3.20000000000001,-78.16));
#57308=CARTESIAN_POINT('Origin',(-67.3504246383764,-3.20000000000001,-78.16));
#57309=CARTESIAN_POINT('',(-67.1104246383764,-3.20000000000001,-78.16));
#57310=CARTESIAN_POINT('Origin',(-67.1104246383764,-3.20000000000001,-78.16));
#57311=CARTESIAN_POINT('',(-67.1104246383764,-3.20000000000001,-78.4));
#57312=CARTESIAN_POINT('Origin',(52.8895753616236,-3.20000000000001,-78.4));
#57313=CARTESIAN_POINT('',(52.8895753616236,-3.20000000000001,-78.4));
#57314=CARTESIAN_POINT('',(52.8895753616236,-3.20000000000001,-78.16));
#57315=CARTESIAN_POINT('Origin',(52.8895753616236,-3.20000000000001,-78.16));
#57316=CARTESIAN_POINT('',(53.1295753616236,-3.20000000000001,-78.16));
#57317=CARTESIAN_POINT('Origin',(53.1295753616236,-3.20000000000001,-78.16));
#57318=CARTESIAN_POINT('Origin',(52.8895753616236,-2.40000000000002,-78.4));
#57319=CARTESIAN_POINT('',(52.8895753616236,-2.40000000000002,-79.2));
#57320=CARTESIAN_POINT('',(52.8895753616236,-2.40000000000002,-80.));
#57321=CARTESIAN_POINT('',(52.8895753616236,-2.40000000000001,-80.0000000000001));
#57322=CARTESIAN_POINT('Origin',(52.8895753616236,-2.40000000000002,-78.4));
#57323=CARTESIAN_POINT('Origin',(52.8895753616236,-2.40000000000002,-78.4));
#57324=CARTESIAN_POINT('Origin',(-67.1104246383764,-2.40000000000002,-78.4));
#57325=CARTESIAN_POINT('',(-67.1104246383764,-2.40000000000002,-79.2));
#57326=CARTESIAN_POINT('Origin',(-67.1104246383764,-2.40000000000002,-78.4));
#57327=CARTESIAN_POINT('',(-67.1104246383764,-2.40000000000001,-80.));
#57328=CARTESIAN_POINT('',(-67.1104246383764,-2.40000000000001,-79.2));
#57329=CARTESIAN_POINT('Origin',(-67.1104246383764,-2.40000000000002,-78.4));
#57330=CARTESIAN_POINT('Origin',(-67.1104246383764,-2.40000000000002,-78.4));
#57331=CARTESIAN_POINT('',(52.8895753616236,-2.40000000000001,-80.));
#57332=CARTESIAN_POINT('Origin',(-67.1104246383764,-2.40000000000002,-78.4));
#57333=CARTESIAN_POINT('',(52.8895753616236,-2.40000000000001,-79.2));
#57334=CARTESIAN_POINT('Origin',(52.8895753616236,2.80000000000001,-80.));
#57335=CARTESIAN_POINT('',(52.8895753616236,2.80000000000002,-79.2));
#57336=CARTESIAN_POINT('',(52.8895753616236,2.80000000000012,-79.2));
#57337=CARTESIAN_POINT('',(52.8895753616236,2.80000000000002,-80.));
#57338=CARTESIAN_POINT('',(52.8895753616236,2.80000000000001,-80.));
#57339=CARTESIAN_POINT('',(52.8895753616236,2.80000000000001,-80.));
#57340=CARTESIAN_POINT('Origin',(-67.1104246383764,-3.2,-80.));
#57341=CARTESIAN_POINT('',(-67.1104246383764,2.79999999999997,-80.));
#57342=CARTESIAN_POINT('',(-67.1104246383764,-3.2,-80.));
#57343=CARTESIAN_POINT('',(-67.1104246383764,2.79999999999997,-79.2));
#57344=CARTESIAN_POINT('',(-67.1104246383764,2.79999999999999,-79.2));
#57345=CARTESIAN_POINT('',(-67.1104246383764,2.79999999999996,-80.));
#57346=CARTESIAN_POINT('Origin',(-63.1104246383764,2.79999999999999,-80.));
#57347=CARTESIAN_POINT('',(-63.1104246383764,6.79999999999999,-80.));
#57348=CARTESIAN_POINT('Origin',(-63.1104246383764,2.79999999999999,-80.));
#57349=CARTESIAN_POINT('',(48.8895753616235,6.80000000000003,-80.));
#57350=CARTESIAN_POINT('',(-63.1104246383764,6.79999999999999,-80.));
#57351=CARTESIAN_POINT('Origin',(48.8895753616236,2.80000000000003,-80.));
#57352=CARTESIAN_POINT('Origin',(-63.1104246383764,2.79999999999999,-79.2));
#57353=CARTESIAN_POINT('',(48.8895753616235,6.80000000000003,-79.2));
#57354=CARTESIAN_POINT('Origin',(48.8895753616236,2.80000000000003,-79.2));
#57355=CARTESIAN_POINT('',(-63.1104246383764,6.79999999999999,-79.2));
#57356=CARTESIAN_POINT('',(-63.1104246383764,6.79999999999999,-79.2));
#57357=CARTESIAN_POINT('Origin',(-63.1104246383764,2.79999999999999,-79.2));
#57358=CARTESIAN_POINT('Origin',(-63.1104246383764,2.79999999999999,-80.));
#57359=CARTESIAN_POINT('',(-63.1104246383764,6.79999999999999,-80.));
#57360=CARTESIAN_POINT('Origin',(-63.1104246383764,6.79999999999999,-80.));
#57361=CARTESIAN_POINT('',(48.8895753616235,6.80000000000003,-80.));
#57362=CARTESIAN_POINT('Origin',(48.8895753616236,2.80000000000003,-80.));
#65294=UNCERTAINTY_MEASURE_WITH_UNIT(LENGTH_MEASURE(0.01),#65305,
'DISTANCE_ACCURACY_VALUE',
'Maximum model space distance between geometric entities at asserted c
onnectivities');
#65298=UNCERTAINTY_MEASURE_WITH_UNIT(LENGTH_MEASURE(0.01),#65305,
'DISTANCE_ACCURACY_VALUE',
'Maximum model space distance between geometric entities at asserted c
onnectivities');
#65300=(
GEOMETRIC_REPRESENTATION_CONTEXT(3)
GLOBAL_UNCERTAINTY_ASSIGNED_CONTEXT((#65294))
GLOBAL_UNIT_ASSIGNED_CONTEXT((#65305,#65307,#65308))
REPRESENTATION_CONTEXT('','3D')
);
#65304=(
GEOMETRIC_REPRESENTATION_CONTEXT(3)
GLOBAL_UNCERTAINTY_ASSIGNED_CONTEXT((#65298))
GLOBAL_UNIT_ASSIGNED_CONTEXT((#65305,#65307,#65308))
REPRESENTATION_CONTEXT('','3D')
);
#65305=(
LENGTH_UNIT()
NAMED_UNIT(*)
SI_UNIT(.MILLI.,.METRE.)
);
#65307=(
NAMED_UNIT(*)
PLANE_ANGLE_UNIT()
SI_UNIT($,.RADIAN.)
);
#65308=(
NAMED_UNIT(*)
SI_UNIT($,.STERADIAN.)
SOLID_ANGLE_UNIT()
);
#65310=SHAPE_DEFINITION_REPRESENTATION(#65315,#65324);
#65315=PRODUCT_DEFINITION_SHAPE('',$,#65330);
#65324=SHAPE_REPRESENTATION('',(#39984),#65300);
#65328=PRODUCT_DEFINITION_CONTEXT('part definition',#65345,'design');
#65330=PRODUCT_DEFINITION('Sheet Metal Down','Sheet Metal Down',#65335,
#65328);
#65335=PRODUCT_DEFINITION_FORMATION('',$,#65348);
#65345=APPLICATION_CONTEXT(
'Core Data for Automotive Mechanical Design Process');
#65346=PRODUCT_CONTEXT('part definition',#65345,'mechanical');
#65348=PRODUCT('Sheet Metal Down','Sheet Metal Down',$,(#65346));
#65353=PRESENTATION_STYLE_ASSIGNMENT((#65358));
#65358=SURFACE_STYLE_USAGE(.BOTH.,#65363);
#65363=SURFACE_SIDE_STYLE('',(#65368));
#65368=SURFACE_STYLE_FILL_AREA(#65373);
#65373=FILL_AREA_STYLE('Opaque(104,114,127)',(#65378));
#65378=FILL_AREA_STYLE_COLOUR('Opaque(104,114,127)',#65383);
#65383=COLOUR_RGB('Opaque(104,114,127)',0.407843137254902,0.447058823529412,
0.498039215686275);
ENDSEC;
END-ISO-10303-21;
